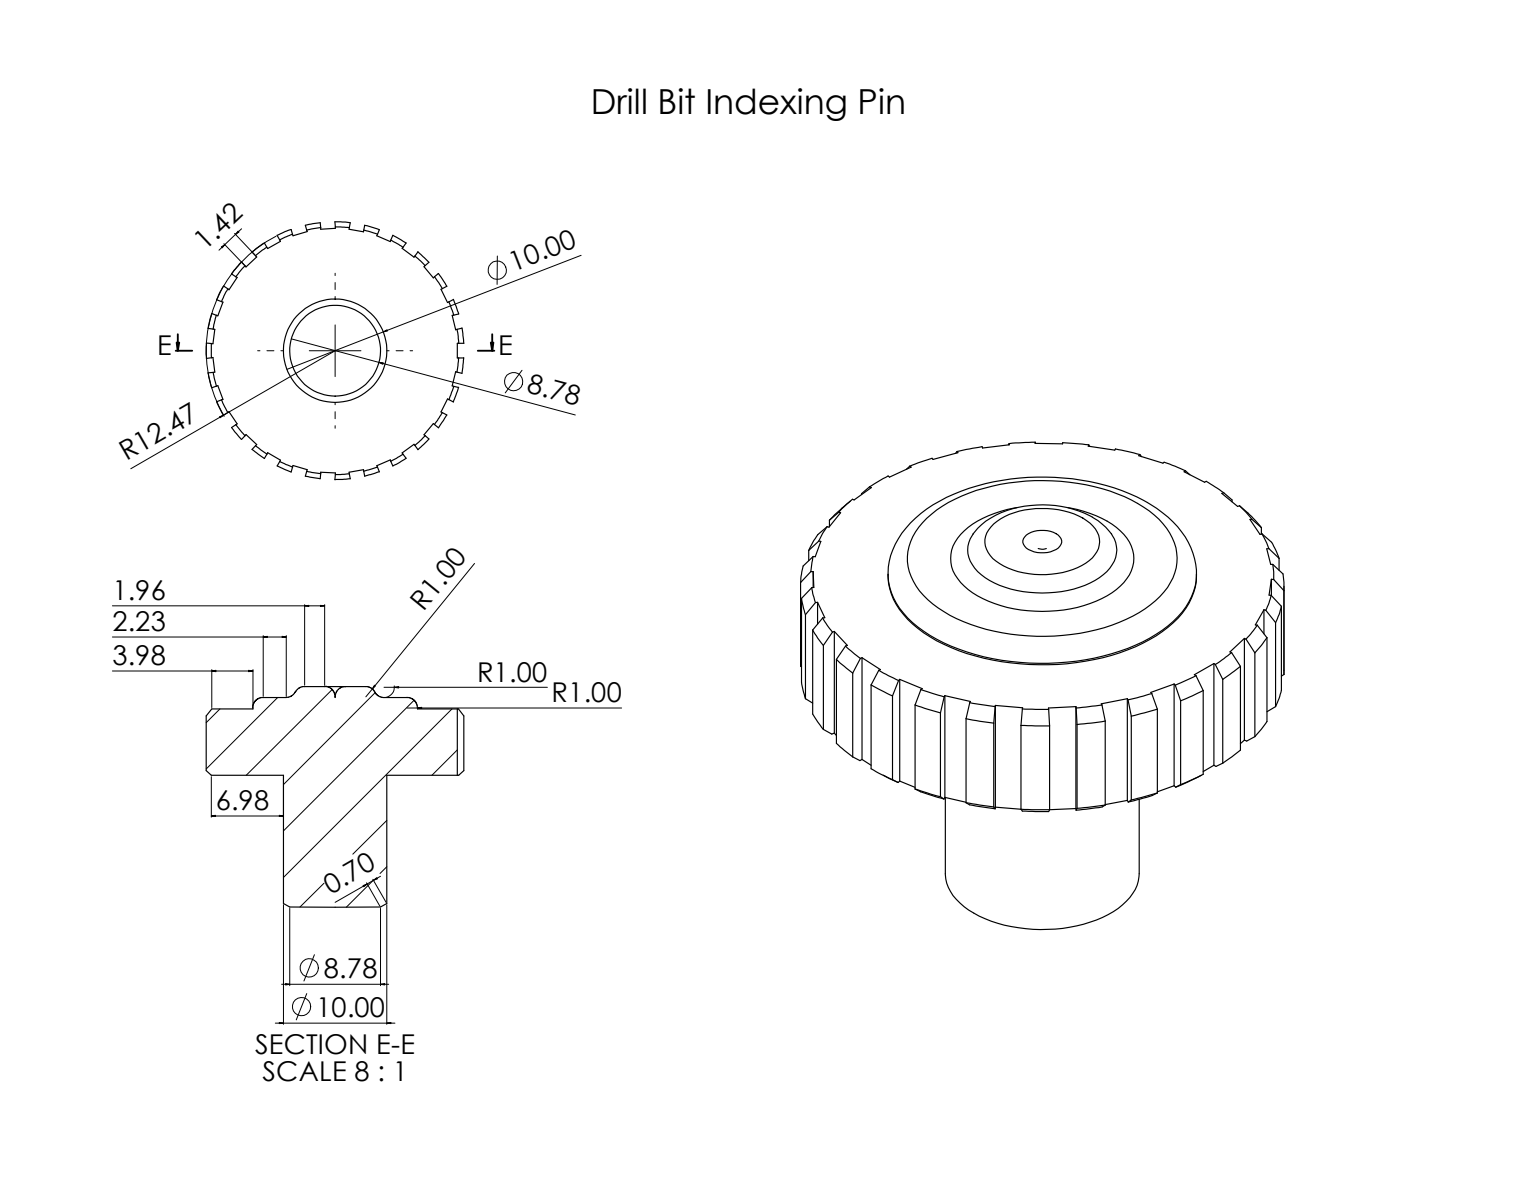
ISO-10303-21;
HEADER;
FILE_DESCRIPTION (('STEP AP214'),
    '1' );
FILE_NAME ('Drill Bit Indexing Pin.step',
    '2026-10-26T22:46:44',
    ( '' ),
    ( '' ),
    'SwSTEP 2.0',
    'SolidWorks 2025',
    '' );
FILE_SCHEMA (( 'AUTOMOTIVE_DESIGN' ));
ENDSEC;

DATA;
#1=PLANE ( 'NONE',  #9182 ) ;
#14=ORIENTED_EDGE ( 'NONE', *, *, #6610, .T. ) ;
#16=DIRECTION ( 'NONE',  ( -0.8660254037844355990, -0.5000000000000055511, 0.000000000000000000 ) ) ;
#17=ORIENTED_EDGE ( 'NONE', *, *, #2123, .F. ) ;
#21=LINE ( 'NONE', #16230, #18993 ) ;
#23=FACE_OUTER_BOUND ( 'NONE', #2829, .T. ) ;
#24=CARTESIAN_POINT ( 'NONE',  ( 211.0853526979653907, 12.80985690719961312, -24.65893733905802776 ) ) ;
#25=AXIS2_PLACEMENT_3D ( 'NONE', #18547, #841, #7289 ) ;
#31=DIRECTION ( 'NONE',  ( -0.2483788854153071712, -0.1434016163555487389, -0.9579895123154875680 ) ) ;
#32=VECTOR ( 'NONE', #7463, 1000.000000000000114 ) ;
#34=LINE ( 'NONE', #11272, #10471 ) ;
#35=CARTESIAN_POINT ( 'NONE',  ( 214.5488276859554162, 7.740514238813806180, -25.36561010639692881 ) ) ;
#39=EDGE_CURVE ( 'NONE', #7899, #11760, #18628, .T. ) ;
#43=B_SPLINE_CURVE_WITH_KNOTS ( 'NONE', 3,
 ( #9463, #2715, #6285, #20719 ),
 .UNSPECIFIED., .F., .F.,
 ( 4, 4 ),
 ( 9.419794497943025677E-05, 0.0009481836829574997018 ),
 .UNSPECIFIED. ) ;
#46=VECTOR ( 'NONE', #10219, 1000.000000000000227 ) ;
#52=LINE ( 'NONE', #20812, #10386 ) ;
#60=ORIENTED_EDGE ( 'NONE', *, *, #4152, .T. ) ;
#63=CARTESIAN_POINT ( 'NONE',  ( 213.9541640218532166, 4.979392293579961937, -14.00000000000005507 ) ) ;
#68=CARTESIAN_POINT ( 'NONE',  ( 204.1847125716027733, 2.529609678273321727, -2.551678190571418092 ) ) ;
#70=CARTESIAN_POINT ( 'NONE',  ( 192.7136026671465174, 6.680946580180795458, -11.01983352639493141 ) ) ;
#77=CARTESIAN_POINT ( 'NONE',  ( 199.2231352798573027, 21.03391272677540513, -14.00000000000005507 ) ) ;
#83=CARTESIAN_POINT ( 'NONE',  ( 215.3534639294407782, 15.62807865697965504, -9.913166705713923221 ) ) ;
#86=ORIENTED_EDGE ( 'NONE', *, *, #18700, .F. ) ;
#89=CARTESIAN_POINT ( 'NONE',  ( 204.5373383384513772, 2.217977392850209561, -25.12838443884007944 ) ) ;
#96=DIRECTION ( 'NONE',  ( 0.7500000000000014433, 0.4330127018922259596, 0.4999999999999919509 ) ) ;
#103=CIRCLE ( 'NONE', #7142, 11.94520687646042667 ) ;
#106=CARTESIAN_POINT ( 'NONE',  ( 199.3420759002524960, 10.50789738563077513, -26.10173121575770239 ) ) ;
#108=CARTESIAN_POINT ( 'NONE',  ( 209.9458835816058411, 16.63000860489531263, -23.47937149798938350 ) ) ;
#109=ADVANCED_FACE ( 'NONE', ( #2310 ), #10446, .F. ) ;
#110=FACE_OUTER_BOUND ( 'NONE', #8894, .T. ) ;
#112=VERTEX_POINT ( 'NONE', #8556 ) ;
#118=EDGE_CURVE ( 'NONE', #7633, #8779, #11849, .T. ) ;
#119=ORIENTED_EDGE ( 'NONE', *, *, #8707, .T. ) ;
#128=DIRECTION ( 'NONE',  ( 0.5000000000000054401, -0.8660254037844354880, 0.000000000000000000 ) ) ;
#131=ORIENTED_EDGE ( 'NONE', *, *, #17184, .F. ) ;
#145=CYLINDRICAL_SURFACE ( 'NONE', #15851, 12.47473710546057646 ) ;
#148=AXIS2_PLACEMENT_3D ( 'NONE', #15807, #6608, #5027 ) ;
#155=ORIENTED_EDGE ( 'NONE', *, *, #17412, .T. ) ;
#157=EDGE_LOOP ( 'NONE', ( #6682, #1571, #19730, #8704 ) ) ;
#159=DIRECTION ( 'NONE',  ( 0.5000000000000054401, -0.8660254037844353769, 3.330669073875469128E-16 ) ) ;
#160=LINE ( 'NONE', #8201, #12763 ) ;
#161=AXIS2_PLACEMENT_3D ( 'NONE', #9354, #1324, #10848 ) ;
#163=CARTESIAN_POINT ( 'NONE',  ( 204.3649803021097568, 2.376073449241438595, -2.709673684914560621 ) ) ;
#171=EDGE_CURVE ( 'NONE', #6173, #11821, #2564, .T. ) ;
#177=VECTOR ( 'NONE', #19876, 1000.000000000000114 ) ;
#178=ORIENTED_EDGE ( 'NONE', *, *, #4682, .F. ) ;
#184=VERTEX_POINT ( 'NONE', #12380 ) ;
#185=ORIENTED_EDGE ( 'NONE', *, *, #2629, .T. ) ;
#186=EDGE_CURVE ( 'NONE', #5696, #10545, #15103, .T. ) ;
#192=ORIENTED_EDGE ( 'NONE', *, *, #8358, .F. ) ;
#194=VECTOR ( 'NONE', #13444, 1000.000000000000000 ) ;
#202=CARTESIAN_POINT ( 'NONE',  ( 206.2111997916997552, 10.34978999605213978, -2.036337243043280676 ) ) ;
#210=EDGE_CURVE ( 'NONE', #4589, #15417, #7306, .T. ) ;
#211=VECTOR ( 'NONE', #12529, 1000.000000000000114 ) ;
#212=CARTESIAN_POINT ( 'NONE',  ( 206.9147384664715048, 10.75597823931694563, -16.91825718831810477 ) ) ;
#224=CIRCLE ( 'NONE', #4614, 1.000000000000000888 ) ;
#230=DIRECTION ( 'NONE',  ( -0.5000000000000049960, 0.8660254037844358210, -0.000000000000000000 ) ) ;
#233=DIRECTION ( 'NONE',  ( -0.8660254037844354880, -0.5000000000000055511, 0.000000000000000000 ) ) ;
#234=ADVANCED_FACE ( 'NONE', ( #2627 ), #13079, .T. ) ;
#242=ORIENTED_EDGE ( 'NONE', *, *, #18363, .T. ) ;
#244=DIRECTION ( 'NONE',  ( -0.5000000000000049960, 0.8660254037844357100, -0.000000000000000000 ) ) ;
#248=CARTESIAN_POINT ( 'NONE',  ( 215.3457899893760725, 15.62364810561754958, -18.11117897393244647 ) ) ;
#251=LINE ( 'NONE', #16684, #18558 ) ;
#255=VERTEX_POINT ( 'NONE', #1143 ) ;
#257=ORIENTED_EDGE ( 'NONE', *, *, #4813, .T. ) ;
#258=CARTESIAN_POINT ( 'NONE',  ( 204.4631859798315361, 9.340573751222835952, -1.438440158918556255 ) ) ;
#260=CARTESIAN_POINT ( 'NONE',  ( 216.5552780741873278, 15.79089711517258188, -12.53629070788368338 ) ) ;
#266=ORIENTED_EDGE ( 'NONE', *, *, #16288, .F. ) ;
#267=VECTOR ( 'NONE', #19215, 1000.000000000000227 ) ;
#271=B_SPLINE_CURVE_WITH_KNOTS ( 'NONE', 3,
 ( #15574, #20319, #4421, #12593 ),
 .UNSPECIFIED., .F., .F.,
 ( 4, 4 ),
 ( 3.854193985297353114E-07, 0.0008543711573825201388 ),
 .UNSPECIFIED. ) ;
#275=LINE ( 'NONE', #15144, #3748 ) ;
#277=EDGE_CURVE ( 'NONE', #4589, #9756, #12406, .T. ) ;
#284=B_SPLINE_CURVE_WITH_KNOTS ( 'NONE', 3,
 ( #15872, #6200, #7896, #7588 ),
 .UNSPECIFIED., .F., .F.,
 ( 4, 4 ),
 ( 5.392423665328082974E-07, 0.0008545249803445767369 ),
 .UNSPECIFIED. ) ;
#286=ORIENTED_EDGE ( 'NONE', *, *, #8772, .T. ) ;
#291=CARTESIAN_POINT ( 'NONE',  ( 213.7304257015346423, 14.51400719500950132, -6.188753603160008332 ) ) ;
#295=EDGE_CURVE ( 'NONE', #10545, #10364, #20522, .T. ) ;
#296=DIRECTION ( 'NONE',  ( 0.5943026915289653100, 0.3431208189343725179, 0.7273736415730454041 ) ) ;
#303=CARTESIAN_POINT ( 'NONE',  ( 205.0644204223817439, 9.510686714291797017, -26.12768996730766347 ) ) ;
#306=ORIENTED_EDGE ( 'NONE', *, *, #3575, .F. ) ;
#307=EDGE_CURVE ( 'NONE', #6314, #7288, #8664, .T. ) ;
#310=VERTEX_POINT ( 'NONE', #12278 ) ;
#315=EDGE_CURVE ( 'NONE', #14969, #8807, #10929, .T. ) ;
#317=CARTESIAN_POINT ( 'NONE',  ( 207.3576251285122112, 11.01167897286662800, -2.341985411377013548 ) ) ;
#320=DIRECTION ( 'NONE',  ( -0.8660254037844355990, -0.5000000000000055511, 0.000000000000000000 ) ) ;
#321=ORIENTED_EDGE ( 'NONE', *, *, #9028, .T. ) ;
#323=CARTESIAN_POINT ( 'NONE',  ( 209.1177676012032407, 5.377710327540435209, -26.45271578590685380 ) ) ;
#325=AXIS2_PLACEMENT_3D ( 'NONE', #1147, #20520, #11965 ) ;
#328=DIRECTION ( 'NONE',  ( 0.9537419254229496657, 0.000000000000000000, 0.3006265784832155008 ) ) ;
#330=VERTEX_POINT ( 'NONE', #3444 ) ;
#335=ORIENTED_EDGE ( 'NONE', *, *, #7992, .F. ) ;
#340=VERTEX_POINT ( 'NONE', #1652 ) ;
#341=LINE ( 'NONE', #19828, #4394 ) ;
#343=EDGE_CURVE ( 'NONE', #18516, #1461, #6859, .T. ) ;
#344=ORIENTED_EDGE ( 'NONE', *, *, #7860, .F. ) ;
#346=VECTOR ( 'NONE', #15320, 1000.000000000000114 ) ;
#356=CARTESIAN_POINT ( 'NONE',  ( 205.5965122587965084, 9.994899983462953941, -14.00000000000005507 ) ) ;
#357=CARTESIAN_POINT ( 'NONE',  ( 218.1364845712607803, 10.58466899794828642, -8.415281845792092597 ) ) ;
#360=ADVANCED_FACE ( 'NONE', ( #16385 ), #15798, .T. ) ;
#367=AXIS2_PLACEMENT_3D ( 'NONE', #16920, #11953, #10334 ) ;
#370=LINE ( 'NONE', #11808, #12203 ) ;
#375=LINE ( 'NONE', #8408, #1415 ) ;
#377=AXIS2_PLACEMENT_3D ( 'NONE', #5841, #2472, #8925 ) ;
#380=DIRECTION ( 'NONE',  ( 0.3430151393149036276, 0.1980398830195791438, -0.9182161068802751069 ) ) ;
#384=FACE_OUTER_BOUND ( 'NONE', #1878, .T. ) ;
#389=DIRECTION ( 'NONE',  ( 0.8660254037844355990, 0.5000000000000054401, 0.000000000000000000 ) ) ;
#392=CARTESIAN_POINT ( 'NONE',  ( 205.8264633344831225, 9.596613037118636669, -14.00000000000005507 ) ) ;
#405=DIRECTION ( 'NONE',  ( 1.000000000000000000, 0.000000000000000000, 0.000000000000000000 ) ) ;
#413=CIRCLE ( 'NONE', #5471, 12.47473710546057823 ) ;
#415=VECTOR ( 'NONE', #6964, 1000.000000000000114 ) ;
#418=DIRECTION ( 'NONE',  ( 0.1005394128318083530, 0.05804645706261224447, -0.9932383577419438003 ) ) ;
#420=CARTESIAN_POINT ( 'NONE',  ( 199.2144802262915846, 21.04890371929339921, -14.00000000000005507 ) ) ;
#421=DIRECTION ( 'NONE',  ( -0.8660254037844355990, -0.5000000000000054401, 9.734124438199387596E-15 ) ) ;
#425=VERTEX_POINT ( 'NONE', #12897 ) ;
#430=VECTOR ( 'NONE', #14086, 1000.000000000000114 ) ;
#437=VERTEX_POINT ( 'NONE', #8202 ) ;
#438=CARTESIAN_POINT ( 'NONE',  ( 212.7108869958215109, 14.10238615300026410, -22.72623880687309139 ) ) ;
#440=DIRECTION ( 'NONE',  ( 0.9679941405060923376, 0.000000000000000000, 0.2509727952306220478 ) ) ;
#441=CARTESIAN_POINT ( 'NONE',  ( 200.5889925535338989, 11.22780505105986748, -1.381056684022586634 ) ) ;
#446=DIRECTION ( 'NONE',  ( 0.8426815769442687065, 0.4865224352899183979, 0.2306158707424263710 ) ) ;
#451=CARTESIAN_POINT ( 'NONE',  ( 218.7787453705537928, 10.18265835266665675, -11.24974199967301836 ) ) ;
#453=EDGE_LOOP ( 'NONE', ( #8064, #10260, #20838, #5288 ) ) ;
#455=EDGE_CURVE ( 'NONE', #2505, #184, #11818, .T. ) ;
#457=AXIS2_PLACEMENT_3D ( 'NONE', #2689, #2291, #9232 ) ;
#467=EDGE_CURVE ( 'NONE', #12472, #14490, #11407, .T. ) ;
#472=AXIS2_PLACEMENT_3D ( 'NONE', #20887, #6361, #6670 ) ;
#473=CARTESIAN_POINT ( 'NONE',  ( 203.1005406747554218, 12.67784803492986434, -27.13030671846408737 ) ) ;
#478=EDGE_CURVE ( 'NONE', #11306, #15921, #11716, .T. ) ;
#479=ORIENTED_EDGE ( 'NONE', *, *, #14298, .T. ) ;
#489=DIRECTION ( 'NONE',  ( 0.8660254037844352659, 0.5000000000000056621, 0.000000000000000000 ) ) ;
#508=ORIENTED_EDGE ( 'NONE', *, *, #8439, .F. ) ;
#514=DIRECTION ( 'NONE',  ( 0.5171545105027486322, 0.2985792958513951434, -0.8021231927550452889 ) ) ;
#515=CARTESIAN_POINT ( 'NONE',  ( 203.4466382902124622, 1.588261426394339981, -3.504773242918958420 ) ) ;
#518=CIRCLE ( 'NONE', #2552, 11.94520687646042667 ) ;
#531=ORIENTED_EDGE ( 'NONE', *, *, #18795, .T. ) ;
#534=DIRECTION ( 'NONE',  ( -0.5000000000000051070, 0.8660254037844359321, -0.000000000000000000 ) ) ;
#536=EDGE_CURVE ( 'NONE', #19458, #4355, #2580, .T. ) ;
#539=CARTESIAN_POINT ( 'NONE',  ( 212.9607779367323417, 18.37065867240589156, -8.669480444820855780 ) ) ;
#543=DIRECTION ( 'NONE',  ( -0.8404609622711977091, 0.000000000000000000, 0.5418720982835085742 ) ) ;
#550=CARTESIAN_POINT ( 'NONE',  ( 207.0013954503587286, 3.383002205901548098, -25.76107385416581508 ) ) ;
#552=B_SPLINE_CURVE_WITH_KNOTS ( 'NONE', 3,
 ( #19683, #19790, #16415, #17907 ),
 .UNSPECIFIED., .F., .F.,
 ( 4, 4 ),
 ( 5.256891072071942815E-05, 0.0007252197027765627845 ),
 .UNSPECIFIED. ) ;
#556=ORIENTED_EDGE ( 'NONE', *, *, #2526, .F. ) ;
#561=EDGE_CURVE ( 'NONE', #18877, #3166, #9046, .T. ) ;
#562=VECTOR ( 'NONE', #12012, 1000.000000000000000 ) ;
#567=DIRECTION ( 'NONE',  ( -0.8660254037844355990, -0.5000000000000054401, 9.734124438199387596E-15 ) ) ;
#568=FACE_OUTER_BOUND ( 'NONE', #8960, .T. ) ;
#574=CARTESIAN_POINT ( 'NONE',  ( 205.7612434495831621, 0.2492073957305620258, -14.00000000000005507 ) ) ;
#579=ORIENTED_EDGE ( 'NONE', *, *, #17154, .T. ) ;
#581=DIRECTION ( 'NONE',  ( -0.5000000000000051070, 0.8660254037844359321, -0.000000000000000000 ) ) ;
#582=CARTESIAN_POINT ( 'NONE',  ( 199.2144802262915846, 21.04890371929339921, -14.00000000000005507 ) ) ;
#589=EDGE_CURVE ( 'NONE', #17484, #14639, #4503, .T. ) ;
#590=FACE_OUTER_BOUND ( 'NONE', #6120, .T. ) ;
#593=ADVANCED_FACE ( 'NONE', ( #20489 ), #18839, .T. ) ;
#599=CARTESIAN_POINT ( 'NONE',  ( 209.9028093415542457, 12.48114176340366122, -13.84394651341481008 ) ) ;
#600=VERTEX_POINT ( 'NONE', #20184 ) ;
#605=ADVANCED_FACE ( 'NONE', ( #2494 ), #17328, .F. ) ;
#606=ORIENTED_EDGE ( 'NONE', *, *, #5768, .T. ) ;
#610=DIRECTION ( 'NONE',  ( 0.5000000000000049960, -0.8660254037844358210, 0.000000000000000000 ) ) ;
#613=VECTOR ( 'NONE', #5948, 1000.000000000000114 ) ;
#620=CARTESIAN_POINT ( 'NONE',  ( 200.2585560139914378, -0.5099779577875940273, -20.52105855319921801 ) ) ;
#622=CARTESIAN_POINT ( 'NONE',  ( 199.5722073119862046, -0.9062415656482646353, -8.625373497621064089 ) ) ;
#629=EDGE_CURVE ( 'NONE', #9080, #19592, #13093, .T. ) ;
#630=EDGE_LOOP ( 'NONE', ( #1633, #10180, #13625, #15445 ) ) ;
#633=DIRECTION ( 'NONE',  ( 0.8645602258681710506, 0.4991540791356393614, -0.05814482891047953461 ) ) ;
#635=ORIENTED_EDGE ( 'NONE', *, *, #10307, .F. ) ;
#637=ORIENTED_EDGE ( 'NONE', *, *, #186, .T. ) ;
#642=DIRECTION ( 'NONE',  ( -0.7951984747223626027, -0.4591080534401425495, -0.3960797660391542907 ) ) ;
#644=LINE ( 'NONE', #6991, #11943 ) ;
#648=DIRECTION ( 'NONE',  ( -0.8660254037844354880, -0.5000000000000055511, 0.000000000000000000 ) ) ;
#649=VECTOR ( 'NONE', #3501, 1000.000000000000227 ) ;
#650=ORIENTED_EDGE ( 'NONE', *, *, #14383, .T. ) ;
#652=EDGE_CURVE ( 'NONE', #15437, #9266, #15812, .T. ) ;
#654=CARTESIAN_POINT ( 'NONE',  ( 198.4658173668363190, 5.877991368080599521, -5.291540431471293715 ) ) ;
#667=FACE_OUTER_BOUND ( 'NONE', #13989, .T. ) ;
#668=AXIS2_PLACEMENT_3D ( 'NONE', #6471, #18619, #19618 ) ;
#671=EDGE_LOOP ( 'NONE', ( #12795, #14132, #9579, #15722 ) ) ;
#683=DIRECTION ( 'NONE',  ( -0.8660254037844360431, -0.5000000000000046629, 0.000000000000000000 ) ) ;
#684=DIRECTION ( 'NONE',  ( -0.5000000000000049960, 0.8660254037844357100, -0.000000000000000000 ) ) ;
#688=VERTEX_POINT ( 'NONE', #7875 ) ;
#689=AXIS2_PLACEMENT_3D ( 'NONE', #12223, #19001, #18689 ) ;
#691=VECTOR ( 'NONE', #8828, 1000.000000000000114 ) ;
#694=VERTEX_POINT ( 'NONE', #14476 ) ;
#695=LINE ( 'NONE', #805, #4095 ) ;
#696=CARTESIAN_POINT ( 'NONE',  ( 197.9607918626003311, -1.063772618484184918, -11.13829696442576811 ) ) ;
#697=AXIS2_PLACEMENT_3D ( 'NONE', #2673, #767, #5401 ) ;
#698=CARTESIAN_POINT ( 'NONE',  ( 202.6752174627569332, 8.308289646587223132, -25.34310559273323449 ) ) ;
#700=DIRECTION ( 'NONE',  ( -0.8660254037844355990, -0.5000000000000055511, 0.000000000000000000 ) ) ;
#703=ORIENTED_EDGE ( 'NONE', *, *, #15898, .T. ) ;
#704=ORIENTED_EDGE ( 'NONE', *, *, #7277, .F. ) ;
#706=ORIENTED_EDGE ( 'NONE', *, *, #17795, .T. ) ;
#707=LINE ( 'NONE', #18409, #13248 ) ;
#708=DIRECTION ( 'NONE',  ( 0.9367698044638429478, 0.000000000000000000, 0.3499461864984006465 ) ) ;
#712=ORIENTED_EDGE ( 'NONE', *, *, #4751, .F. ) ;
#717=ORIENTED_EDGE ( 'NONE', *, *, #18489, .F. ) ;
#727=CARTESIAN_POINT ( 'NONE',  ( 209.3139125749813445, 4.975733814115070430, -1.899081834577973860 ) ) ;
#728=AXIS2_PLACEMENT_3D ( 'NONE', #13100, #4823, #8301 ) ;
#736=ORIENTED_EDGE ( 'NONE', *, *, #2296, .F. ) ;
#743=VECTOR ( 'NONE', #7557, 1000.000000000000227 ) ;
#744=EDGE_CURVE ( 'NONE', #6868, #9199, #6180, .T. ) ;
#746=ORIENTED_EDGE ( 'NONE', *, *, #6799, .T. ) ;
#751=VECTOR ( 'NONE', #3852, 1000.000000000000227 ) ;
#754=ADVANCED_FACE ( 'NONE', ( #1529, #19230 ), #4696, .F. ) ;
#756=CARTESIAN_POINT ( 'NONE',  ( 208.8107687779841228, 4.427644383670616079, -14.00000000000005507 ) ) ;
#759=CARTESIAN_POINT ( 'NONE',  ( 215.9194406937061217, 8.531838027793467560, -5.321846656828220112 ) ) ;
#764=VECTOR ( 'NONE', #5969, 1000.000000000000114 ) ;
#767=DIRECTION ( 'NONE',  ( 0.5000000000000054401, -0.8660254037844354880, 0.000000000000000000 ) ) ;
#768=CARTESIAN_POINT ( 'NONE',  ( 203.1960812450809897, 12.73300840892584063, -0.8632678296711639998 ) ) ;
#772=VERTEX_POINT ( 'NONE', #13385 ) ;
#777=CARTESIAN_POINT ( 'NONE',  ( 199.3993387870319509, 20.72871929987707063, -14.00000000000005507 ) ) ;
#781=CARTESIAN_POINT ( 'NONE',  ( 199.2144802262915846, 21.04890371929339921, -14.00000000000005507 ) ) ;
#782=CARTESIAN_POINT ( 'NONE',  ( 205.8264633344831225, 9.596613037118636669, -14.00000000000005507 ) ) ;
#786=DIRECTION ( 'NONE',  ( 0.5000000000000051070, -0.8660254037844359321, 0.000000000000000000 ) ) ;
#791=VERTEX_POINT ( 'NONE', #15207 ) ;
#792=ORIENTED_EDGE ( 'NONE', *, *, #10046, .T. ) ;
#797=FACE_OUTER_BOUND ( 'NONE', #8862, .T. ) ;
#798=ORIENTED_EDGE ( 'NONE', *, *, #10136, .F. ) ;
#799=EDGE_CURVE ( 'NONE', #310, #13335, #18256, .T. ) ;
#802=LINE ( 'NONE', #2502, #12393 ) ;
#803=VECTOR ( 'NONE', #16193, 1000.000000000000227 ) ;
#805=CARTESIAN_POINT ( 'NONE',  ( 189.5541235174889607, 15.47149417299831420, -8.415281845791808379 ) ) ;
#806=CARTESIAN_POINT ( 'NONE',  ( 198.4854721009812124, -1.276069208452816683, -11.19970074074890398 ) ) ;
#809=CARTESIAN_POINT ( 'NONE',  ( 200.9478142713745967, -0.1120345173462600208, -21.59012016402711609 ) ) ;
#811=EDGE_LOOP ( 'NONE', ( #7188, #13971, #15070, #13697 ) ) ;
#812=CARTESIAN_POINT ( 'NONE',  ( 201.7213150758130382, 0.3345463803147161741, -22.69908973750332848 ) ) ;
#821=DIRECTION ( 'NONE',  ( -0.8660254037844355990, -0.5000000000000054401, 1.154189040529355901E-14 ) ) ;
#834=ORIENTED_EDGE ( 'NONE', *, *, #12337, .F. ) ;
#835=VERTEX_POINT ( 'NONE', #6798 ) ;
#836=ORIENTED_EDGE ( 'NONE', *, *, #13762, .F. ) ;
#841=DIRECTION ( 'NONE',  ( -0.5000000000000049960, 0.8660254037844357100, -0.000000000000000000 ) ) ;
#844=VERTEX_POINT ( 'NONE', #8603 ) ;
#846=LINE ( 'NONE', #13785, #16170 ) ;
#852=ORIENTED_EDGE ( 'NONE', *, *, #12815, .T. ) ;
#855=CARTESIAN_POINT ( 'NONE',  ( 213.9946316566572193, 7.420549012114688203, -3.662783021451589960 ) ) ;
#858=DIRECTION ( 'NONE',  ( 0.1997192025788214198, 0.1153079353712215815, 0.9730448705798235842 ) ) ;
#859=CARTESIAN_POINT ( 'NONE',  ( 206.8262688097345574, 1.942051447093357419, -14.00000000000005507 ) ) ;
#860=CARTESIAN_POINT ( 'NONE',  ( 207.0179943350029248, 10.81559304280895262, -12.31324071153516364 ) ) ;
#864=VECTOR ( 'NONE', #2674, 1000.000000000000114 ) ;
#866=DIRECTION ( 'NONE',  ( 0.5000000000000052180, -0.8660254037844355990, 8.326672684688672821E-17 ) ) ;
#870=LINE ( 'NONE', #1189, #10969 ) ;
#872=DIRECTION ( 'NONE',  ( -0.8660254037844355990, -0.5000000000000055511, 0.000000000000000000 ) ) ;
#878=CARTESIAN_POINT ( 'NONE',  ( 202.7409362990318584, 7.815183172608958451, -2.044871543906938705 ) ) ;
#879=AXIS2_PLACEMENT_3D ( 'NONE', #8903, #12316, #5705 ) ;
#880=ADVANCED_FACE ( 'NONE', ( #19627 ), #12422, .T. ) ;
#882=ADVANCED_FACE ( 'NONE', ( #16671 ), #18054, .F. ) ;
#887=ADVANCED_FACE ( 'NONE', ( #5202 ), #10073, .F. ) ;
#893=EDGE_LOOP ( 'NONE', ( #12615, #1786 ) ) ;
#896=CIRCLE ( 'NONE', #4616, 12.47473710546057823 ) ;
#901=ORIENTED_EDGE ( 'NONE', *, *, #17043, .F. ) ;
#902=LINE ( 'NONE', #18920, #12017 ) ;
#904=DIRECTION ( 'NONE',  ( -0.5000000000000054401, 0.8660254037844354880, -0.000000000000000000 ) ) ;
#905=CARTESIAN_POINT ( 'NONE',  ( 205.0662616026534693, 10.91332106064940888, -14.00000000000005507 ) ) ;
#908=CARTESIAN_POINT ( 'NONE',  ( 209.6893306017077805, 12.35788975548704016, -15.55404723004300926 ) ) ;
#910=CARTESIAN_POINT ( 'NONE',  ( 199.2144802262915846, 21.04890371929339921, -14.00000000000005507 ) ) ;
#915=CARTESIAN_POINT ( 'NONE',  ( 211.7316270624183403, 13.53701016684330405, -23.47937149798937995 ) ) ;
#920=CARTESIAN_POINT ( 'NONE',  ( 205.8264633344831225, 9.596613037118636669, -14.00000000000005507 ) ) ;
#925=DIRECTION ( 'NONE',  ( -0.5000000000000054401, 0.8660254037844354880, -0.000000000000000000 ) ) ;
#928=EDGE_LOOP ( 'NONE', ( #19595, #19195, #3468, #19468 ) ) ;
#934=DIRECTION ( 'NONE',  ( -0.8660254037844354880, -0.5000000000000055511, 0.000000000000000000 ) ) ;
#937=ORIENTED_EDGE ( 'NONE', *, *, #14366, .F. ) ;
#940=DIRECTION ( 'NONE',  ( -0.8660254037844355990, -0.5000000000000054401, 1.237624392856779246E-14 ) ) ;
#945=EDGE_CURVE ( 'NONE', #3585, #11939, #6044, .T. ) ;
#958=VECTOR ( 'NONE', #7619, 999.9999999999998863 ) ;
#963=DIRECTION ( 'NONE',  ( 0.3430151393149145633, 0.1980398830195858606, 0.9182161068802694448 ) ) ;
#971=ORIENTED_EDGE ( 'NONE', *, *, #18549, .T. ) ;
#972=DIRECTION ( 'NONE',  ( 0.8296432542242784258, 0.4789947561577511115, 0.2868032327110801583 ) ) ;
#976=CARTESIAN_POINT ( 'NONE',  ( 213.4594667654058924, 14.53457888447970170, -21.59012016402729728 ) ) ;
#977=EDGE_CURVE ( 'NONE', #9718, #6001, #15416, .T. ) ;
#982=CYLINDRICAL_SURFACE ( 'NONE', #9493, 12.47473710546057646 ) ;
#984=CARTESIAN_POINT ( 'NONE',  ( 202.6090205221545943, 8.270070825110927615, -2.522505859538386908 ) ) ;
#985=ADVANCED_FACE ( 'NONE', ( #17194 ), #18683, .F. ) ;
#987=CARTESIAN_POINT ( 'NONE',  ( 219.2382532868116982, 10.96316161069002426, -14.00530714776927255 ) ) ;
#995=CARTESIAN_POINT ( 'NONE',  ( 202.7409362990318584, 7.815183172608958451, -2.044871543906938705 ) ) ;
#998=ORIENTED_EDGE ( 'NONE', *, *, #19233, .T. ) ;
#1000=VERTEX_POINT ( 'NONE', #976 ) ;
#1004=ORIENTED_EDGE ( 'NONE', *, *, #4187, .F. ) ;
#1006=EDGE_CURVE ( 'NONE', #18042, #12264, #12108, .T. ) ;
#1008=EDGE_CURVE ( 'NONE', #18502, #19425, #870, .T. ) ;
#1010=DIRECTION ( 'NONE',  ( 0.8660254037844355990, 0.5000000000000054401, 0.000000000000000000 ) ) ;
#1015=DIRECTION ( 'NONE',  ( -0.5000000000000049960, 0.8660254037844357100, -0.000000000000000000 ) ) ;
#1016=AXIS2_PLACEMENT_3D ( 'NONE', #910, #16815, #20500 ) ;
#1021=ORIENTED_EDGE ( 'NONE', *, *, #945, .F. ) ;
#1023=CARTESIAN_POINT ( 'NONE',  ( 198.8427921854145666, -1.327369585325435697, -11.24974199967268618 ) ) ;
#1025=ORIENTED_EDGE ( 'NONE', *, *, #12215, .T. ) ;
#1028=CARTESIAN_POINT ( 'NONE',  ( 197.6529114527598381, 5.408659919762685675, -6.286464976498783663 ) ) ;
#1029=CARTESIAN_POINT ( 'NONE',  ( 205.0662616026534693, 10.91332106064940888, -14.00000000000005507 ) ) ;
#1030=DIRECTION ( 'NONE',  ( -0.5000000000000053291, 0.8660254037844354880, 0.000000000000000000 ) ) ;
#1033=ORIENTED_EDGE ( 'NONE', *, *, #8767, .F. ) ;
#1036=AXIS2_PLACEMENT_3D ( 'NONE', #3801, #18758, #2222 ) ;
#1045=ORIENTED_EDGE ( 'NONE', *, *, #1095, .T. ) ;
#1046=AXIS2_PLACEMENT_3D ( 'NONE', #11317, #4843, #17688 ) ;
#1047=LINE ( 'NONE', #7499, #3075 ) ;
#1048=CARTESIAN_POINT ( 'NONE',  ( 213.0626749079333422, 13.95146441739924725, -5.040853264743544671 ) ) ;
#1049=CARTESIAN_POINT ( 'NONE',  ( 212.7675431533135679, 7.484909225033065994, -2.551678190571531335 ) ) ;
#1051=VERTEX_POINT ( 'NONE', #1087 ) ;
#1053=VERTEX_POINT ( 'NONE', #2782 ) ;
#1055=DIRECTION ( 'NONE',  ( 0.8660254037844355990, 0.5000000000000054401, 4.449885457462577074E-15 ) ) ;
#1059=ORIENTED_EDGE ( 'NONE', *, *, #1720, .F. ) ;
#1060=EDGE_CURVE ( 'NONE', #14979, #11827, #7535, .T. ) ;
#1061=DIRECTION ( 'NONE',  ( 0.5000000000000055511, -0.8660254037844353769, 2.220446049250313574E-16 ) ) ;
#1063=CARTESIAN_POINT ( 'NONE',  ( 209.7467543128910563, 12.39104335059656670, -14.69381062500531954 ) ) ;
#1068=EDGE_CURVE ( 'NONE', #5521, #2903, #5936, .T. ) ;
#1073=CARTESIAN_POINT ( 'NONE',  ( 215.9063259570648654, 8.781865454870326104, -5.186396688528637000 ) ) ;
#1082=CARTESIAN_POINT ( 'NONE',  ( 210.7420593526228458, 5.542675516821637949, -26.96550585544247269 ) ) ;
#1085=VECTOR ( 'NONE', #6641, 1000.000000000000000 ) ;
#1087=CARTESIAN_POINT ( 'NONE',  ( 202.7150726112346319, 7.800250765496993033, -25.94618751764486575 ) ) ;
#1092=CARTESIAN_POINT ( 'NONE',  ( 202.0355941508142337, 1.288815579510670828, -24.01557619556968248 ) ) ;
#1095=EDGE_CURVE ( 'NONE', #9963, #11917, #13002, .T. ) ;
#1096=DIRECTION ( 'NONE',  ( 0.8660254037844358210, 0.5000000000000049960, 0.000000000000000000 ) ) ;
#1099=VECTOR ( 'NONE', #8346, 1000.000000000000114 ) ;
#1100=CARTESIAN_POINT ( 'NONE',  ( 203.0861028855985069, 1.895327080324426428, -3.188775577416750995 ) ) ;
#1101=CARTESIAN_POINT ( 'NONE',  ( 210.8574505745143028, 17.15630205363537186, -5.407152407594056243 ) ) ;
#1103=ORIENTED_EDGE ( 'NONE', *, *, #15143, .T. ) ;
#1104=DIRECTION ( 'NONE',  ( 0.8660254037844352659, 0.5000000000000056621, 0.000000000000000000 ) ) ;
#1110=ORIENTED_EDGE ( 'NONE', *, *, #3916, .F. ) ;
#1112=ORIENTED_EDGE ( 'NONE', *, *, #18437, .T. ) ;
#1122=CARTESIAN_POINT ( 'NONE',  ( 198.4659246047362444, -1.544954184478863901, -13.98474561060102772 ) ) ;
#1125=CARTESIAN_POINT ( 'NONE',  ( 214.8665333410018263, 15.34694915066777909, -8.609703802792745719 ) ) ;
#1133=ORIENTED_EDGE ( 'NONE', *, *, #18363, .F. ) ;
#1136=CARTESIAN_POINT ( 'NONE',  ( 218.3033847652179702, 9.908208779213840245, -6.724618537539639007 ) ) ;
#1143=CARTESIAN_POINT ( 'NONE',  ( 198.3196067457501783, -0.8566107491083605474, -18.25196083293855409 ) ) ;
#1144=PLANE ( 'NONE',  #16507 ) ;
#1145=TOROIDAL_SURFACE ( 'NONE', #16388, 2.961423854602172501, 1.000000000000000000 ) ;
#1147=CARTESIAN_POINT ( 'NONE',  ( 213.7787453705537075, 18.84291239051101741, -11.24974199967302013 ) ) ;
#1149=LINE ( 'NONE', #9488, #430 ) ;
#1151=LINE ( 'NONE', #3896, #18721 ) ;
#1152=CARTESIAN_POINT ( 'NONE',  ( 199.9308801844630636, -0.4415624623656884684, -20.66514661561410549 ) ) ;
#1158=AXIS2_PLACEMENT_3D ( 'NONE', #16759, #2241, #2346 ) ;
#1162=ORIENTED_EDGE ( 'NONE', *, *, #18700, .T. ) ;
#1163=CARTESIAN_POINT ( 'NONE',  ( 205.3647371392095806, 3.210897180031505371, -25.94618751764486575 ) ) ;
#1164=LINE ( 'NONE', #1470, #8820 ) ;
#1167=ORIENTED_EDGE ( 'NONE', *, *, #13583, .F. ) ;
#1168=ORIENTED_EDGE ( 'NONE', *, *, #10911, .T. ) ;
#1171=CARTESIAN_POINT ( 'NONE',  ( 204.2095024616932051, 2.543922127990230209, -25.46066938576250038 ) ) ;
#1174=CARTESIAN_POINT ( 'NONE',  ( 212.1209189702634035, 13.40774137327457360, -4.128377653168339378 ) ) ;
#1176=CARTESIAN_POINT ( 'NONE',  ( 199.1867014016590076, -1.128813506749884343, -18.06789442459577799 ) ) ;
#1177=CARTESIAN_POINT ( 'NONE',  ( 213.9518117939439890, 7.653426176657557534, -3.504773242919091647 ) ) ;
#1181=ORIENTED_EDGE ( 'NONE', *, *, #20493, .T. ) ;
#1184=EDGE_LOOP ( 'NONE', ( #11879, #20337, #17758, #4615, #18514, #9160 ) ) ;
#1186=CARTESIAN_POINT ( 'NONE',  ( 214.4659469037960662, 7.692662996923436580, -2.579136038830254218 ) ) ;
#1187=EDGE_CURVE ( 'NONE', #10193, #12707, #6084, .T. ) ;
#1189=CARTESIAN_POINT ( 'NONE',  ( 210.8363079006330452, 5.597089941386081513, -1.053683606938506045 ) ) ;
#1190=VERTEX_POINT ( 'NONE', #6246 ) ;
#1194=DIRECTION ( 'NONE',  ( 0.5000000000000057732, -0.8660254037844352659, 4.857225732735059864E-17 ) ) ;
#1197=CARTESIAN_POINT ( 'NONE',  ( 206.2111997916997552, 10.34978999605213978, -2.036337243043280676 ) ) ;
#1204=FACE_OUTER_BOUND ( 'NONE', #16741, .T. ) ;
#1206=APPLICATION_CONTEXT ( 'automotive_design' ) ;
#1209=ORIENTED_EDGE ( 'NONE', *, *, #20082, .F. ) ;
#1223=CARTESIAN_POINT ( 'NONE',  ( 205.5965122587965084, 9.994899983462953941, -14.00000000000005507 ) ) ;
#1226=LINE ( 'NONE', #7675, #19537 ) ;
#1228=CARTESIAN_POINT ( 'NONE',  ( 203.7831613941889088, 8.947961373646505123, -25.80036831778739881 ) ) ;
#1235=ORIENTED_EDGE ( 'NONE', *, *, #18795, .F. ) ;
#1238=DIRECTION ( 'NONE',  ( 0.5000000000000051070, -0.8660254037844359321, 0.000000000000000000 ) ) ;
#1241=CARTESIAN_POINT ( 'NONE',  ( 209.9776323673034426, 12.17031427610509908, -2.697891510991576869 ) ) ;
#1244=AXIS2_PLACEMENT_3D ( 'NONE', #5646, #18600, #13730 ) ;
#1246=EDGE_CURVE ( 'NONE', #6296, #7157, #7592, .T. ) ;
#1248=CARTESIAN_POINT ( 'NONE',  ( 196.9311089575304266, 4.991927054840251010, -20.59651891138145174 ) ) ;
#1249=CARTESIAN_POINT ( 'NONE',  ( 210.7957517463719057, 12.99668230119596934, -3.627429155984617459 ) ) ;
#1252=EDGE_CURVE ( 'NONE', #8980, #17374, #4189, .T. ) ;
#1256=ORIENTED_EDGE ( 'NONE', *, *, #17820, .F. ) ;
#1261=ORIENTED_EDGE ( 'NONE', *, *, #6861, .T. ) ;
#1262=AXIS2_PLACEMENT_3D ( 'NONE', #9740, #1916, #8362 ) ;
#1264=AXIS2_PLACEMENT_3D ( 'NONE', #6030, #17709, #18980 ) ;
#1274=DIRECTION ( 'NONE',  ( 0.000000000000000000, 0.000000000000000000, 1.000000000000000000 ) ) ;
#1275=DIRECTION ( 'NONE',  ( 0.8660254037844369313, 0.5000000000000027756, 0.000000000000000000 ) ) ;
#1276=EDGE_CURVE ( 'NONE', #12454, #9370, #18344, .T. ) ;
#1279=CIRCLE ( 'NONE', #13122, 12.47473710546057823 ) ;
#1284=AXIS2_PLACEMENT_3D ( 'NONE', #20720, #9259, #6188 ) ;
#1298=ORIENTED_EDGE ( 'NONE', *, *, #15859, .T. ) ;
#1302=FACE_OUTER_BOUND ( 'NONE', #1876, .T. ) ;
#1304=DIRECTION ( 'NONE',  ( 0.8660254037844352659, 0.5000000000000056621, 0.000000000000000000 ) ) ;
#1306=EDGE_CURVE ( 'NONE', #694, #5859, #19492, .T. ) ;
#1308=ORIENTED_EDGE ( 'NONE', *, *, #2161, .F. ) ;
#1312=LINE ( 'NONE', #10835, #6469 ) ;
#1313=DIRECTION ( 'NONE',  ( 0.5000000000000055511, -0.8660254037844353769, -3.885780586188047891E-16 ) ) ;
#1314=ORIENTED_EDGE ( 'NONE', *, *, #8642, .T. ) ;
#1315=ORIENTED_EDGE ( 'NONE', *, *, #3282, .F. ) ;
#1316=ORIENTED_EDGE ( 'NONE', *, *, #3981, .F. ) ;
#1317=LINE ( 'NONE', #10841, #8842 ) ;
#1324=DIRECTION ( 'NONE',  ( 0.1997192025788090408, 0.1153079353712143929, -0.9730448705798271369 ) ) ;
#1329=DIRECTION ( 'NONE',  ( -0.8137976813493730255, -0.4698463103929600426, -0.3420201433256623291 ) ) ;
#1330=EDGE_CURVE ( 'NONE', #7157, #3143, #8364, .T. ) ;
#1337=VERTEX_POINT ( 'NONE', #16647 ) ;
#1338=ORIENTED_EDGE ( 'NONE', *, *, #16161, .T. ) ;
#1340=LINE ( 'NONE', #16082, #15648 ) ;
#1342=B_SPLINE_CURVE_WITH_KNOTS ( 'NONE', 3,
 ( #15658, #12259, #12363, #1125 ),
 .UNSPECIFIED., .F., .F.,
 ( 4, 4 ),
 ( 6.919709117056541925E-07, 0.0006733427629548835750 ),
 .UNSPECIFIED. ) ;
#1347=CARTESIAN_POINT ( 'NONE',  ( 215.7735982840993927, 15.87064333973761343, -15.39542905462748656 ) ) ;
#1348=ADVANCED_FACE ( 'NONE', ( #8581 ), #10797, .F. ) ;
#1349=CONICAL_SURFACE ( 'NONE', #17952, 38.65920715899539317, 0.03863996524032856789 ) ;
#1350=EDGE_CURVE ( 'NONE', #14490, #14969, #12086, .T. ) ;
#1355=FACE_OUTER_BOUND ( 'NONE', #13439, .T. ) ;
#1359=CARTESIAN_POINT ( 'NONE',  ( 212.7272071507568967, 14.11180859884542649, -5.291540431471497996 ) ) ;
#1360=( NAMED_UNIT ( * ) SI_UNIT ( $, .STERADIAN. ) SOLID_ANGLE_UNIT ( ) );
#1361=ORIENTED_EDGE ( 'NONE', *, *, #4420, .F. ) ;
#1371=ORIENTED_EDGE ( 'NONE', *, *, #1850, .F. ) ;
#1377=DIRECTION ( 'NONE',  ( -0.5000000000000049960, 0.8660254037844358210, -0.000000000000000000 ) ) ;
#1378=CARTESIAN_POINT ( 'NONE',  ( 207.8614403295549380, 4.652369439064019119, -1.545471579934808215 ) ) ;
#1384=CARTESIAN_POINT ( 'NONE',  ( 208.4761278624580711, 5.007259451653140125, -14.00000000000005507 ) ) ;
#1386=EDGE_LOOP ( 'NONE', ( #16247, #3887, #7387, #1033, #8752, #6624 ) ) ;
#1390=ORIENTED_EDGE ( 'NONE', *, *, #8484, .T. ) ;
#1399=AXIS2_PLACEMENT_3D ( 'NONE', #17157, #2641, #9082 ) ;
#1405=DIRECTION ( 'NONE',  ( -0.8660254037844357100, -0.5000000000000051070, 0.000000000000000000 ) ) ;
#1406=AXIS2_PLACEMENT_3D ( 'NONE', #3019, #7571, #20811 ) ;
#1408=CARTESIAN_POINT ( 'NONE',  ( 210.9308365141136790, 12.89766362403163491, -24.52223341984404570 ) ) ;
#1410=VECTOR ( 'NONE', #159, 1000.000000000000114 ) ;
#1411=LINE ( 'NONE', #20788, #14012 ) ;
#1414=ORIENTED_EDGE ( 'NONE', *, *, #5727, .F. ) ;
#1415=VECTOR ( 'NONE', #11712, 1000.000000000000227 ) ;
#1423=EDGE_LOOP ( 'NONE', ( #15729, #19961, #20861, #4129, #20202, #13171, #20531 ) ) ;
#1433=VERTEX_POINT ( 'NONE', #20449 ) ;
#1439=LINE ( 'NONE', #15662, #5742 ) ;
#1447=DIRECTION ( 'NONE',  ( 1.000000000000000000, 0.000000000000000000, 0.000000000000000000 ) ) ;
#1452=ORIENTED_EDGE ( 'NONE', *, *, #6302, .F. ) ;
#1453=CARTESIAN_POINT ( 'NONE',  ( 212.2669970461267042, 13.31505690926096364, -24.01557619556987788 ) ) ;
#1461=VERTEX_POINT ( 'NONE', #18446 ) ;
#1468=ORIENTED_EDGE ( 'NONE', *, *, #11042, .F. ) ;
#1470=CARTESIAN_POINT ( 'NONE',  ( 214.4667135392577961, 16.34067451675213434, -14.00000000000005507 ) ) ;
#1471=CARTESIAN_POINT ( 'NONE',  ( 216.2725394319739110, 15.91768827161142674, -14.00000000000005507 ) ) ;
#1475=VERTEX_POINT ( 'NONE', #8898 ) ;
#1480=B_SPLINE_CURVE_WITH_KNOTS ( 'NONE', 3,
 ( #878, #2892, #18792, #984 ),
 .UNSPECIFIED., .F., .F.,
 ( 4, 4 ),
 ( 2.816680711908978775E-07, 0.0006729324601288649149 ),
 .UNSPECIFIED. ) ;
#1489=ORIENTED_EDGE ( 'NONE', *, *, #12667, .F. ) ;
#1491=ADVANCED_FACE ( 'NONE', ( #7399 ), #9603, .T. ) ;
#1493=ORIENTED_EDGE ( 'NONE', *, *, #2131, .F. ) ;
#1495=CARTESIAN_POINT ( 'NONE',  ( 209.3577481411912231, 3.480248335904264856, -14.00000000000005507 ) ) ;
#1498=ORIENTED_EDGE ( 'NONE', *, *, #7269, .T. ) ;
#1502=CARTESIAN_POINT ( 'NONE',  ( 194.1867014016589508, 7.531440531094472313, -18.06789442459577444 ) ) ;
#1506=ADVANCED_FACE ( 'NONE', ( #17384 ), #8308, .F. ) ;
#1508=DIRECTION ( 'NONE',  ( -0.5000000000000049960, 0.8660254037844357100, -0.000000000000000000 ) ) ;
#1511=LINE ( 'NONE', #3303, #4175 ) ;
#1513=CARTESIAN_POINT ( 'NONE',  ( 202.6305150283801026, 8.282480684066333865, -25.48492467622465441 ) ) ;
#1517=EDGE_CURVE ( 'NONE', #1689, #7288, #16483, .T. ) ;
#1522=VERTEX_POINT ( 'NONE', #20650 ) ;
#1524=ORIENTED_EDGE ( 'NONE', *, *, #171, .T. ) ;
#1529=FACE_BOUND ( 'NONE', #1543, .T. ) ;
#1532=CARTESIAN_POINT ( 'NONE',  ( 215.7705878007389515, 15.51487865500265073, -18.20503500338685399 ) ) ;
#1534=EDGE_LOOP ( 'NONE', ( #11958, #14108, #9602, #5050 ) ) ;
#1536=PLANE ( 'NONE',  #8185 ) ;
#1537=EDGE_CURVE ( 'NONE', #9185, #5663, #6711, .T. ) ;
#1541=DIRECTION ( 'NONE',  ( -0.8660254037844358210, -0.5000000000000049960, 0.000000000000000000 ) ) ;
#1543=EDGE_LOOP ( 'NONE', ( #7691, #17063 ) ) ;
#1545=LINE ( 'NONE', #8086, #1740 ) ;
#1546=ORIENTED_EDGE ( 'NONE', *, *, #18168, .T. ) ;
#1548=FACE_OUTER_BOUND ( 'NONE', #20054, .T. ) ;
#1550=AXIS2_PLACEMENT_3D ( 'NONE', #3099, #1508, #11566 ) ;
#1555=CARTESIAN_POINT ( 'NONE',  ( 209.0038672028605617, 11.96213727764295598, -11.52983444460693008 ) ) ;
#1560=VECTOR ( 'NONE', #12071, 1000.000000000000114 ) ;
#1565=ORIENTED_EDGE ( 'NONE', *, *, #4070, .T. ) ;
#1567=CARTESIAN_POINT ( 'NONE',  ( 194.1738290307969805, 7.524008664312185957, -9.972943347741734854 ) ) ;
#1570=ORIENTED_EDGE ( 'NONE', *, *, #10314, .T. ) ;
#1571=ORIENTED_EDGE ( 'NONE', *, *, #12337, .T. ) ;
#1581=VECTOR ( 'NONE', #10544, 1000.000000000000000 ) ;
#1583=DIRECTION ( 'NONE',  ( -0.5943026915289566503, -0.3431208189343668002, 0.7273736415730551741 ) ) ;
#1584=DIRECTION ( 'NONE',  ( -0.8137976813493681405, -0.4698463103929584328, 0.3420201433256762624 ) ) ;
#1587=EDGE_CURVE ( 'NONE', #11760, #1337, #2864, .T. ) ;
#1589=CARTESIAN_POINT ( 'NONE',  ( 208.4761278624580711, 5.007259451653140125, -14.00000000000005507 ) ) ;
#1592=AXIS2_PLACEMENT_3D ( 'NONE', #582, #684, #8524 ) ;
#1593=EDGE_CURVE ( 'NONE', #255, #1746, #12510, .T. ) ;
#1599=CARTESIAN_POINT ( 'NONE',  ( 208.4761278624580711, 5.007259451653140125, -14.00000000000005507 ) ) ;
#1606=DIRECTION ( 'NONE',  ( -0.8089634933040120712, 0.000000000000000000, 0.5878588831525550784 ) ) ;
#1608=FACE_OUTER_BOUND ( 'NONE', #671, .T. ) ;
#1619=CARTESIAN_POINT ( 'NONE',  ( 202.7058429191241089, 0.9029637956749735350, -4.494676796018656439 ) ) ;
#1624=ORIENTED_EDGE ( 'NONE', *, *, #6295, .F. ) ;
#1628=ORIENTED_EDGE ( 'NONE', *, *, #10951, .T. ) ;
#1632=EDGE_CURVE ( 'NONE', #3202, #8339, #7249, .T. ) ;
#1633=ORIENTED_EDGE ( 'NONE', *, *, #16546, .T. ) ;
#1634=CIRCLE ( 'NONE', #17557, 12.47473710546057823 ) ;
#1635=FACE_OUTER_BOUND ( 'NONE', #16500, .T. ) ;
#1636=ADVANCED_FACE ( 'NONE', ( #797 ), #11820, .F. ) ;
#1644=CARTESIAN_POINT ( 'NONE',  ( 207.8564944041415004, 11.29970128344163882, -16.00578157674290125 ) ) ;
#1647=EDGE_CURVE ( 'NONE', #12707, #2199, #5884, .T. ) ;
#1652=CARTESIAN_POINT ( 'NONE',  ( 209.6384834804775608, 12.32853315635724556, -3.125199447383530060 ) ) ;
#1658=CARTESIAN_POINT ( 'NONE',  ( 201.7852296553354563, 11.91845286379962943, -1.053683606938436323 ) ) ;
#1669=ORIENTED_EDGE ( 'NONE', *, *, #20521, .T. ) ;
#1670=ORIENTED_EDGE ( 'NONE', *, *, #2537, .T. ) ;
#1671=CARTESIAN_POINT ( 'NONE',  ( 204.3734207737316808, 2.380946557804465957, -25.29453042277885544 ) ) ;
#1672=DIRECTION ( 'NONE',  ( -0.1503837331804444566, -0.08682408883347132733, -0.9848077530122061329 ) ) ;
#1674=EDGE_LOOP ( 'NONE', ( #3864, #19996, #508, #20023 ) ) ;
#1680=AXIS2_PLACEMENT_3D ( 'NONE', #12486, #10879, #4627 ) ;
#1684=LINE ( 'NONE', #15905, #8770 ) ;
#1685=B_SPLINE_CURVE_WITH_KNOTS ( 'NONE', 3,
 ( #10004, #18194, #3658, #10111 ),
 .UNSPECIFIED., .F., .F.,
 ( 4, 4 ),
 ( 5.762863496319040269E-05, 0.0009116143729456499924 ),
 .UNSPECIFIED. ) ;
#1689=VERTEX_POINT ( 'NONE', #16588 ) ;
#1692=EDGE_LOOP ( 'NONE', ( #15892, #9863, #17810, #13286, #4435, #5929 ) ) ;
#1695=AXIS2_PLACEMENT_3D ( 'NONE', #4115, #2115, #20215 ) ;
#1696=ORIENTED_EDGE ( 'NONE', *, *, #17820, .T. ) ;
#1697=DIRECTION ( 'NONE',  ( -1.000000000000000000, 0.000000000000000000, 2.645739781067712995E-16 ) ) ;
#1701=CARTESIAN_POINT ( 'NONE',  ( 208.8107687779841228, 4.427644383670616079, -14.00000000000005507 ) ) ;
#1707=DIRECTION ( 'NONE',  ( 0.5000000000000049960, -0.8660254037844358210, 0.000000000000000000 ) ) ;
#1709=LINE ( 'NONE', #12961, #11365 ) ;
#1710=CARTESIAN_POINT ( 'NONE',  ( 214.1110484215691656, 14.37972046727219144, -5.993340328401894013 ) ) ;
#1714=CARTESIAN_POINT ( 'NONE',  ( 207.0274154277438754, 3.398024846849156511, -2.233628351993186101 ) ) ;
#1717=LINE ( 'NONE', #16241, #12214 ) ;
#1720=EDGE_CURVE ( 'NONE', #15392, #20411, #15740, .T. ) ;
#1722=ORIENTED_EDGE ( 'NONE', *, *, #9784, .F. ) ;
#1727=ORIENTED_EDGE ( 'NONE', *, *, #6581, .T. ) ;
#1728=VECTOR ( 'NONE', #1778, 1000.000000000000227 ) ;
#1733=DIRECTION ( 'NONE',  ( 0.1503837331804316890, 0.08682408883346424966, -0.9848077530122086864 ) ) ;
#1736=ORIENTED_EDGE ( 'NONE', *, *, #7040, .F. ) ;
#1740=VECTOR ( 'NONE', #11292, 1000.000000000000227 ) ;
#1746=VERTEX_POINT ( 'NONE', #2182 ) ;
#1751=ORIENTED_EDGE ( 'NONE', *, *, #4381, .F. ) ;
#1756=AXIS2_PLACEMENT_3D ( 'NONE', #539, #642, #6989 ) ;
#1759=DIRECTION ( 'NONE',  ( 0.6946590618905487124, 0.4010615963775265858, 0.5971585917027844026 ) ) ;
#1760=VERTEX_POINT ( 'NONE', #14914 ) ;
#1765=EDGE_CURVE ( 'NONE', #17716, #11581, #11935, .T. ) ;
#1766=EDGE_LOOP ( 'NONE', ( #16172, #13234, #3164, #836 ) ) ;
#1767=FACE_OUTER_BOUND ( 'NONE', #11658, .T. ) ;
#1773=LINE ( 'NONE', #13115, #20854 ) ;
#1774=EDGE_LOOP ( 'NONE', ( #1414, #5592, #7610, #17747, #12350, #20491 ) ) ;
#1775=ORIENTED_EDGE ( 'NONE', *, *, #10252, .F. ) ;
#1777=ORIENTED_EDGE ( 'NONE', *, *, #10252, .T. ) ;
#1778=DIRECTION ( 'NONE',  ( -0.5000000000000049960, 0.8660254037844358210, -0.000000000000000000 ) ) ;
#1780=EDGE_CURVE ( 'NONE', #8339, #20025, #11662, .T. ) ;
#1781=ORIENTED_EDGE ( 'NONE', *, *, #13560, .T. ) ;
#1782=EDGE_LOOP ( 'NONE', ( #10897, #13519, #16878, #2698, #556, #15768, #8331 ) ) ;
#1786=ORIENTED_EDGE ( 'NONE', *, *, #277, .T. ) ;
#1788=B_SPLINE_CURVE_WITH_KNOTS ( 'NONE', 3,
 ( #17763, #3231, #11396, #7892 ),
 .UNSPECIFIED., .F., .F.,
 ( 4, 4 ),
 ( 4.692417266429781039E-07, 0.0008544549797053814250 ),
 .UNSPECIFIED. ) ;
#1790=ADVANCED_FACE ( 'NONE', ( #18601 ), #17016, .F. ) ;
#1797=DIRECTION ( 'NONE',  ( -0.5000000000000054401, 0.8660254037844354880, -0.000000000000000000 ) ) ;
#1801=DIRECTION ( 'NONE',  ( -0.8660254037844355990, -0.5000000000000054401, 2.642119490368404866E-15 ) ) ;
#1802=ORIENTED_EDGE ( 'NONE', *, *, #8441, .F. ) ;
#1805=ORIENTED_EDGE ( 'NONE', *, *, #20779, .T. ) ;
#1812=CARTESIAN_POINT ( 'NONE',  ( 215.3534639294407782, 15.62807865697965504, -9.913166705713923221 ) ) ;
#1816=CARTESIAN_POINT ( 'NONE',  ( 205.0662616026534693, 10.91332106064940888, -14.00000000000005507 ) ) ;
#1817=LINE ( 'NONE', #20687, #12630 ) ;
#1818=VERTEX_POINT ( 'NONE', #7669 ) ;
#1822=ORIENTED_EDGE ( 'NONE', *, *, #1008, .F. ) ;
#1825=ADVANCED_FACE ( 'NONE', ( #12567 ), #9281, .T. ) ;
#1830=CIRCLE ( 'NONE', #8241, 1.000000000000000888 ) ;
#1831=B_SPLINE_CURVE_WITH_KNOTS ( 'NONE', 3,
 ( #3340, #1858, #9789, #13205 ),
 .UNSPECIFIED., .F., .F.,
 ( 4, 4 ),
 ( 4.499189576780315060E-05, 0.0008989776337512245903 ),
 .UNSPECIFIED. ) ;
#1832=EDGE_LOOP ( 'NONE', ( #8388, #6845, #1751, #131, #19942, #18550 ) ) ;
#1836=ORIENTED_EDGE ( 'NONE', *, *, #8767, .T. ) ;
#1838=ORIENTED_EDGE ( 'NONE', *, *, #1765, .F. ) ;
#1844=EDGE_CURVE ( 'NONE', #20139, #4463, #10999, .T. ) ;
#1846=AXIS2_PLACEMENT_3D ( 'NONE', #15131, #19763, #13521 ) ;
#1849=ORIENTED_EDGE ( 'NONE', *, *, #13049, .F. ) ;
#1850=EDGE_CURVE ( 'NONE', #20019, #13147, #15755, .T. ) ;
#1853=VERTEX_POINT ( 'NONE', #5967 ) ;
#1858=CARTESIAN_POINT ( 'NONE',  ( 216.7437086208277321, 9.265328561208580282, -21.78787861992518415 ) ) ;
#1863=ORIENTED_EDGE ( 'NONE', *, *, #11828, .F. ) ;
#1867=ADVANCED_FACE ( 'NONE', ( #2609 ), #2815, .F. ) ;
#1872=EDGE_CURVE ( 'NONE', #12920, #3711, #10863, .T. ) ;
#1873=DIRECTION ( 'NONE',  ( 0.5000000000000055511, -0.8660254037844353769, 2.775557561562890735E-17 ) ) ;
#1876=EDGE_LOOP ( 'NONE', ( #7394, #14928, #19480, #9817 ) ) ;
#1877=EDGE_LOOP ( 'NONE', ( #5949, #5091, #15998, #9190 ) ) ;
#1878=EDGE_LOOP ( 'NONE', ( #3906, #8354, #1025, #3153 ) ) ;
#1879=DIRECTION ( 'NONE',  ( -0.8089634933040207310, 0.000000000000000000, -0.5878588831525431990 ) ) ;
#1888=ORIENTED_EDGE ( 'NONE', *, *, #15850, .F. ) ;
#1889=EDGE_CURVE ( 'NONE', #10818, #1853, #14056, .T. ) ;
#1899=FACE_OUTER_BOUND ( 'NONE', #4390, .T. ) ;
#1901=EDGE_CURVE ( 'NONE', #2978, #13943, #902, .T. ) ;
#1906=EDGE_CURVE ( 'NONE', #13379, #18096, #15079, .T. ) ;
#1911=CARTESIAN_POINT ( 'NONE',  ( 210.5178922176470451, 5.670851784906956183, -2.061577111287821840 ) ) ;
#1916=DIRECTION ( 'NONE',  ( 0.5000000000000054401, -0.8660254037844354880, 0.000000000000000000 ) ) ;
#1917=EDGE_CURVE ( 'NONE', #14639, #2132, #3024, .T. ) ;
#1920=VECTOR ( 'NONE', #16064, 999.9999999999998863 ) ;
#1926=CARTESIAN_POINT ( 'NONE',  ( 207.8872982515397609, 15.44148381043179263, -24.85758746085098991 ) ) ;
#1927=VERTEX_POINT ( 'NONE', #14480 ) ;
#1930=CARTESIAN_POINT ( 'NONE',  ( 215.9000602621138114, 8.778247954203701298, -22.82042918318467173 ) ) ;
#1931=ORIENTED_EDGE ( 'NONE', *, *, #1780, .F. ) ;
#1933=CARTESIAN_POINT ( 'NONE',  ( 200.4233784773551861, 6.654163220837372883, -3.334988897836806299 ) ) ;
#1942=ORIENTED_EDGE ( 'NONE', *, *, #6092, .T. ) ;
#1946=LINE ( 'NONE', #16883, #6090 ) ;
#1956=CARTESIAN_POINT ( 'NONE',  ( 205.8264633344831225, 9.596613037118636669, -14.00000000000005507 ) ) ;
#1959=ADVANCED_FACE ( 'NONE', ( #9873 ), #3543, .T. ) ;
#1967=VECTOR ( 'NONE', #3429, 1000.000000000000227 ) ;
#1968=EDGE_CURVE ( 'NONE', #15950, #18037, #16419, .T. ) ;
#1976=FACE_OUTER_BOUND ( 'NONE', #20668, .T. ) ;
#1977=DIRECTION ( 'NONE',  ( 0.5000000000000049960, -0.8660254037844358210, 0.000000000000000000 ) ) ;
#1978=( GEOMETRIC_REPRESENTATION_CONTEXT ( 3 ) GLOBAL_UNCERTAINTY_ASSIGNED_CONTEXT ( ( #8067 ) ) GLOBAL_UNIT_ASSIGNED_CONTEXT ( ( #11108, #10782, #1360 ) ) REPRESENTATION_CONTEXT ( 'NONE', 'WORKASPACE' ) );
#1982=ORIENTED_EDGE ( 'NONE', *, *, #19125, .T. ) ;
#1984=CARTESIAN_POINT ( 'NONE',  ( 215.8997106868019387, 9.293266993639628382, -23.06309126349817618 ) ) ;
#1987=ORIENTED_EDGE ( 'NONE', *, *, #4381, .T. ) ;
#1990=LINE ( 'NONE', #16611, #4096 ) ;
#1991=CARTESIAN_POINT ( 'NONE',  ( 213.9207374538404736, 14.44686705926026882, -6.091045511237016541 ) ) ;
#1994=FACE_OUTER_BOUND ( 'NONE', #18121, .T. ) ;
#1995=EDGE_CURVE ( 'NONE', #15941, #18395, #13922, .T. ) ;
#1997=EDGE_CURVE ( 'NONE', #16845, #4228, #19716, .T. ) ;
#1998=CARTESIAN_POINT ( 'NONE',  ( 216.3390813779211612, 15.84309857482137396, -12.56470246848408223 ) ) ;
#1999=CONICAL_SURFACE ( 'NONE', #16232, 13.07248899748297433, 0.6693469023067423196 ) ;
#2000=DIRECTION ( 'NONE',  ( -0.8660254037844354880, -0.5000000000000055511, 0.000000000000000000 ) ) ;
#2003=PLANE ( 'NONE',  #11847 ) ;
#2011=VERTEX_POINT ( 'NONE', #11382 ) ;
#2014=DIRECTION ( 'NONE',  ( -0.8660254037844358210, -0.5000000000000049960, 0.000000000000000000 ) ) ;
#2020=CARTESIAN_POINT ( 'NONE',  ( 208.8627203077920171, 26.61931772755388081, -19.61257667712965258 ) ) ;
#2025=CARTESIAN_POINT ( 'NONE',  ( 207.4098631234038521, 11.04183859327925354, -25.80036831778744144 ) ) ;
#2027=EDGE_CURVE ( 'NONE', #8176, #2805, #11482, .T. ) ;
#2029=CARTESIAN_POINT ( 'NONE',  ( 205.5965122587965084, 9.994899983462953941, -14.00000000000005507 ) ) ;
#2030=CIRCLE ( 'NONE', #11853, 12.47473710546057823 ) ;
#2031=CARTESIAN_POINT ( 'NONE',  ( 215.7517163971578782, 8.326610718103061970, -14.00000000000005329 ) ) ;
#2032=CARTESIAN_POINT ( 'NONE',  ( 215.8998893078988033, 9.035756268811685032, -22.94176278698385119 ) ) ;
#2041=VERTEX_POINT ( 'NONE', #7879 ) ;
#2044=VECTOR ( 'NONE', #16175, 1000.000000000000227 ) ;
#2054=VECTOR ( 'NONE', #4786, 1000.000000000000114 ) ;
#2057=ORIENTED_EDGE ( 'NONE', *, *, #7860, .T. ) ;
#2058=CIRCLE ( 'NONE', #1046, 12.47473710546057823 ) ;
#2059=CARTESIAN_POINT ( 'NONE',  ( 218.1364845712607803, 10.58466899794828642, -8.415281845792092597 ) ) ;
#2066=ORIENTED_EDGE ( 'NONE', *, *, #1593, .T. ) ;
#2068=CARTESIAN_POINT ( 'NONE',  ( 208.4761278624580711, 5.007259451653140125, -14.00000000000005507 ) ) ;
#2070=CARTESIAN_POINT ( 'NONE',  ( 195.9595725116093945, 4.431010226260183593, -9.972943347741736630 ) ) ;
#2080=CARTESIAN_POINT ( 'NONE',  ( 205.0662616026534693, 10.91332106064940888, -14.00000000000005507 ) ) ;
#2084=CARTESIAN_POINT ( 'NONE',  ( 212.8019350911804963, 7.247151567852217369, -25.29453042277899755 ) ) ;
#2085=CARTESIAN_POINT ( 'NONE',  ( 207.4176018615383441, 11.04630655582438337, -15.90550977090996909 ) ) ;
#2087=CIRCLE ( 'NONE', #20689, 4.730184897849355252 ) ;
#2103=CARTESIAN_POINT ( 'NONE',  ( 208.8107687779841228, 4.427644383670616079, -14.00000000000005507 ) ) ;
#2109=AXIS2_PLACEMENT_3D ( 'NONE', #7229, #13712, #20164 ) ;
#2112=DIRECTION ( 'NONE',  ( -0.8645602258681719388, -0.4991540791356394169, -0.05814482891046558050 ) ) ;
#2114=CARTESIAN_POINT ( 'NONE',  ( 206.2878473285719281, 10.21703256791452041, -1.872710068124176841 ) ) ;
#2115=DIRECTION ( 'NONE',  ( -0.5000000000000054401, 0.8660254037844354880, -0.000000000000000000 ) ) ;
#2116=DIRECTION ( 'NONE',  ( 0.5000000000000054401, -0.8660254037844354880, 0.000000000000000000 ) ) ;
#2121=EDGE_CURVE ( 'NONE', #18641, #13417, #8613, .T. ) ;
#2123=EDGE_CURVE ( 'NONE', #7107, #10758, #6797, .T. ) ;
#2125=CARTESIAN_POINT ( 'NONE',  ( 218.6326489791658503, 10.87112965241456841, -18.25196083293883120 ) ) ;
#2126=AXIS2_PLACEMENT_3D ( 'NONE', #5501, #18134, #3606 ) ;
#2127=VECTOR ( 'NONE', #20616, 1000.000000000000114 ) ;
#2128=ORIENTED_EDGE ( 'NONE', *, *, #4038, .F. ) ;
#2129=LINE ( 'NONE', #14865, #7674 ) ;
#2131=EDGE_CURVE ( 'NONE', #4355, #3665, #15432, .T. ) ;
#2132=VERTEX_POINT ( 'NONE', #11909 ) ;
#2134=DIRECTION ( 'NONE',  ( 0.000000000000000000, 0.000000000000000000, -1.000000000000000000 ) ) ;
#2137=CARTESIAN_POINT ( 'NONE',  ( 195.6285356662269237, 4.239886014466930142, -11.24974199967268618 ) ) ;
#2138=VECTOR ( 'NONE', #10774, 1000.000000000000227 ) ;
#2143=VERTEX_POINT ( 'NONE', #16569 ) ;
#2145=EDGE_CURVE ( 'NONE', #4987, #1053, #18374, .T. ) ;
#2148=EDGE_LOOP ( 'NONE', ( #6519, #11364, #16039, #18985 ) ) ;
#2154=EDGE_LOOP ( 'NONE', ( #10992, #18674, #1110, #16450 ) ) ;
#2157=CARTESIAN_POINT ( 'NONE',  ( 211.5875185857062206, 6.803621723274593691, -25.94618751764496878 ) ) ;
#2160=CARTESIAN_POINT ( 'NONE',  ( 219.2049426021622764, 11.20154352970703471, -12.53629070788368338 ) ) ;
#2161=EDGE_CURVE ( 'NONE', #16889, #14507, #3838, .T. ) ;
#2168=LINE ( 'NONE', #8619, #17284 ) ;
#2171=EDGE_CURVE ( 'NONE', #3291, #4535, #15006, .T. ) ;
#2172=ORIENTED_EDGE ( 'NONE', *, *, #17565, .F. ) ;
#2174=VERTEX_POINT ( 'NONE', #20064 ) ;
#2177=CARTESIAN_POINT ( 'NONE',  ( 208.4761278624580711, 5.007259451653140125, -14.00000000000005507 ) ) ;
#2182=CARTESIAN_POINT ( 'NONE',  ( 195.6699422177752581, 3.732742836357164862, -18.25196083293855054 ) ) ;
#2187=LINE ( 'NONE', #20401, #9823 ) ;
#2190=DIRECTION ( 'NONE',  ( -0.8660254037844358210, -0.5000000000000049960, 0.000000000000000000 ) ) ;
#2192=DIRECTION ( 'NONE',  ( -0.5000000000000051070, 0.8660254037844359321, -0.000000000000000000 ) ) ;
#2194=ORIENTED_EDGE ( 'NONE', *, *, #8580, .F. ) ;
#2195=ORIENTED_EDGE ( 'NONE', *, *, #1632, .T. ) ;
#2198=PLANE ( 'NONE',  #15254 ) ;
#2199=VERTEX_POINT ( 'NONE', #11799 ) ;
#2200=VERTEX_POINT ( 'NONE', #5526 ) ;
#2209=EDGE_CURVE ( 'NONE', #5382, #13116, #19946, .T. ) ;
#2213=DIRECTION ( 'NONE',  ( 0.5000000000000054401, -0.8660254037844354880, 0.000000000000000000 ) ) ;
#2216=CARTESIAN_POINT ( 'NONE',  ( 213.3559741392790556, 18.59882530632892994, -21.18305361806777398 ) ) ;
#2218=ORIENTED_EDGE ( 'NONE', *, *, #19902, .F. ) ;
#2222=DIRECTION ( 'NONE',  ( -0.9987303135603804449, 0.000000000000000000, 0.05037619254751497799 ) ) ;
#2223=CARTESIAN_POINT ( 'NONE',  ( 220.1325240088992814, 10.96426281393859981, -15.47241223420017775 ) ) ;
#2225=AXIS2_PLACEMENT_3D ( 'NONE', #768, #10278, #10383 ) ;
#2226=ORIENTED_EDGE ( 'NONE', *, *, #11032, .F. ) ;
#2231=ORIENTED_EDGE ( 'NONE', *, *, #8439, .T. ) ;
#2234=EDGE_CURVE ( 'NONE', #5663, #14662, #1946, .T. ) ;
#2237=CARTESIAN_POINT ( 'NONE',  ( 214.9988779556950078, 8.000350883196837515, -23.57241037536588735 ) ) ;
#2238=DIRECTION ( 'NONE',  ( -0.8426815769442687065, -0.4865224352899185645, -0.2306158707424266763 ) ) ;
#2241=DIRECTION ( 'NONE',  ( 0.5000000000000054401, -0.8660254037844354880, 0.000000000000000000 ) ) ;
#2244=VERTEX_POINT ( 'NONE', #9327 ) ;
#2247=VERTEX_POINT ( 'NONE', #2683 ) ;
#2248=DIRECTION ( 'NONE',  ( -0.5000000000000051070, 0.8660254037844359321, -0.000000000000000000 ) ) ;
#2255=DIRECTION ( 'NONE',  ( 0.5000000000000051070, -0.8660254037844359321, 0.000000000000000000 ) ) ;
#2257=CARTESIAN_POINT ( 'NONE',  ( 198.4369456227295245, 5.507295677492109576, -5.040853264743329731 ) ) ;
#2261=EDGE_CURVE ( 'NONE', #20843, #16845, #18974, .T. ) ;
#2262=CARTESIAN_POINT ( 'NONE',  ( 208.0931370707057226, 4.270918748101473206, -26.10149651730435494 ) ) ;
#2263=CARTESIAN_POINT ( 'NONE',  ( 209.9432949659958183, 27.24318779734733553, -12.53629070788368338 ) ) ;
#2265=ORIENTED_EDGE ( 'NONE', *, *, #15773, .F. ) ;
#2267=DIRECTION ( 'NONE',  ( -0.8660254037844354880, -0.5000000000000055511, 0.000000000000000000 ) ) ;
#2274=CARTESIAN_POINT ( 'NONE',  ( 192.3204675648519242, 17.06864365341445477, -14.00000000000005507 ) ) ;
#2277=ORIENTED_EDGE ( 'NONE', *, *, #1587, .T. ) ;
#2278=EDGE_CURVE ( 'NONE', #1760, #20025, #15627, .T. ) ;
#2286=CARTESIAN_POINT ( 'NONE',  ( 210.5718816476998256, 5.444423373074280370, -2.341985411377013548 ) ) ;
#2290=DIRECTION ( 'NONE',  ( 0.3886714912512189701, 0.2243995901002275584, -0.8936326403234180482 ) ) ;
#2291=DIRECTION ( 'NONE',  ( 0.5000000000000051070, -0.8660254037844359321, 0.000000000000000000 ) ) ;
#2293=FACE_OUTER_BOUND ( 'NONE', #20113, .T. ) ;
#2295=CARTESIAN_POINT ( 'NONE',  ( 206.4681030732283205, 9.967063913005945963, -26.45271578590685380 ) ) ;
#2296=EDGE_CURVE ( 'NONE', #3214, #5044, #12539, .T. ) ;
#2297=VERTEX_POINT ( 'NONE', #1092 ) ;
#2299=EDGE_LOOP ( 'NONE', ( #5299, #19836, #10972, #16721 ) ) ;
#2304=TOROIDAL_SURFACE ( 'NONE', #5312, 2.961423854602172501, 1.000000000000000000 ) ;
#2306=DIRECTION ( 'NONE',  ( -0.5000000000000051070, 0.8660254037844359321, -0.000000000000000000 ) ) ;
#2308=ADVANCED_FACE ( 'NONE', ( #12113 ), #18657, .T. ) ;
#2309=AXIS2_PLACEMENT_3D ( 'NONE', #5495, #8995, #15497 ) ;
#2310=FACE_OUTER_BOUND ( 'NONE', #12343, .T. ) ;
#2311=CARTESIAN_POINT ( 'NONE',  ( 203.0861028855985069, 1.895327080324426428, -3.188775577416750995 ) ) ;
#2314=ADVANCED_FACE ( 'NONE', ( #20372 ), #982, .T. ) ;
#2315=B_SPLINE_CURVE_WITH_KNOTS ( 'NONE', 3,
 ( #3925, #15506, #1073, #759 ),
 .UNSPECIFIED., .F., .F.,
 ( 4, 4 ),
 ( 4.203583920150003484E-07, 0.0008544060963757356712 ),
 .UNSPECIFIED. ) ;
#2320=DIRECTION ( 'NONE',  ( -0.8528685319524387243, -0.4924038765061080070, 0.1736481776669413502 ) ) ;
#2327=ORIENTED_EDGE ( 'NONE', *, *, #16127, .F. ) ;
#2329=ORIENTED_EDGE ( 'NONE', *, *, #20256, .T. ) ;
#2339=CARTESIAN_POINT ( 'NONE',  ( 214.9458835816058979, 7.969754567050957306, -23.47937149798938350 ) ) ;
#2342=LINE ( 'NONE', #20452, #4135 ) ;
#2344=DIRECTION ( 'NONE',  ( 0.5000000000000051070, -0.8660254037844355990, 0.000000000000000000 ) ) ;
#2346=DIRECTION ( 'NONE',  ( -0.8660254037844355990, -0.5000000000000054401, 2.044166132021871316E-14 ) ) ;
#2348=VECTOR ( 'NONE', #15597, 999.9999999999998863 ) ;
#2354=ADVANCED_FACE ( 'NONE', ( #13919 ), #9824, .T. ) ;
#2361=DIRECTION ( 'NONE',  ( 0.8660254037844355990, 0.5000000000000054401, 0.000000000000000000 ) ) ;
#2362=CARTESIAN_POINT ( 'NONE',  ( 196.2195613929434899, 4.227088295528298900, -8.480087152951162111 ) ) ;
#2365=ADVANCED_FACE ( 'NONE', ( #18899 ), #14950, .T. ) ;
#2366=CARTESIAN_POINT ( 'NONE',  ( 217.5077365114557608, 9.448841045723993304, -22.49869731917979010 ) ) ;
#2368=VERTEX_POINT ( 'NONE', #15734 ) ;
#2369=CARTESIAN_POINT ( 'NONE',  ( 213.7874248973967610, 18.84792351767029572, -16.70797078425240656 ) ) ;
#2371=DIRECTION ( 'NONE',  ( 0.5000000000000052180, -0.8660254037844355990, -0.000000000000000000 ) ) ;
#2373=EDGE_CURVE ( 'NONE', #13537, #7703, #14250, .T. ) ;
#2381=CARTESIAN_POINT ( 'NONE',  ( 219.0841311483638947, 10.35897291369198747, -15.40190399002830723 ) ) ;
#2391=ORIENTED_EDGE ( 'NONE', *, *, #14474, .F. ) ;
#2392=DIRECTION ( 'NONE',  ( 0.8660254037844355990, 0.5000000000000054401, 0.000000000000000000 ) ) ;
#2394=EDGE_CURVE ( 'NONE', #4803, #4463, #14455, .T. ) ;
#2399=ORIENTED_EDGE ( 'NONE', *, *, #5489, .T. ) ;
#2401=CARTESIAN_POINT ( 'NONE',  ( 209.4254563108873413, 4.782534396259798370, -2.075899210536075401 ) ) ;
#2402=CARTESIAN_POINT ( 'NONE',  ( 203.0627220339503936, 1.881828139331499727, -24.79563718815128226 ) ) ;
#2404=VECTOR ( 'NONE', #96, 1000.000000000000227 ) ;
#2411=DIRECTION ( 'NONE',  ( -0.8601696498176563122, -0.4966191788709776733, -0.1160929141252233648 ) ) ;
#2412=FACE_OUTER_BOUND ( 'NONE', #9581, .T. ) ;
#2424=ORIENTED_EDGE ( 'NONE', *, *, #16699, .T. ) ;
#2426=CIRCLE ( 'NONE', #14296, 12.47473710546057823 ) ;
#2428=ORIENTED_EDGE ( 'NONE', *, *, #17412, .F. ) ;
#2429=EDGE_LOOP ( 'NONE', ( #1493, #12041, #20542, #18730, #10468, #7009 ) ) ;
#2435=DIRECTION ( 'NONE',  ( 0.5000000000000054401, -0.8660254037844354880, 0.000000000000000000 ) ) ;
#2436=ADVANCED_FACE ( 'NONE', ( #1608 ), #9435, .T. ) ;
#2439=CARTESIAN_POINT ( 'NONE',  ( 207.6891655446386551, 10.67204465957205350, -26.28791492288521781 ) ) ;
#2445=VECTOR ( 'NONE', #15907, 1000.000000000000114 ) ;
#2448=AXIS2_PLACEMENT_3D ( 'NONE', #781, #7331, #15112 ) ;
#2452=VERTEX_POINT ( 'NONE', #16044 ) ;
#2454=LINE ( 'NONE', #14230, #14712 ) ;
#2460=AXIS2_PLACEMENT_3D ( 'NONE', #6433, #16521, #11434 ) ;
#2467=ORIENTED_EDGE ( 'NONE', *, *, #3686, .F. ) ;
#2468=CARTESIAN_POINT ( 'NONE',  ( 211.7141293194486025, 6.361499597646727011, -2.388950188371981032 ) ) ;
#2470=AXIS2_PLACEMENT_3D ( 'NONE', #14671, #128, #16344 ) ;
#2472=DIRECTION ( 'NONE',  ( -0.5000000000000054401, 0.8660254037844354880, -0.000000000000000000 ) ) ;
#2473=ORIENTED_EDGE ( 'NONE', *, *, #20493, .F. ) ;
#2474=VECTOR ( 'NONE', #19048, 1000.000000000000114 ) ;
#2477=DIRECTION ( 'NONE',  ( 0.1005394128318209540, 0.05804645706261960664, 0.9932383577419421350 ) ) ;
#2486=CARTESIAN_POINT ( 'NONE',  ( 212.6158184066919716, 14.04749827747483693, -22.62267072728679906 ) ) ;
#2487=AXIS2_PLACEMENT_3D ( 'NONE', #18427, #15476, #12068 ) ;
#2488=ORIENTED_EDGE ( 'NONE', *, *, #3032, .F. ) ;
#2490=CARTESIAN_POINT ( 'NONE',  ( 205.6550139379351663, 24.76734759143572262, -24.01557619556987788 ) ) ;
#2491=CARTESIAN_POINT ( 'NONE',  ( 211.7681187495013830, 6.135071185814040540, -2.669358488461178069 ) ) ;
#2493=EDGE_CURVE ( 'NONE', #6314, #20898, #21, .T. ) ;
#2494=FACE_OUTER_BOUND ( 'NONE', #20816, .T. ) ;
#2500=CARTESIAN_POINT ( 'NONE',  ( 219.0136128684463870, 10.31825916579886382, -8.145074743996644884 ) ) ;
#2502=CARTESIAN_POINT ( 'NONE',  ( 205.6089461623839441, 14.12607661844890039, -25.65046807331635748 ) ) ;
#2505=VERTEX_POINT ( 'NONE', #11260 ) ;
#2509=CARTESIAN_POINT ( 'NONE',  ( 217.9776690748798558, 9.720156737717866591, -19.29168348739315775 ) ) ;
#2510=CARTESIAN_POINT ( 'NONE',  ( 199.4574108924007305, -0.1996992187545574282, -7.132002368301175288 ) ) ;
#2515=DIRECTION ( 'NONE',  ( 0.1997192025788092351, 0.1153079353712145594, -0.9730448705798270259 ) ) ;
#2517=EDGE_LOOP ( 'NONE', ( #13399, #4945, #9576, #14159 ) ) ;
#2521=CARTESIAN_POINT ( 'NONE',  ( 205.8264633344831225, 9.596613037118636669, -14.00000000000005507 ) ) ;
#2523=CARTESIAN_POINT ( 'NONE',  ( 199.3931344365919927, 6.236368223744671369, -4.253719131806056986 ) ) ;
#2525=CARTESIAN_POINT ( 'NONE',  ( 205.2117758015800462, 9.241723024529527208, -1.545471579934808215 ) ) ;
#2526=EDGE_CURVE ( 'NONE', #772, #9185, #16908, .T. ) ;
#2532=DIRECTION ( 'NONE',  ( 0.5000000000000049960, -0.8660254037844358210, 0.000000000000000000 ) ) ;
#2535=ORIENTED_EDGE ( 'NONE', *, *, #19238, .F. ) ;
#2537=EDGE_CURVE ( 'NONE', #20176, #19523, #12107, .T. ) ;
#2544=DIRECTION ( 'NONE',  ( -0.8660254037844355990, -0.5000000000000054401, -3.615531934188343626E-15 ) ) ;
#2548=CARTESIAN_POINT ( 'NONE',  ( 212.7272071507568967, 14.11180859884542649, -5.291540431471497996 ) ) ;
#2549=ADVANCED_FACE ( 'NONE', ( #8121 ), #20341, .F. ) ;
#2550=CARTESIAN_POINT ( 'NONE',  ( 211.6495311407713018, 17.61360998178372483, -6.376588578941996488 ) ) ;
#2552=AXIS2_PLACEMENT_3D ( 'NONE', #15146, #2192, #11834 ) ;
#2553=LINE ( 'NONE', #7400, #4712 ) ;
#2554=EDGE_CURVE ( 'NONE', #19224, #15951, #3261, .T. ) ;
#2561=CARTESIAN_POINT ( 'NONE',  ( 205.8264633344831225, 9.596613037118636669, -14.00000000000005507 ) ) ;
#2564=CIRCLE ( 'NONE', #5238, 12.47473710546057823 ) ;
#2567=ORIENTED_EDGE ( 'NONE', *, *, #8251, .F. ) ;
#2575=EDGE_CURVE ( 'NONE', #3665, #9396, #10168, .T. ) ;
#2579=ORIENTED_EDGE ( 'NONE', *, *, #4235, .F. ) ;
#2580=CIRCLE ( 'NONE', #14438, 11.94520687646042667 ) ;
#2590=CARTESIAN_POINT ( 'NONE',  ( 205.8311783259423464, 2.707377034109388347, -2.561001429077326197 ) ) ;
#2591=ORIENTED_EDGE ( 'NONE', *, *, #10824, .T. ) ;
#2593=DIRECTION ( 'NONE',  ( 0.5000000000000027756, -0.8660254037844372643, 0.000000000000000000 ) ) ;
#2594=CARTESIAN_POINT ( 'NONE',  ( 211.2164883113428857, 12.70854540844746872, -3.188775577416895324 ) ) ;
#2595=DIRECTION ( 'NONE',  ( -0.8660254037844355990, -0.5000000000000054401, 2.044166132021871316E-14 ) ) ;
#2597=ORIENTED_EDGE ( 'NONE', *, *, #12642, .F. ) ;
#2599=ORIENTED_EDGE ( 'NONE', *, *, #6392, .F. ) ;
#2609=FACE_OUTER_BOUND ( 'NONE', #13876, .T. ) ;
#2615=CARTESIAN_POINT ( 'NONE',  ( 208.0983737146324870, 5.661548828456886895, -14.00000000000005507 ) ) ;
#2617=DIRECTION ( 'NONE',  ( 0.7951984747223628247, 0.4591080534401421609, 0.3960797660391544572 ) ) ;
#2619=ORIENTED_EDGE ( 'NONE', *, *, #15165, .F. ) ;
#2621=DIRECTION ( 'NONE',  ( -0.8660254037844357100, -0.5000000000000051070, 0.000000000000000000 ) ) ;
#2626=CARTESIAN_POINT ( 'NONE',  ( 200.4142678326970213, 6.648903187691491468, -24.65893733905786078 ) ) ;
#2627=FACE_OUTER_BOUND ( 'NONE', #9159, .T. ) ;
#2629=EDGE_CURVE ( 'NONE', #10364, #340, #12712, .T. ) ;
#2636=DIRECTION ( 'NONE',  ( -0.4330127018922106941, -0.2499999999999983347, 0.8660254037844433705 ) ) ;
#2639=ORIENTED_EDGE ( 'NONE', *, *, #12097, .T. ) ;
#2641=DIRECTION ( 'NONE',  ( -0.5000000000000049960, 0.8660254037844357100, -0.000000000000000000 ) ) ;
#2644=VERTEX_POINT ( 'NONE', #8553 ) ;
#2646=CARTESIAN_POINT ( 'NONE',  ( 206.4249228987308413, 10.47318308942859133, -13.04168858804099784 ) ) ;
#2655=CARTESIAN_POINT ( 'NONE',  ( 199.2231352798573027, 21.03391272677540513, -14.00000000000005507 ) ) ;
#2658=DIRECTION ( 'NONE',  ( -0.8660254037844357100, -0.5000000000000049960, 0.000000000000000000 ) ) ;
#2661=CARTESIAN_POINT ( 'NONE',  ( 193.8341126585712857, 7.327873325359597345, -16.70797078425209392 ) ) ;
#2662=CARTESIAN_POINT ( 'NONE',  ( 208.6806335619233153, 11.77551824803669689, -26.30940818168328477 ) ) ;
#2664=LINE ( 'NONE', #12320, #14185 ) ;
#2666=CARTESIAN_POINT ( 'NONE',  ( 208.4761278624580711, 5.007259451653140125, -14.00000000000005507 ) ) ;
#2673=CARTESIAN_POINT ( 'NONE',  ( 205.0662616026534693, 10.91332106064940888, -14.00000000000005507 ) ) ;
#2674=DIRECTION ( 'NONE',  ( 0.8528685319524407227, 0.4924038765061096168, 0.1736481776669271115 ) ) ;
#2680=CARTESIAN_POINT ( 'NONE',  ( 211.7903592300262119, 6.147911733231966380, -2.561001429077395475 ) ) ;
#2681=CARTESIAN_POINT ( 'NONE',  ( 201.4921241270915857, 0.4598221481815398803, -5.186396688528427390 ) ) ;
#2683=CARTESIAN_POINT ( 'NONE',  ( 212.2669970461267042, 13.31505690926096364, -24.01557619556987788 ) ) ;
#2689=CARTESIAN_POINT ( 'NONE',  ( 205.5965122587965084, 9.994899983462953941, -14.00000000000005507 ) ) ;
#2690=CARTESIAN_POINT ( 'NONE',  ( 205.5965122587965084, 9.994899983462953941, -14.00000000000005507 ) ) ;
#2698=ORIENTED_EDGE ( 'NONE', *, *, #1537, .F. ) ;
#2700=VECTOR ( 'NONE', #20829, 1000.000000000000227 ) ;
#2703=ORIENTED_EDGE ( 'NONE', *, *, #12792, .F. ) ;
#2704=EDGE_CURVE ( 'NONE', #17213, #11315, #15258, .T. ) ;
#2707=B_SPLINE_CURVE_WITH_KNOTS ( 'NONE', 3,
 ( #18022, #4875, #9737, #3493 ),
 .UNSPECIFIED., .F., .F.,
 ( 4, 4 ),
 ( 2.946819598302503673E-07, 0.0008542804199448367306 ),
 .UNSPECIFIED. ) ;
#2710=VERTEX_POINT ( 'NONE', #7167 ) ;
#2713=VECTOR ( 'NONE', #15106, 1000.000000000000114 ) ;
#2715=CARTESIAN_POINT ( 'NONE',  ( 199.9261466397861113, -0.4442953756591617176, -7.343163769975552313 ) ) ;
#2719=CARTESIAN_POINT ( 'NONE',  ( 215.9094043865061110, 15.77204112533624958, -11.19512133156266032 ) ) ;
#2723=EDGE_LOOP ( 'NONE', ( #19092, #6082, #335, #2194, #8230, #7344 ) ) ;
#2725=VERTEX_POINT ( 'NONE', #13546 ) ;
#2731=AXIS2_PLACEMENT_3D ( 'NONE', #11154, #7964, #1104 ) ;
#2732=ORIENTED_EDGE ( 'NONE', *, *, #16416, .F. ) ;
#2737=CARTESIAN_POINT ( 'NONE',  ( 209.0908153953612612, 5.362149464242316199, -1.545471579934816875 ) ) ;
#2738=LINE ( 'NONE', #5895, #8445 ) ;
#2742=ORIENTED_EDGE ( 'NONE', *, *, #20819, .F. ) ;
#2743=VECTOR ( 'NONE', #14626, 1000.000000000000227 ) ;
#2745=CARTESIAN_POINT ( 'NONE',  ( 208.8026598822967514, 11.49194359559607115, -2.204078039983189630 ) ) ;
#2760=AXIS2_PLACEMENT_3D ( 'NONE', #8227, #19377, #17790 ) ;
#2762=CARTESIAN_POINT ( 'NONE',  ( 216.6299025733443102, 15.83398158984899240, -14.00000000000005507 ) ) ;
#2770=CARTESIAN_POINT ( 'NONE',  ( 208.5625094892126583, 11.70731928285941770, -25.48492467622476099 ) ) ;
#2779=VECTOR ( 'NONE', #3257, 1000.000000000000227 ) ;
#2782=CARTESIAN_POINT ( 'NONE',  ( 199.4915863999364660, 6.470219395467344370, -4.494676796018650222 ) ) ;
#2787=DIRECTION ( 'NONE',  ( -0.5000000000000049960, 0.8660254037844357100, -0.000000000000000000 ) ) ;
#2788=EDGE_CURVE ( 'NONE', #3973, #3166, #1990, .T. ) ;
#2798=DIRECTION ( 'NONE',  ( 0.5000000000000055511, -0.8660254037844353769, -3.885780586188047891E-16 ) ) ;
#2805=VERTEX_POINT ( 'NONE', #15568 ) ;
#2806=EDGE_LOOP ( 'NONE', ( #11116, #1546, #14669, #20944 ) ) ;
#2815=PLANE ( 'NONE',  #161 ) ;
#2821=EDGE_CURVE ( 'NONE', #10684, #11395, #8310, .T. ) ;
#2827=CARTESIAN_POINT ( 'NONE',  ( 199.2144802262915846, 21.04890371929339921, -14.00000000000005507 ) ) ;
#2828=EDGE_CURVE ( 'NONE', #11210, #9561, #10761, .T. ) ;
#2829=EDGE_LOOP ( 'NONE', ( #17064, #1727, #12572, #7279, #20224, #20917 ) ) ;
#2833=PLANE ( 'NONE',  #2938 ) ;
#2839=DIRECTION ( 'NONE',  ( 0.8660254037844352659, 0.5000000000000056621, 0.000000000000000000 ) ) ;
#2840=CARTESIAN_POINT ( 'NONE',  ( 211.7903592300262119, 6.147911733231966380, -2.561001429077395475 ) ) ;
#2849=VECTOR ( 'NONE', #20466, 1000.000000000000114 ) ;
#2852=CIRCLE ( 'NONE', #9254, 12.47473710546057823 ) ;
#2853=DIRECTION ( 'NONE',  ( -0.5000000000000054401, 0.8660254037844354880, -0.000000000000000000 ) ) ;
#2855=ORIENTED_EDGE ( 'NONE', *, *, #15536, .T. ) ;
#2861=VERTEX_POINT ( 'NONE', #15771 ) ;
#2863=CARTESIAN_POINT ( 'NONE',  ( 207.3946896431964149, 11.03307818039693267, -25.65046807331635392 ) ) ;
#2864=LINE ( 'NONE', #9299, #16071 ) ;
#2865=EDGE_CURVE ( 'NONE', #9778, #3962, #3769, .T. ) ;
#2868=DIRECTION ( 'NONE',  ( 0.6299240516454520655, 0.3636868207865263658, -0.6862416378687372642 ) ) ;
#2872=FACE_OUTER_BOUND ( 'NONE', #8945, .T. ) ;
#2885=CARTESIAN_POINT ( 'NONE',  ( 202.4269704670640238, 0.9995559342156025151, -23.72013913782470595 ) ) ;
#2886=ADVANCED_FACE ( 'NONE', ( #20823 ), #7893, .F. ) ;
#2892=CARTESIAN_POINT ( 'NONE',  ( 202.6969606483661721, 7.966816499295318543, -2.204078039983093706 ) ) ;
#2898=CARTESIAN_POINT ( 'NONE',  ( 194.6438684810882194, 7.795386067467640068, -19.29168348739290550 ) ) ;
#2901=DIRECTION ( 'NONE',  ( -0.8660254037844357100, -0.5000000000000051070, 0.000000000000000000 ) ) ;
#2903=VERTEX_POINT ( 'NONE', #12893 ) ;
#2904=EDGE_LOOP ( 'NONE', ( #10747, #1361, #2579, #19863, #12319, #1498 ) ) ;
#2907=ORIENTED_EDGE ( 'NONE', *, *, #8738, .T. ) ;
#2910=EDGE_LOOP ( 'NONE', ( #13458, #9217, #12056, #15316 ) ) ;
#2911=CONICAL_SURFACE ( 'NONE', #7961, 10.85470691220533190, 0.8171114040043576665 ) ;
#2913=CIRCLE ( 'NONE', #8303, 12.47473710546057823 ) ;
#2914=DIRECTION ( 'NONE',  ( 0.5000000000000051070, -0.8660254037844359321, 0.000000000000000000 ) ) ;
#2917=EDGE_CURVE ( 'NONE', #9370, #2041, #1340, .T. ) ;
#2922=CARTESIAN_POINT ( 'NONE',  ( 209.8577037357181894, 2.614299844655262106, -14.00000000000005507 ) ) ;
#2927=CARTESIAN_POINT ( 'NONE',  ( 217.4948448325154970, 10.21421812206089541, -7.132002368301439077 ) ) ;
#2930=DIRECTION ( 'NONE',  ( -0.8660254037844355990, -0.5000000000000055511, 0.000000000000000000 ) ) ;
#2931=CARTESIAN_POINT ( 'NONE',  ( 207.6064227804952225, 10.80129578285631453, -1.876704962899016893 ) ) ;
#2932=CARTESIAN_POINT ( 'NONE',  ( 209.5209968812125112, 4.837694770255529519, -27.13030671846411579 ) ) ;
#2933=EDGE_CURVE ( 'NONE', #12370, #15417, #20357, .T. ) ;
#2938=AXIS2_PLACEMENT_3D ( 'NONE', #14077, #5985, #20825 ) ;
#2939=CARTESIAN_POINT ( 'NONE',  ( 215.8574505745143597, 8.496048015791016539, -5.407152407594054466 ) ) ;
#2941=EDGE_CURVE ( 'NONE', #9185, #6444, #10528, .T. ) ;
#2944=CARTESIAN_POINT ( 'NONE',  ( 210.2598317367304332, 3.924419927273977482, -14.00000000000005507 ) ) ;
#2947=ORIENTED_EDGE ( 'NONE', *, *, #9251, .F. ) ;
#2952=EDGE_CURVE ( 'NONE', #17941, #6800, #12690, .T. ) ;
#2960=VERTEX_POINT ( 'NONE', #19250 ) ;
#2966=DIRECTION ( 'NONE',  ( -0.5000000000000058842, 0.8660254037844351549, 0.000000000000000000 ) ) ;
#2969=CARTESIAN_POINT ( 'NONE',  ( 205.0443405901917231, 9.676103521955074172, -13.34105989163307981 ) ) ;
#2971=DIRECTION ( 'NONE',  ( -0.4758887346169484722, -0.2747544890354094993, -0.8354878114129318245 ) ) ;
#2974=AXIS2_PLACEMENT_3D ( 'NONE', #4193, #1015, #15557 ) ;
#2975=DIRECTION ( 'NONE',  ( 0.8660254037844352659, 0.5000000000000056621, 0.000000000000000000 ) ) ;
#2978=VERTEX_POINT ( 'NONE', #17559 ) ;
#2981=ORIENTED_EDGE ( 'NONE', *, *, #19238, .T. ) ;
#2983=CARTESIAN_POINT ( 'NONE',  ( 200.9720064151970575, -0.09806717659808367182, -6.376588578941771779 ) ) ;
#2987=DIRECTION ( 'NONE',  ( -0.8426815769442658199, -0.4865224352899169546, 0.2306158707424407761 ) ) ;
#2996=DIRECTION ( 'NONE',  ( -0.8660254037844354880, -0.5000000000000055511, 0.000000000000000000 ) ) ;
#2999=LINE ( 'NONE', #9440, #4450 ) ;
#3000=LINE ( 'NONE', #20583, #267 ) ;
#3001=ORIENTED_EDGE ( 'NONE', *, *, #17168, .T. ) ;
#3011=ORIENTED_EDGE ( 'NONE', *, *, #18559, .T. ) ;
#3013=DIRECTION ( 'NONE',  ( -0.5000000000000054401, 0.8660254037844354880, -0.000000000000000000 ) ) ;
#3018=ORIENTED_EDGE ( 'NONE', *, *, #14425, .F. ) ;
#3019=CARTESIAN_POINT ( 'NONE',  ( 209.4102522745655506, 3.389308509292514149, -14.00000000000005507 ) ) ;
#3021=DIRECTION ( 'NONE',  ( -0.4330127018922105830, -0.2499999999999990563, 0.8660254037844432595 ) ) ;
#3024=B_SPLINE_CURVE_WITH_KNOTS ( 'NONE', 3,
 ( #17955, #6586, #12876, #19331 ),
 .UNSPECIFIED., .F., .F.,
 ( 4, 4 ),
 ( 3.993865398866640540E-07, 0.0006730501785945447674 ),
 .UNSPECIFIED. ) ;
#3026=EDGE_LOOP ( 'NONE', ( #16299, #19995, #7059, #14450, #19047, #8478 ) ) ;
#3028=ORIENTED_EDGE ( 'NONE', *, *, #9163, .F. ) ;
#3031=DIRECTION ( 'NONE',  ( -0.5000000000000054401, 0.8660254037844354880, -0.000000000000000000 ) ) ;
#3032=EDGE_CURVE ( 'NONE', #18332, #12370, #2087, .T. ) ;
#3041=CARTESIAN_POINT ( 'NONE',  ( 209.9458835816058411, 16.63000860489531263, -23.47937149798938350 ) ) ;
#3042=AXIS2_PLACEMENT_3D ( 'NONE', #14262, #19018, #14469 ) ;
#3043=EDGE_CURVE ( 'NONE', #8683, #15788, #18074, .T. ) ;
#3044=DIRECTION ( 'NONE',  ( 0.3430151393149146744, 0.1980398830195856108, 0.9182161068802695558 ) ) ;
#3054=CARTESIAN_POINT ( 'NONE',  ( 219.2795586678252562, 11.24462313530347757, -14.01558723443205068 ) ) ;
#3056=VECTOR ( 'NONE', #2798, 1000.000000000000114 ) ;
#3065=LINE ( 'NONE', #14424, #12813 ) ;
#3074=DIRECTION ( 'NONE',  ( -0.6946590618905486014, -0.4010615963775267523, -0.5971585917027842916 ) ) ;
#3075=VECTOR ( 'NONE', #13990, 1000.000000000000000 ) ;
#3076=DIRECTION ( 'NONE',  ( 0.5000000000000054401, -0.8660254037844354880, 0.000000000000000000 ) ) ;
#3081=VECTOR ( 'NONE', #4970, 999.9999999999998863 ) ;
#3085=CARTESIAN_POINT ( 'NONE',  ( 208.0983737146324870, 5.661548828456886895, -14.00000000000005507 ) ) ;
#3086=CONICAL_SURFACE ( 'NONE', #13240, 10.85470691220533190, 0.8171114040043576665 ) ;
#3088=VECTOR ( 'NONE', #4887, 1000.000000000000227 ) ;
#3090=DIRECTION ( 'NONE',  ( 0.5000000000000052180, -0.8660254037844355990, 0.000000000000000000 ) ) ;
#3096=DIRECTION ( 'NONE',  ( -0.5566703992264186995, -0.3213938048432738448, -0.7660444431189767922 ) ) ;
#3099=CARTESIAN_POINT ( 'NONE',  ( 199.2144802262915846, 21.04890371929339921, -14.00000000000005507 ) ) ;
#3100=FACE_OUTER_BOUND ( 'NONE', #18819, .T. ) ;
#3106=ORIENTED_EDGE ( 'NONE', *, *, #19854, .T. ) ;
#3107=AXIS2_PLACEMENT_3D ( 'NONE', #10271, #16760, #11998 ) ;
#3108=AXIS2_PLACEMENT_3D ( 'NONE', #5903, #6113, #18861 ) ;
#3109=LINE ( 'NONE', #20479, #8122 ) ;
#3134=EDGE_CURVE ( 'NONE', #9243, #18502, #19007, .T. ) ;
#3135=CIRCLE ( 'NONE', #15008, 6.960520131757800932 ) ;
#3136=ORIENTED_EDGE ( 'NONE', *, *, #7836, .F. ) ;
#3138=DIRECTION ( 'NONE',  ( -0.5000000000000051070, 0.8660254037844359321, -0.000000000000000000 ) ) ;
#3139=DIRECTION ( 'NONE',  ( -0.5000000000000051070, 0.8660254037844359321, -0.000000000000000000 ) ) ;
#3143=VERTEX_POINT ( 'NONE', #8302 ) ;
#3145=CARTESIAN_POINT ( 'NONE',  ( 197.6384891630574430, 5.400333206920676865, -21.69368824361338355 ) ) ;
#3146=VECTOR ( 'NONE', #10242, 1000.000000000000000 ) ;
#3147=ORIENTED_EDGE ( 'NONE', *, *, #16761, .T. ) ;
#3150=DIRECTION ( 'NONE',  ( -0.6946590618905487124, -0.4010615963775269188, -0.5971585917027841806 ) ) ;
#3153=ORIENTED_EDGE ( 'NONE', *, *, #14366, .T. ) ;
#3154=CARTESIAN_POINT ( 'NONE',  ( 195.4355411401220124, 3.951450668684652445, -16.79818413631467067 ) ) ;
#3163=CONICAL_SURFACE ( 'NONE', #9918, 10.85470691220533190, 0.8171114040043576665 ) ;
#3164=ORIENTED_EDGE ( 'NONE', *, *, #16286, .T. ) ;
#3165=EDGE_CURVE ( 'NONE', #16570, #5150, #15023, .T. ) ;
#3166=VERTEX_POINT ( 'NONE', #11610 ) ;
#3175=AXIS2_PLACEMENT_3D ( 'NONE', #5396, #19718, #10162 ) ;
#3178=DIRECTION ( 'NONE',  ( -0.4758887346169385357, -0.2747544890354034486, 0.8354878114129393740 ) ) ;
#3179=EDGE_CURVE ( 'NONE', #14733, #18877, #17665, .T. ) ;
#3180=ORIENTED_EDGE ( 'NONE', *, *, #9539, .T. ) ;
#3182=ORIENTED_EDGE ( 'NONE', *, *, #19141, .F. ) ;
#3185=CARTESIAN_POINT ( 'NONE',  ( 217.5096804110553137, 10.22278344732445809, -20.84195174293596153 ) ) ;
#3192=CARTESIAN_POINT ( 'NONE',  ( 212.6431940553267452, 14.06330361558336861, -5.407152407594061572 ) ) ;
#3195=VERTEX_POINT ( 'NONE', #20593 ) ;
#3197=DIRECTION ( 'NONE',  ( 0.5000000000000054401, -0.8660254037844354880, 0.000000000000000000 ) ) ;
#3199=LINE ( 'NONE', #17023, #2054 ) ;
#3202=VERTEX_POINT ( 'NONE', #14050 ) ;
#3204=DIRECTION ( 'NONE',  ( 0.8660254037844352659, 0.5000000000000056621, 0.000000000000000000 ) ) ;
#3207=LINE ( 'NONE', #9343, #20597 ) ;
#3212=ORIENTED_EDGE ( 'NONE', *, *, #3394, .T. ) ;
#3214=VERTEX_POINT ( 'NONE', #4066 ) ;
#3217=CARTESIAN_POINT ( 'NONE',  ( 195.3111273346253824, 3.525580966981323616, -11.13829696442576811 ) ) ;
#3220=CARTESIAN_POINT ( 'NONE',  ( 206.6380630506355089, 25.33491126127989546, -23.06309126349817618 ) ) ;
#3222=CARTESIAN_POINT ( 'NONE',  ( 214.2406644785986600, 14.98560359448187818, -21.57386172707946059 ) ) ;
#3223=VERTEX_POINT ( 'NONE', #2491 ) ;
#3224=CARTESIAN_POINT ( 'NONE',  ( 199.3859296228393134, 5.878169164976177363, -24.01557619556968248 ) ) ;
#3225=CARTESIAN_POINT ( 'NONE',  ( 198.7027818574981666, 10.13880079795527323, -24.25943249057081630 ) ) ;
#3231=CARTESIAN_POINT ( 'NONE',  ( 200.4318181982995952, 0.1052612498401872959, -21.90921222372413979 ) ) ;
#3233=VECTOR ( 'NONE', #7042, 999.9999999999998863 ) ;
#3235=CARTESIAN_POINT ( 'NONE',  ( 209.3053130134501885, 4.970768854950152971, -26.10149651730436915 ) ) ;
#3238=EDGE_LOOP ( 'NONE', ( #6683, #6477, #9346, #19511, #15256 ) ) ;
#3241=DIRECTION ( 'NONE',  ( -0.5000000000000049960, 0.8660254037844358210, -0.000000000000000000 ) ) ;
#3243=CARTESIAN_POINT ( 'NONE',  ( 211.5616548979095626, 6.788689316162965781, -2.044871543907030631 ) ) ;
#3244=VECTOR ( 'NONE', #10888, 1000.000000000000227 ) ;
#3247=ORIENTED_EDGE ( 'NONE', *, *, #9674, .T. ) ;
#3249=EDGE_LOOP ( 'NONE', ( #11950, #1982 ) ) ;
#3250=CARTESIAN_POINT ( 'NONE',  ( 201.7213150758130382, 0.3345463803147161741, -22.69908973750332848 ) ) ;
#3257=DIRECTION ( 'NONE',  ( -0.5000000000000049960, 0.8660254037844358210, -0.000000000000000000 ) ) ;
#3259=B_SPLINE_CURVE_WITH_KNOTS ( 'NONE', 3,
 ( #5092, #1933, #11574, #13069 ),
 .UNSPECIFIED., .F., .F.,
 ( 4, 4 ),
 ( 3.066983677782642140E-07, 0.0006729574904242660452 ),
 .UNSPECIFIED. ) ;
#3261=LINE ( 'NONE', #14635, #2404 ) ;
#3266=AXIS2_PLACEMENT_3D ( 'NONE', #18734, #3031, #9270 ) ;
#3267=DIRECTION ( 'NONE',  ( 0.7743856023693681534, 0.000000000000000000, 0.6327139470906508745 ) ) ;
#3278=ORIENTED_EDGE ( 'NONE', *, *, #9674, .F. ) ;
#3282=EDGE_CURVE ( 'NONE', #3474, #20283, #4285, .T. ) ;
#3291=VERTEX_POINT ( 'NONE', #16899 ) ;
#3299=CARTESIAN_POINT ( 'NONE',  ( 203.6269058993112253, 1.434739755226664970, -3.662783021451444299 ) ) ;
#3302=PLANE ( 'NONE',  #7457 ) ;
#3303=CARTESIAN_POINT ( 'NONE',  ( 213.4348361543090959, 18.64435631193540388, -18.06789442459603023 ) ) ;
#3304=CARTESIAN_POINT ( 'NONE',  ( 206.5868379288083645, 3.916477399883220745, -1.717498466822807490 ) ) ;
#3307=DIRECTION ( 'NONE',  ( 0.6634139481689348417, 0.3830222215594926705, -0.6427876096865408062 ) ) ;
#3314=ORIENTED_EDGE ( 'NONE', *, *, #11329, .T. ) ;
#3317=EDGE_CURVE ( 'NONE', #9778, #10058, #11277, .T. ) ;
#3320=ORIENTED_EDGE ( 'NONE', *, *, #10046, .F. ) ;
#3323=VERTEX_POINT ( 'NONE', #6476 ) ;
#3325=DIRECTION ( 'NONE',  ( -0.5000000000000054401, 0.8660254037844354880, -0.000000000000000000 ) ) ;
#3326=B_SPLINE_CURVE_WITH_KNOTS ( 'NONE', 3,
 ( #13757, #2523, #5359, #15469 ),
 .UNSPECIFIED., .F., .F.,
 ( 4, 4 ),
 ( 5.891946918164437828E-05, 0.0007315702612368541607 ),
 .UNSPECIFIED. ) ;
#3327=EDGE_CURVE ( 'NONE', #11827, #9243, #16062, .T. ) ;
#3328=( GEOMETRIC_REPRESENTATION_CONTEXT ( 3 ) GLOBAL_UNCERTAINTY_ASSIGNED_CONTEXT ( ( #18710 ) ) GLOBAL_UNIT_ASSIGNED_CONTEXT ( ( #20717, #12570, #12678 ) ) REPRESENTATION_CONTEXT ( 'NONE', 'WORKASPACE' ) );
#3335=DIRECTION ( 'NONE',  ( 0.5566703992264184775, 0.3213938048432735117, 0.7660444431189770143 ) ) ;
#3340=CARTESIAN_POINT ( 'NONE',  ( 216.7438708388689292, 9.007822994031293717, -21.66653917424403986 ) ) ;
#3342=DIRECTION ( 'NONE',  ( -0.4758887346169383692, -0.2747544890354036706, 0.8354878114129394850 ) ) ;
#3351=DIRECTION ( 'NONE',  ( 0.5000000000000049960, -0.8660254037844358210, 0.000000000000000000 ) ) ;
#3353=VERTEX_POINT ( 'NONE', #17428 ) ;
#3355=ORIENTED_EDGE ( 'NONE', *, *, #18858, .F. ) ;
#3356=CARTESIAN_POINT ( 'NONE',  ( 218.6234151596997322, 10.86579850426016769, -9.718744748713266546 ) ) ;
#3357=DIRECTION ( 'NONE',  ( -0.8660254037844355990, -0.5000000000000055511, 0.000000000000000000 ) ) ;
#3360=CARTESIAN_POINT ( 'NONE',  ( 205.5965122587965084, 9.994899983462953941, -14.00000000000005507 ) ) ;
#3361=CARTESIAN_POINT ( 'NONE',  ( 214.8451803045405484, 14.80357170752643370, -7.132002368301448847 ) ) ;
#3371=CARTESIAN_POINT ( 'NONE',  ( 209.6730417323522033, 12.34848537237979649, -24.85758746085098991 ) ) ;
#3372=FACE_OUTER_BOUND ( 'NONE', #9626, .T. ) ;
#3391=ADVANCED_FACE ( 'NONE', ( #10431 ), #13611, .T. ) ;
#3394=EDGE_CURVE ( 'NONE', #17439, #15921, #14064, .T. ) ;
#3397=B_SPLINE_CURVE_WITH_KNOTS ( 'NONE', 3,
 ( #2157, #10391, #19945, #5525 ),
 .UNSPECIFIED., .F., .F.,
 ( 4, 4 ),
 ( 3.426792995371261377E-07, 0.0008543284172840702635 ),
 .UNSPECIFIED. ) ;
#3400=CARTESIAN_POINT ( 'NONE',  ( 206.1084928877312734, 25.02916378517234364, -14.00000000000005329 ) ) ;
#3401=PLANE ( 'NONE',  #8166 ) ;
#3403=CARTESIAN_POINT ( 'NONE',  ( 208.0983737146324870, 5.661548828456886895, -14.00000000000005507 ) ) ;
#3408=CIRCLE ( 'NONE', #4757, 11.98469917212512215 ) ;
#3419=ORIENTED_EDGE ( 'NONE', *, *, #7177, .F. ) ;
#3420=DIRECTION ( 'NONE',  ( -0.2961981327260175267, -0.1710100716628331352, 0.9396926207859105373 ) ) ;
#3423=VECTOR ( 'NONE', #17452, 1000.000000000000114 ) ;
#3429=DIRECTION ( 'NONE',  ( 0.5000000000000049960, -0.8660254037844358210, 0.000000000000000000 ) ) ;
#3434=VERTEX_POINT ( 'NONE', #12044 ) ;
#3444=CARTESIAN_POINT ( 'NONE',  ( 202.6090205221545943, 8.270070825110927615, -2.522505859538386908 ) ) ;
#3447=ORIENTED_EDGE ( 'NONE', *, *, #799, .T. ) ;
#3449=ADVANCED_FACE ( 'NONE', ( #2293 ), #10541, .T. ) ;
#3453=FACE_OUTER_BOUND ( 'NONE', #1782, .T. ) ;
#3455=DIRECTION ( 'NONE',  ( -0.7500000000000013323, -0.4330127018922261817, -0.4999999999999918954 ) ) ;
#3462=ORIENTED_EDGE ( 'NONE', *, *, #19445, .T. ) ;
#3466=CARTESIAN_POINT ( 'NONE',  ( 192.5001239273000806, 6.557694572264193944, -12.41782726985248964 ) ) ;
#3468=ORIENTED_EDGE ( 'NONE', *, *, #11961, .T. ) ;
#3469=ORIENTED_EDGE ( 'NONE', *, *, #8484, .F. ) ;
#3474=VERTEX_POINT ( 'NONE', #698 ) ;
#3477=FACE_OUTER_BOUND ( 'NONE', #8979, .T. ) ;
#3478=AXIS2_PLACEMENT_3D ( 'NONE', #441, #2238, #2344 ) ;
#3482=LINE ( 'NONE', #14850, #4150 ) ;
#3484=CARTESIAN_POINT ( 'NONE',  ( 198.8157711536554189, -0.5701500946419610916, -8.415281845791808379 ) ) ;
#3485=B_SPLINE_CURVE_WITH_KNOTS ( 'NONE', 3,
 ( #11469, #15095, #9860, #550 ),
 .UNSPECIFIED., .F., .F.,
 ( 4, 4 ),
 ( 3.242053695260285290E-07, 0.0008543099433540281762 ),
 .UNSPECIFIED. ) ;
#3487=CARTESIAN_POINT ( 'NONE',  ( 204.7687975563032978, 2.094011210776437704, -3.125199447383417262 ) ) ;
#3489=ORIENTED_EDGE ( 'NONE', *, *, #14474, .T. ) ;
#3490=AXIS2_PLACEMENT_3D ( 'NONE', #19583, #2213, #7075 ) ;
#3492=ORIENTED_EDGE ( 'NONE', *, *, #14716, .T. ) ;
#3493=CARTESIAN_POINT ( 'NONE',  ( 207.8614403295549380, 4.652369439064019119, -1.545471579934808215 ) ) ;
#3501=DIRECTION ( 'NONE',  ( -0.5000000000000049960, 0.8660254037844358210, -0.000000000000000000 ) ) ;
#3502=AXIS2_PLACEMENT_3D ( 'NONE', #2944, #9383, #11309 ) ;
#3503=CARTESIAN_POINT ( 'NONE',  ( 205.8264633344831225, 9.596613037118636669, -14.00000000000005507 ) ) ;
#3506=B_SPLINE_CURVE_WITH_KNOTS ( 'NONE', 3,
 ( #1812, #4578, #12958, #20681 ),
 .UNSPECIFIED., .F., .F.,
 ( 4, 4 ),
 ( 0.0001303590654009653270, 0.0008030098574441160708 ),
 .UNSPECIFIED. ) ;
#3509=CARTESIAN_POINT ( 'NONE',  ( 193.1209940990829637, 6.916154133074862820, -9.448537646917497312 ) ) ;
#3512=LINE ( 'NONE', #14566, #10836 ) ;
#3514=CARTESIAN_POINT ( 'NONE',  ( 205.5965122587965084, 9.994899983462953941, -14.00000000000005507 ) ) ;
#3518=VERTEX_POINT ( 'NONE', #20914 ) ;
#3522=VERTEX_POINT ( 'NONE', #3224 ) ;
#3524=FACE_OUTER_BOUND ( 'NONE', #18859, .T. ) ;
#3536=ADVANCED_FACE ( 'NONE', ( #14175 ), #6190, .F. ) ;
#3538=ORIENTED_EDGE ( 'NONE', *, *, #17867, .T. ) ;
#3540=LINE ( 'NONE', #10093, #15312 ) ;
#3543=CONICAL_SURFACE ( 'NONE', #4569, 13.07248899748297433, 0.6693469023067423196 ) ;
#3545=LINE ( 'NONE', #13208, #5999 ) ;
#3556=DIRECTION ( 'NONE',  ( 0.5000000000000051070, -0.8660254037844359321, 0.000000000000000000 ) ) ;
#3561=EDGE_LOOP ( 'NONE', ( #6545, #20756, #9762, #7156 ) ) ;
#3562=ORIENTED_EDGE ( 'NONE', *, *, #1060, .F. ) ;
#3575=EDGE_CURVE ( 'NONE', #11395, #13335, #8443, .T. ) ;
#3581=LINE ( 'NONE', #17911, #12950 ) ;
#3584=EDGE_CURVE ( 'NONE', #20836, #17213, #4277, .T. ) ;
#3585=VERTEX_POINT ( 'NONE', #12884 ) ;
#3592=CARTESIAN_POINT ( 'NONE',  ( 198.5778388975847690, -0.9651341984995248646, -18.20125362229437016 ) ) ;
#3602=CARTESIAN_POINT ( 'NONE',  ( 197.7577498960094431, 5.469188423194260906, -6.376588578941773555 ) ) ;
#3603=CIRCLE ( 'NONE', #14475, 11.94520687646042667 ) ;
#3604=ORIENTED_EDGE ( 'NONE', *, *, #7207, .F. ) ;
#3606=DIRECTION ( 'NONE',  ( 0.8660254037844355990, 0.5000000000000054401, 0.000000000000000000 ) ) ;
#3608=LINE ( 'NONE', #19819, #6432 ) ;
#3610=CARTESIAN_POINT ( 'NONE',  ( 206.7336986317416176, 3.743653614488819503, -1.889534153981315523 ) ) ;
#3611=ORIENTED_EDGE ( 'NONE', *, *, #7381, .T. ) ;
#3612=DIRECTION ( 'NONE',  ( 0.5000000000000051070, -0.8660254037844359321, 0.000000000000000000 ) ) ;
#3620=ORIENTED_EDGE ( 'NONE', *, *, #15618, .F. ) ;
#3621=CARTESIAN_POINT ( 'NONE',  ( 212.9776690748797989, 18.38041077556222191, -19.29168348739316130 ) ) ;
#3622=ORIENTED_EDGE ( 'NONE', *, *, #14406, .T. ) ;
#3623=CARTESIAN_POINT ( 'NONE',  ( 204.7012550509497260, 2.055015527128745578, -24.96223045542551233 ) ) ;
#3628=CARTESIAN_POINT ( 'NONE',  ( 219.0871984830704662, 10.36074384021052985, -12.62839849932177394 ) ) ;
#3629=CARTESIAN_POINT ( 'NONE',  ( 208.0983737146324870, 5.661548828456886895, -14.00000000000005507 ) ) ;
#3631=ADVANCED_FACE ( 'NONE', ( #17341 ), #20642, .F. ) ;
#3633=ORIENTED_EDGE ( 'NONE', *, *, #10450, .F. ) ;
#3636=PLANE ( 'NONE',  #6095 ) ;
#3647=ORIENTED_EDGE ( 'NONE', *, *, #3923, .F. ) ;
#3656=CARTESIAN_POINT ( 'NONE',  ( 195.7290327299236594, 3.943881439888561324, -18.20503500338657688 ) ) ;
#3658=CARTESIAN_POINT ( 'NONE',  ( 205.5286554512480848, 3.047921609845726465, -25.78004855466121370 ) ) ;
#3659=AXIS2_PLACEMENT_3D ( 'NONE', #8047, #17727, #11456 ) ;
#3661=ORIENTED_EDGE ( 'NONE', *, *, #5748, .F. ) ;
#3665=VERTEX_POINT ( 'NONE', #2059 ) ;
#3666=ADVANCED_FACE ( 'NONE', ( #19638 ), #16471, .F. ) ;
#3675=CARTESIAN_POINT ( 'NONE',  ( 213.2304086110926278, 13.87128283563446018, -4.915515517929359035 ) ) ;
#3679=CARTESIAN_POINT ( 'NONE',  ( 207.0179943350028395, 10.81559304280891531, -15.68675928846492695 ) ) ;
#3683=ORIENTED_EDGE ( 'NONE', *, *, #6658, .T. ) ;
#3684=ORIENTED_EDGE ( 'NONE', *, *, #1917, .F. ) ;
#3686=EDGE_CURVE ( 'NONE', #10275, #15281, #5117, .T. ) ;
#3690=EDGE_LOOP ( 'NONE', ( #12816, #10856, #15069, #3180 ) ) ;
#3691=CARTESIAN_POINT ( 'NONE',  ( 203.1960812450809897, 12.73300840892584063, -2.187257959407754804 ) ) ;
#3692=DIRECTION ( 'NONE',  ( -0.5000000000000051070, 0.8660254037844359321, -0.000000000000000000 ) ) ;
#3693=ORIENTED_EDGE ( 'NONE', *, *, #5697, .T. ) ;
#3708=VECTOR ( 'NONE', #7049, 1000.000000000000114 ) ;
#3711=VERTEX_POINT ( 'NONE', #11704 ) ;
#3714=B_SPLINE_CURVE_WITH_KNOTS ( 'NONE', 3,
 ( #2737, #13871, #727, #5578 ),
 .UNSPECIFIED., .F., .F.,
 ( 4, 4 ),
 ( 3.220132087640094245E-07, 0.0008543077511937698446 ),
 .UNSPECIFIED. ) ;
#3718=ORIENTED_EDGE ( 'NONE', *, *, #3584, .F. ) ;
#3724=ORIENTED_EDGE ( 'NONE', *, *, #18207, .F. ) ;
#3727=DIRECTION ( 'NONE',  ( 0.8660254037844352659, 0.5000000000000056621, 0.000000000000000000 ) ) ;
#3733=FACE_OUTER_BOUND ( 'NONE', #5121, .T. ) ;
#3736=AXIS2_PLACEMENT_3D ( 'NONE', #17475, #4431, #12705 ) ;
#3748=VECTOR ( 'NONE', #14434, 1000.000000000000000 ) ;
#3766=DIRECTION ( 'NONE',  ( 0.5566703992264087075, 0.3213938048432681271, -0.7660444431189863401 ) ) ;
#3769=CIRCLE ( 'NONE', #16641, 11.98469917212512215 ) ;
#3775=AXIS2_PLACEMENT_3D ( 'NONE', #19400, #17816, #11345 ) ;
#3777=CIRCLE ( 'NONE', #8511, 12.47473710546057823 ) ;
#3786=CARTESIAN_POINT ( 'NONE',  ( 208.6876230897591142, 11.60254374963070667, -25.63868392505628435 ) ) ;
#3794=CARTESIAN_POINT ( 'NONE',  ( 215.2205796351215668, 15.55135787388338464, -18.06789442459603023 ) ) ;
#3797=ORIENTED_EDGE ( 'NONE', *, *, #6157, .F. ) ;
#3799=ORIENTED_EDGE ( 'NONE', *, *, #10826, .F. ) ;
#3801=CARTESIAN_POINT ( 'NONE',  ( 215.1325240088992246, 19.62451685178295691, -15.47241223420017953 ) ) ;
#3802=CARTESIAN_POINT ( 'NONE',  ( 217.4675698996929896, 9.683250065417357888, -20.66514661561436483 ) ) ;
#3813=ADVANCED_FACE ( 'NONE', ( #15116 ), #12021, .T. ) ;
#3817=FACE_OUTER_BOUND ( 'NONE', #15287, .T. ) ;
#3826=ADVANCED_FACE ( 'NONE', ( #10296 ), #16787, .T. ) ;
#3827=ORIENTED_EDGE ( 'NONE', *, *, #16546, .F. ) ;
#3829=FACE_OUTER_BOUND ( 'NONE', #1692, .T. ) ;
#3830=EDGE_CURVE ( 'NONE', #688, #1818, #13718, .T. ) ;
#3832=CIRCLE ( 'NONE', #4525, 12.47473710546057823 ) ;
#3833=DIRECTION ( 'NONE',  ( -0.000000000000000000, 0.000000000000000000, 1.000000000000000000 ) ) ;
#3838=LINE ( 'NONE', #10078, #5063 ) ;
#3842=DIRECTION ( 'NONE',  ( 0.8296432542242749841, 0.4789947561577487245, -0.2868032327110942581 ) ) ;
#3844=DIRECTION ( 'NONE',  ( 0.5000000000000049960, -0.8660254037844358210, 0.000000000000000000 ) ) ;
#3845=CARTESIAN_POINT ( 'NONE',  ( 208.2224579217690632, 4.087982952467670295, -25.92587471718749725 ) ) ;
#3848=AXIS2_PLACEMENT_3D ( 'NONE', #4030, #12321, #9309 ) ;
#3852=DIRECTION ( 'NONE',  ( 0.5000000000000054401, -0.8660254037844354880, -1.665334536937734318E-16 ) ) ;
#3854=ORIENTED_EDGE ( 'NONE', *, *, #5139, .T. ) ;
#3859=CARTESIAN_POINT ( 'NONE',  ( 205.7420593526227890, 14.20292955466599238, -26.96550585544247269 ) ) ;
#3863=CARTESIAN_POINT ( 'NONE',  ( 198.4834855446717938, -1.277216147272815849, -16.79062062844341696 ) ) ;
#3864=ORIENTED_EDGE ( 'NONE', *, *, #1632, .F. ) ;
#3866=DIRECTION ( 'NONE',  ( 0.5000000000000054401, -0.8660254037844354880, 0.000000000000000000 ) ) ;
#3867=ORIENTED_EDGE ( 'NONE', *, *, #12518, .F. ) ;
#3874=ORIENTED_EDGE ( 'NONE', *, *, #10282, .F. ) ;
#3878=VECTOR ( 'NONE', #12139, 1000.000000000000114 ) ;
#3882=VERTEX_POINT ( 'NONE', #4688 ) ;
#3883=ORIENTED_EDGE ( 'NONE', *, *, #17795, .F. ) ;
#3887=ORIENTED_EDGE ( 'NONE', *, *, #4751, .T. ) ;
#3888=CARTESIAN_POINT ( 'NONE',  ( 204.5209968812124544, 13.49794880809988484, -27.13030671846411579 ) ) ;
#3892=CARTESIAN_POINT ( 'NONE',  ( 197.4890135470689643, -2.108974046597433816, -15.47241223419981715 ) ) ;
#3896=CARTESIAN_POINT ( 'NONE',  ( 209.9028093415542173, 12.48114176340364700, -14.15605348658545282 ) ) ;
#3900=VERTEX_POINT ( 'NONE', #9444 ) ;
#3904=ORIENTED_EDGE ( 'NONE', *, *, #18283, .T. ) ;
#3906=ORIENTED_EDGE ( 'NONE', *, *, #1187, .T. ) ;
#3907=CARTESIAN_POINT ( 'NONE',  ( 199.2144802262915846, 21.04890371929339921, -14.00000000000005507 ) ) ;
#3909=CARTESIAN_POINT ( 'NONE',  ( 200.1138010445123143, -0.5935522783828972582, -22.49869731917958404 ) ) ;
#3912=CARTESIAN_POINT ( 'NONE',  ( 216.1231765438266166, 15.71844586073754790, -16.84511136304323387 ) ) ;
#3913=ORIENTED_EDGE ( 'NONE', *, *, #5748, .T. ) ;
#3916=EDGE_CURVE ( 'NONE', #4803, #10151, #12448, .T. ) ;
#3922=AXIS2_PLACEMENT_3D ( 'NONE', #2521, #4523, #14297 ) ;
#3923=EDGE_CURVE ( 'NONE', #19176, #9963, #4379, .T. ) ;
#3924=ORIENTED_EDGE ( 'NONE', *, *, #2788, .F. ) ;
#3925=CARTESIAN_POINT ( 'NONE',  ( 215.8800731390675764, 9.281929250168950318, -4.915515517929356371 ) ) ;
#3926=FACE_OUTER_BOUND ( 'NONE', #15077, .T. ) ;
#3928=AXIS2_PLACEMENT_3D ( 'NONE', #9114, #12328, #18784 ) ;
#3935=DIRECTION ( 'NONE',  ( 0.8660254037844355990, 0.5000000000000054401, -3.198355172551227375E-14 ) ) ;
#3936=CARTESIAN_POINT ( 'NONE',  ( 213.7787453705537075, 18.84291239051101741, -11.24974199967302013 ) ) ;
#3942=CONICAL_SURFACE ( 'NONE', #9682, 10.85470691220533190, 0.8171114040043576665 ) ;
#3945=CARTESIAN_POINT ( 'NONE',  ( 200.4559313511114453, 7.026984212619883152, -3.762296834228767928 ) ) ;
#3948=EDGE_LOOP ( 'NONE', ( #1103, #12176, #13988, #2172 ) ) ;
#3952=CARTESIAN_POINT ( 'NONE',  ( 210.5718816476998256, 5.444423373074280370, -2.341985411377013548 ) ) ;
#3955=DIRECTION ( 'NONE',  ( -0.5000000000000049960, 0.8660254037844357100, -0.000000000000000000 ) ) ;
#3961=ORIENTED_EDGE ( 'NONE', *, *, #8809, .F. ) ;
#3962=VERTEX_POINT ( 'NONE', #6057 ) ;
#3965=DIRECTION ( 'NONE',  ( 0.5000000000000054401, -0.8660254037844354880, 0.000000000000000000 ) ) ;
#3968=CARTESIAN_POINT ( 'NONE',  ( 206.2818991689553627, 10.21359839635873357, -26.12768996730768478 ) ) ;
#3972=EDGE_CURVE ( 'NONE', #17245, #11939, #11865, .T. ) ;
#3973=VERTEX_POINT ( 'NONE', #17630 ) ;
#3976=CARTESIAN_POINT ( 'NONE',  ( 207.8527399996651184, 15.42153159440924881, -3.125199447383529172 ) ) ;
#3979=CARTESIAN_POINT ( 'NONE',  ( 205.0662616026534693, 10.91332106064940888, -14.00000000000005507 ) ) ;
#3981=EDGE_CURVE ( 'NONE', #6334, #17905, #20928, .T. ) ;
#3986=EDGE_LOOP ( 'NONE', ( #1468, #20086, #13542, #19228 ) ) ;
#3989=PLANE ( 'NONE',  #367 ) ;
#3990=EDGE_CURVE ( 'NONE', #600, #7107, #3109, .T. ) ;
#3992=B_SPLINE_CURVE_WITH_KNOTS ( 'NONE', 3,
 ( #3145, #4725, #7900, #20625 ),
 .UNSPECIFIED., .F., .F.,
 ( 4, 4 ),
 ( 6.424236652724635136E-05, 0.0007368931585819213240 ),
 .UNSPECIFIED. ) ;
#3996=CARTESIAN_POINT ( 'NONE',  ( 195.4998201364199417, 4.165572068683992768, -11.22353489230383339 ) ) ;
#4001=CIRCLE ( 'NONE', #17892, 11.94520687646042667 ) ;
#4004=LINE ( 'NONE', #5792, #2138 ) ;
#4013=ORIENTED_EDGE ( 'NONE', *, *, #19159, .F. ) ;
#4016=EDGE_LOOP ( 'NONE', ( #13423, #14880 ) ) ;
#4020=LINE ( 'NONE', #1063, #958 ) ;
#4022=EDGE_CURVE ( 'NONE', #17056, #4395, #3259, .T. ) ;
#4029=DIRECTION ( 'NONE',  ( 0.8660254037844352659, 0.5000000000000056621, 0.000000000000000000 ) ) ;
#4030=CARTESIAN_POINT ( 'NONE',  ( 209.3577037357181894, 3.480325248439694263, -14.00000000000005507 ) ) ;
#4031=CARTESIAN_POINT ( 'NONE',  ( 201.5598379337182848, 7.133275713455735634, -25.46066938576250394 ) ) ;
#4034=EDGE_CURVE ( 'NONE', #10335, #19279, #17840, .T. ) ;
#4036=DIRECTION ( 'NONE',  ( -0.8660254037844355990, -0.5000000000000055511, 0.000000000000000000 ) ) ;
#4038=EDGE_CURVE ( 'NONE', #15921, #5032, #3512, .T. ) ;
#4039=DIRECTION ( 'NONE',  ( 0.9885408208161388099, 0.000000000000000000, 0.1509537862398780406 ) ) ;
#4040=VECTOR ( 'NONE', #19153, 1000.000000000000000 ) ;
#4041=ORIENTED_EDGE ( 'NONE', *, *, #945, .T. ) ;
#4045=CARTESIAN_POINT ( 'NONE',  ( 205.8264633344831225, 9.596613037118636669, -14.00000000000005507 ) ) ;
#4050=B_SPLINE_CURVE_WITH_KNOTS ( 'NONE', 3,
 ( #5422, #18383, #18588, #10514 ),
 .UNSPECIFIED., .F., .F.,
 ( 4, 4 ),
 ( 6.863716774068141194E-05, 0.0007412879597948096892 ),
 .UNSPECIFIED. ) ;
#4056=CARTESIAN_POINT ( 'NONE',  ( 208.0983737146324870, 5.661548828456886895, -14.00000000000005507 ) ) ;
#4064=VERTEX_POINT ( 'NONE', #5192 ) ;
#4066=CARTESIAN_POINT ( 'NONE',  ( 201.5199827852405861, 7.641314594545947969, -24.85758746085086557 ) ) ;
#4067=EDGE_LOOP ( 'NONE', ( #5245, #6014, #15021, #5942 ) ) ;
#4069=B_SPLINE_CURVE_WITH_KNOTS ( 'NONE', 3,
 ( #15194, #17181, #11996, #18454 ),
 .UNSPECIFIED., .F., .F.,
 ( 4, 4 ),
 ( 5.972954429729013304E-06, 0.0003733324143565315990 ),
 .UNSPECIFIED. ) ;
#4070=EDGE_CURVE ( 'NONE', #688, #14131, #1717, .T. ) ;
#4076=ORIENTED_EDGE ( 'NONE', *, *, #19588, .F. ) ;
#4077=VERTEX_POINT ( 'NONE', #16446 ) ;
#4080=LINE ( 'NONE', #8948, #3233 ) ;
#4081=AXIS2_PLACEMENT_3D ( 'NONE', #19989, #15461, #2621 ) ;
#4083=EDGE_LOOP ( 'NONE', ( #14996, #1298, #1256, #6821, #6211, #6184 ) ) ;
#4090=ORIENTED_EDGE ( 'NONE', *, *, #455, .T. ) ;
#4095=VECTOR ( 'NONE', #6838, 1000.000000000000227 ) ;
#4096=VECTOR ( 'NONE', #20511, 1000.000000000000227 ) ;
#4097=ORIENTED_EDGE ( 'NONE', *, *, #12346, .F. ) ;
#4105=CARTESIAN_POINT ( 'NONE',  ( 203.2663706161054620, 1.741790851292542408, -3.346771071759890859 ) ) ;
#4107=DIRECTION ( 'NONE',  ( -0.5000000000000051070, 0.8660254037844359321, -0.000000000000000000 ) ) ;
#4108=ADVANCED_FACE ( 'NONE', ( #11466 ), #9151, .T. ) ;
#4109=AXIS2_PLACEMENT_3D ( 'NONE', #14395, #6395, #6197 ) ;
#4115=CARTESIAN_POINT ( 'NONE',  ( 205.8264633344831225, 9.596613037118636669, -14.00000000000005507 ) ) ;
#4119=ORIENTED_EDGE ( 'NONE', *, *, #2027, .T. ) ;
#4120=FACE_OUTER_BOUND ( 'NONE', #7915, .T. ) ;
#4123=ADVANCED_FACE ( 'NONE', ( #6467 ), #18659, .T. ) ;
#4128=LINE ( 'NONE', #20027, #5591 ) ;
#4129=ORIENTED_EDGE ( 'NONE', *, *, #10460, .F. ) ;
#4131=LINE ( 'NONE', #15182, #12779 ) ;
#4133=AXIS2_PLACEMENT_3D ( 'NONE', #4396, #18716, #4295 ) ;
#4135=VECTOR ( 'NONE', #1377, 1000.000000000000227 ) ;
#4146=ORIENTED_EDGE ( 'NONE', *, *, #16467, .F. ) ;
#4147=CIRCLE ( 'NONE', #17315, 4.999999999999977796 ) ;
#4150=VECTOR ( 'NONE', #9927, 1000.000000000000000 ) ;
#4152=EDGE_CURVE ( 'NONE', #18151, #18856, #3408, .T. ) ;
#4161=AXIS2_PLACEMENT_3D ( 'NONE', #6643, #7491, #14088 ) ;
#4173=DIRECTION ( 'NONE',  ( -0.8660254037844354880, -0.5000000000000055511, 0.000000000000000000 ) ) ;
#4174=FACE_OUTER_BOUND ( 'NONE', #4016, .T. ) ;
#4175=VECTOR ( 'NONE', #6256, 1000.000000000000114 ) ;
#4179=ORIENTED_EDGE ( 'NONE', *, *, #16223, .T. ) ;
#4183=DIRECTION ( 'NONE',  ( 0.5000000000000049960, -0.8660254037844358210, 0.000000000000000000 ) ) ;
#4185=FACE_OUTER_BOUND ( 'NONE', #10949, .T. ) ;
#4187=EDGE_CURVE ( 'NONE', #15382, #11167, #15198, .T. ) ;
#4189=CIRCLE ( 'NONE', #17743, 11.94520687646042667 ) ;
#4193=CARTESIAN_POINT ( 'NONE',  ( 199.2144802262915846, 21.04890371929339921, -14.00000000000005507 ) ) ;
#4200=EDGE_LOOP ( 'NONE', ( #12514, #4332, #15081, #14287 ) ) ;
#4203=CARTESIAN_POINT ( 'NONE',  ( 210.3388300726135753, 6.082691074106562290, -26.28791492288521425 ) ) ;
#4206=AXIS2_PLACEMENT_3D ( 'NONE', #2655, #8795, #1275 ) ;
#4208=EDGE_CURVE ( 'NONE', #11395, #16570, #14097, .T. ) ;
#4214=ADVANCED_FACE ( 'NONE', ( #20635 ), #20435, .T. ) ;
#4219=EDGE_CURVE ( 'NONE', #5521, #7807, #15620, .T. ) ;
#4228=VERTEX_POINT ( 'NONE', #18854 ) ;
#4230=CARTESIAN_POINT ( 'NONE',  ( 214.1487250227890797, 14.93252232492107545, -20.52105855319947025 ) ) ;
#4234=ORIENTED_EDGE ( 'NONE', *, *, #744, .T. ) ;
#4235=EDGE_CURVE ( 'NONE', #835, #5696, #15155, .T. ) ;
#4237=ORIENTED_EDGE ( 'NONE', *, *, #3032, .T. ) ;
#4243=CARTESIAN_POINT ( 'NONE',  ( 214.7133389289038803, 15.25850231560466597, -7.412933984336929960 ) ) ;
#4244=EDGE_CURVE ( 'NONE', #16739, #18930, #6767, .T. ) ;
#4246=PLANE ( 'NONE',  #9657 ) ;
#4249=DIRECTION ( 'NONE',  ( -0.5000000000000049960, 0.8660254037844358210, -0.000000000000000000 ) ) ;
#4252=ADVANCED_FACE ( 'NONE', ( #10893 ), #7707, .F. ) ;
#4254=ORIENTED_EDGE ( 'NONE', *, *, #13413, .T. ) ;
#4255=VECTOR ( 'NONE', #20361, 1000.000000000000114 ) ;
#4262=EDGE_LOOP ( 'NONE', ( #5568, #15501, #6738, #5039, #7228, #16402 ) ) ;
#4265=CARTESIAN_POINT ( 'NONE',  ( 196.7914626300884322, 9.035300127502988943, -22.62267072728657169 ) ) ;
#4267=CARTESIAN_POINT ( 'NONE',  ( 199.2144802262915846, 21.04890371929339921, -14.00000000000005507 ) ) ;
#4268=AXIS2_PLACEMENT_3D ( 'NONE', #20053, #16981, #5513 ) ;
#4269=FACE_OUTER_BOUND ( 'NONE', #19539, .T. ) ;
#4275=DIRECTION ( 'NONE',  ( -0.8660254037844357100, -0.5000000000000051070, 0.000000000000000000 ) ) ;
#4276=LINE ( 'NONE', #7548, #15935 ) ;
#4277=B_SPLINE_CURVE_WITH_KNOTS ( 'NONE', 3,
 ( #1228, #15762, #15970, #9467 ),
 .UNSPECIFIED., .F., .F.,
 ( 4, 4 ),
 ( 1.412303226746373230E-05, 0.0006867738243255644111 ),
 .UNSPECIFIED. ) ;
#4283=AXIS2_PLACEMENT_3D ( 'NONE', #9401, #17586, #19073 ) ;
#4285=LINE ( 'NONE', #10736, #743 ) ;
#4295=DIRECTION ( 'NONE',  ( -0.8660254037844355990, -0.5000000000000054401, 1.237624392856779246E-14 ) ) ;
#4296=ORIENTED_EDGE ( 'NONE', *, *, #10953, .T. ) ;
#4302=LINE ( 'NONE', #10433, #1581 ) ;
#4306=ORIENTED_EDGE ( 'NONE', *, *, #8567, .F. ) ;
#4308=ORIENTED_EDGE ( 'NONE', *, *, #13828, .T. ) ;
#4309=DIRECTION ( 'NONE',  ( 0.5000000000000051070, -0.8660254037844359321, 0.000000000000000000 ) ) ;
#4310=CARTESIAN_POINT ( 'NONE',  ( 207.7157532681331134, 10.68739508888871548, -1.717498466822861225 ) ) ;
#4311=DIRECTION ( 'NONE',  ( -1.000000000000000000, 0.000000000000000000, 0.000000000000000000 ) ) ;
#4313=AXIS2_PLACEMENT_3D ( 'NONE', #12928, #14843, #3267 ) ;
#4318=B_SPLINE_CURVE_WITH_KNOTS ( 'NONE', 3,
 ( #20846, #12610, #9508, #6321 ),
 .UNSPECIFIED., .F., .F.,
 ( 4, 4 ),
 ( 4.713673267783319110E-06, 0.0006773644653211034414 ),
 .UNSPECIFIED. ) ;
#4319=FACE_OUTER_BOUND ( 'NONE', #3948, .T. ) ;
#4321=CARTESIAN_POINT ( 'NONE',  ( 195.6791760372415183, 3.738073984511642855, -9.718744748712971671 ) ) ;
#4324=EDGE_CURVE ( 'NONE', #18930, #5590, #10781, .T. ) ;
#4327=ORIENTED_EDGE ( 'NONE', *, *, #12667, .T. ) ;
#4330=CARTESIAN_POINT ( 'NONE',  ( 206.6184255029011183, 25.32357351780921917, -4.915515517929356371 ) ) ;
#4332=ORIENTED_EDGE ( 'NONE', *, *, #11381, .T. ) ;
#4335=DIRECTION ( 'NONE',  ( 0.1997192025788214753, 0.1153079353712215399, 0.9730448705798235842 ) ) ;
#4342=EDGE_CURVE ( 'NONE', #18395, #12920, #19319, .T. ) ;
#4343=DIRECTION ( 'NONE',  ( 0.5000000000000052180, -0.8660254037844355990, 2.220446049250312588E-16 ) ) ;
#4348=CARTESIAN_POINT ( 'NONE',  ( 199.2144802262915846, 21.04890371929339921, -14.00000000000005507 ) ) ;
#4353=CARTESIAN_POINT ( 'NONE',  ( 219.8858643771923198, 10.82185380917437278, -17.08769543353844256 ) ) ;
#4354=ADVANCED_FACE ( 'NONE', ( #15790 ), #14206, .F. ) ;
#4355=VERTEX_POINT ( 'NONE', #4738 ) ;
#4361=CARTESIAN_POINT ( 'NONE',  ( 197.6384891630574430, 5.400333206920676865, -21.69368824361338355 ) ) ;
#4362=EDGE_CURVE ( 'NONE', #1433, #18162, #14606, .T. ) ;
#4368=DIRECTION ( 'NONE',  ( -0.2961981327260292396, -0.1710100716628399076, -0.9396926207859056523 ) ) ;
#4371=VECTOR ( 'NONE', #13686, 1000.000000000000114 ) ;
#4372=DIRECTION ( 'NONE',  ( -0.5000000000000027756, 0.8660254037844372643, -0.000000000000000000 ) ) ;
#4374=CARTESIAN_POINT ( 'NONE',  ( 219.1556129512320013, 10.40024295182009517, -13.98474561060134747 ) ) ;
#4375=DIRECTION ( 'NONE',  ( 0.5000000000000052180, -0.8660254037844355990, 1.665334536937734564E-16 ) ) ;
#4377=LINE ( 'NONE', #4487, #613 ) ;
#4379=LINE ( 'NONE', #7757, #14917 ) ;
#4381=EDGE_CURVE ( 'NONE', #16338, #12547, #16101, .T. ) ;
#4382=ADVANCED_FACE ( 'NONE', ( #6416 ), #14411, .F. ) ;
#4386=ORIENTED_EDGE ( 'NONE', *, *, #8580, .T. ) ;
#4390=EDGE_LOOP ( 'NONE', ( #7986, #1781, #9138, #1628 ) ) ;
#4394=VECTOR ( 'NONE', #19723, 1000.000000000000000 ) ;
#4395=VERTEX_POINT ( 'NONE', #5149 ) ;
#4396=CARTESIAN_POINT ( 'NONE',  ( 208.4761278624580711, 5.007259451653140125, -14.00000000000005507 ) ) ;
#4397=EDGE_LOOP ( 'NONE', ( #12714, #15387, #15546, #15107, #13210, #19022 ) ) ;
#4398=CARTESIAN_POINT ( 'NONE',  ( 198.0735972701637024, -1.389238810292188875, -14.00000000000005507 ) ) ;
#4399=CARTESIAN_POINT ( 'NONE',  ( 195.2174643819972744, 4.002553897860817500, -13.98704593443225797 ) ) ;
#4407=ORIENTED_EDGE ( 'NONE', *, *, #8738, .F. ) ;
#4408=EDGE_LOOP ( 'NONE', ( #15426, #14543, #7872, #11973 ) ) ;
#4409=EDGE_CURVE ( 'NONE', #1689, #20898, #2058, .T. ) ;
#4410=DIRECTION ( 'NONE',  ( -0.5000000000000054401, 0.8660254037844354880, -0.000000000000000000 ) ) ;
#4412=CARTESIAN_POINT ( 'NONE',  ( 205.0662616026534693, 10.91332106064940888, -14.00000000000005507 ) ) ;
#4420=EDGE_CURVE ( 'NONE', #5696, #13143, #13225, .T. ) ;
#4421=CARTESIAN_POINT ( 'NONE',  ( 213.9443517339557843, 7.649119109015196649, -24.50020013040646560 ) ) ;
#4423=DIRECTION ( 'NONE',  ( -0.8660254037844369313, -0.5000000000000027756, 0.000000000000000000 ) ) ;
#4426=ORIENTED_EDGE ( 'NONE', *, *, #1906, .T. ) ;
#4427=ORIENTED_EDGE ( 'NONE', *, *, #2952, .F. ) ;
#4431=DIRECTION ( 'NONE',  ( -0.5000000000000049960, 0.8660254037844357100, -0.000000000000000000 ) ) ;
#4433=VECTOR ( 'NONE', #14568, 1000.000000000000114 ) ;
#4435=ORIENTED_EDGE ( 'NONE', *, *, #19079, .F. ) ;
#4438=CARTESIAN_POINT ( 'NONE',  ( 207.3877668936371492, 11.02908132907535332, -2.195132782454303655 ) ) ;
#4442=EDGE_LOOP ( 'NONE', ( #20192, #20407, #4526, #18482, #344, #15073 ) ) ;
#4450=VECTOR ( 'NONE', #12967, 1000.000000000000227 ) ;
#4456=CARTESIAN_POINT ( 'NONE',  ( 211.6640881527417832, 17.62201447656351405, -23.53124788243930965 ) ) ;
#4457=DIRECTION ( 'NONE',  ( 0.5000000000000051070, -0.8660254037844359321, 0.000000000000000000 ) ) ;
#4463=VERTEX_POINT ( 'NONE', #11416 ) ;
#4465=ADVANCED_FACE ( 'NONE', ( #19675 ), #13580, .T. ) ;
#4468=EDGE_CURVE ( 'NONE', #1190, #3202, #9031, .T. ) ;
#4471=VECTOR ( 'NONE', #14316, 1000.000000000000114 ) ;
#4472=VECTOR ( 'NONE', #17107, 1000.000000000000227 ) ;
#4480=VECTOR ( 'NONE', #13848, 1000.000000000000114 ) ;
#4482=CARTESIAN_POINT ( 'NONE',  ( 199.2231352798572743, 21.03391272677540513, -14.00000000000005507 ) ) ;
#4484=AXIS2_PLACEMENT_3D ( 'NONE', #17049, #13662, #18636 ) ;
#4487=CARTESIAN_POINT ( 'NONE',  ( 205.5254235590769838, 9.953856903543536916, -15.84972809015757278 ) ) ;
#4490=ADVANCED_FACE ( 'NONE', ( #16607 ), #3989, .F. ) ;
#4491=DIRECTION ( 'NONE',  ( 0.4661719196087402706, -0.8846941513134933821, 4.730853538934608585E-18 ) ) ;
#4493=CARTESIAN_POINT ( 'NONE',  ( 211.5944766886066191, 17.58182427900635503, -4.392917125964958203 ) ) ;
#4495=ORIENTED_EDGE ( 'NONE', *, *, #5131, .F. ) ;
#4503=LINE ( 'NONE', #15847, #20517 ) ;
#4504=EDGE_CURVE ( 'NONE', #9864, #1927, #14954, .T. ) ;
#4506=DIRECTION ( 'NONE',  ( 0.5000000000000054401, -0.8660254037844354880, 0.000000000000000000 ) ) ;
#4507=DIRECTION ( 'NONE',  ( -0.8660254037844354880, -0.5000000000000055511, 0.000000000000000000 ) ) ;
#4513=DIRECTION ( 'NONE',  ( 0.8660254037844352659, 0.5000000000000056621, 0.000000000000000000 ) ) ;
#4515=ORIENTED_EDGE ( 'NONE', *, *, #1997, .T. ) ;
#4516=DIRECTION ( 'NONE',  ( -0.8660254037844357100, -0.5000000000000051070, 0.000000000000000000 ) ) ;
#4520=DIRECTION ( 'NONE',  ( 0.8660254037844352659, 0.5000000000000056621, 0.000000000000000000 ) ) ;
#4522=CARTESIAN_POINT ( 'NONE',  ( 218.9852377222535154, 11.07469685814948157, -16.89203719259520753 ) ) ;
#4523=DIRECTION ( 'NONE',  ( -0.5000000000000054401, 0.8660254037844354880, -0.000000000000000000 ) ) ;
#4525=AXIS2_PLACEMENT_3D ( 'NONE', #14563, #14463, #7862 ) ;
#4526=ORIENTED_EDGE ( 'NONE', *, *, #16699, .F. ) ;
#4529=CARTESIAN_POINT ( 'NONE',  ( 211.2164883113428857, 12.70854540844746872, -3.188775577416895324 ) ) ;
#4532=CARTESIAN_POINT ( 'NONE',  ( 193.6336827526812101, 7.212155065240265728, -15.39542905462715083 ) ) ;
#4534=EDGE_LOOP ( 'NONE', ( #1316, #5052, #8100, #12206, #17872, #17188 ) ) ;
#4535=VERTEX_POINT ( 'NONE', #13333 ) ;
#4540=ORIENTED_EDGE ( 'NONE', *, *, #2575, .T. ) ;
#4541=ORIENTED_EDGE ( 'NONE', *, *, #5697, .F. ) ;
#4557=CARTESIAN_POINT ( 'NONE',  ( 195.4194262334934535, 4.119156627188157671, -15.39542905462715083 ) ) ;
#4562=LINE ( 'NONE', #7932, #20108 ) ;
#4567=VERTEX_POINT ( 'NONE', #1984 ) ;
#4569=AXIS2_PLACEMENT_3D ( 'NONE', #19235, #3013, #19428 ) ;
#4572=CARTESIAN_POINT ( 'NONE',  ( 201.0721825858487364, 0.7325896531374328502, -4.915515517929136990 ) ) ;
#4576=ORIENTED_EDGE ( 'NONE', *, *, #4034, .F. ) ;
#4577=DIRECTION ( 'NONE',  ( 0.4758887346169485832, 0.2747544890354092773, 0.8354878114129317135 ) ) ;
#4578=CARTESIAN_POINT ( 'NONE',  ( 215.5602275462317436, 15.57044378260907180, -9.848357292554322129 ) ) ;
#4581=EDGE_CURVE ( 'NONE', #18042, #1689, #6725, .T. ) ;
#4583=CARTESIAN_POINT ( 'NONE',  ( 208.0983737146324870, 5.661548828456886895, -14.00000000000005507 ) ) ;
#4586=CARTESIAN_POINT ( 'NONE',  ( 201.9688168050318211, 0.4774415703040005288, -3.480441514389559288 ) ) ;
#4587=CIRCLE ( 'NONE', #17116, 12.47473710546057823 ) ;
#4589=VERTEX_POINT ( 'NONE', #7056 ) ;
#4593=DIRECTION ( 'NONE',  ( -0.5000000000000051070, 0.8660254037844359321, -0.000000000000000000 ) ) ;
#4600=VECTOR ( 'NONE', #17720, 1000.000000000000227 ) ;
#4601=PLANE ( 'NONE',  #8718 ) ;
#4602=CARTESIAN_POINT ( 'NONE',  ( 205.0662616026534693, 10.91332106064940888, -14.00000000000005507 ) ) ;
#4607=FACE_OUTER_BOUND ( 'NONE', #4083, .T. ) ;
#4609=AXIS2_PLACEMENT_3D ( 'NONE', #15774, #14079, #20313 ) ;
#4610=ADVANCED_FACE ( 'NONE', ( #16719 ), #2198, .F. ) ;
#4614=AXIS2_PLACEMENT_3D ( 'NONE', #14941, #8018, #405 ) ;
#4615=ORIENTED_EDGE ( 'NONE', *, *, #20040, .F. ) ;
#4616=AXIS2_PLACEMENT_3D ( 'NONE', #1384, #3076, #1801 ) ;
#4619=DIRECTION ( 'NONE',  ( -0.5000000000000052180, 0.8660254037844355990, 0.000000000000000000 ) ) ;
#4620=CARTESIAN_POINT ( 'NONE',  ( 210.8300749258795577, 17.14049671552684728, -22.62267072728681683 ) ) ;
#4621=DIRECTION ( 'NONE',  ( 0.1005394128318083391, 0.05804645706261228610, -0.9932383577419438003 ) ) ;
#4624=FACE_OUTER_BOUND ( 'NONE', #6834, .T. ) ;
#4626=AXIS2_PLACEMENT_3D ( 'NONE', #17509, #2987, #3090 ) ;
#4627=DIRECTION ( 'NONE',  ( 0.8660254037844352659, 0.5000000000000056621, 0.000000000000000000 ) ) ;
#4631=FACE_OUTER_BOUND ( 'NONE', #15976, .T. ) ;
#4640=CARTESIAN_POINT ( 'NONE',  ( 192.4175317442008009, 6.510009953118869319, -14.05525385477287870 ) ) ;
#4643=EDGE_LOOP ( 'NONE', ( #16156, #155, #1489, #18989, #4013, #10388 ) ) ;
#4646=AXIS2_PLACEMENT_3D ( 'NONE', #19088, #17498, #2975 ) ;
#4654=VECTOR ( 'NONE', #11850, 999.9999999999998863 ) ;
#4657=LINE ( 'NONE', #15909, #14353 ) ;
#4659=LINE ( 'NONE', #17601, #10033 ) ;
#4667=CARTESIAN_POINT ( 'NONE',  ( 208.8577037357181894, 4.346350652224121092, -14.00000000000005507 ) ) ;
#4670=LINE ( 'NONE', #17614, #19520 ) ;
#4675=CARTESIAN_POINT ( 'NONE',  ( 195.3111273346253824, 3.525580966981323616, -11.13829696442576811 ) ) ;
#4678=EDGE_LOOP ( 'NONE', ( #3147, #20446, #18491, #5135 ) ) ;
#4682=EDGE_CURVE ( 'NONE', #4077, #16512, #18946, .T. ) ;
#4688=CARTESIAN_POINT ( 'NONE',  ( 195.3479444306255175, 4.077886589060220501, -13.97827067520021416 ) ) ;
#4696=PLANE ( 'NONE',  #16470 ) ;
#4704=DIRECTION ( 'NONE',  ( 0.5000000000000054401, -0.8660254037844354880, 0.000000000000000000 ) ) ;
#4709=ADVANCED_FACE ( 'NONE', ( #19120 ), #20699, .F. ) ;
#4712=VECTOR ( 'NONE', #8797, 1000.000000000000227 ) ;
#4716=ORIENTED_EDGE ( 'NONE', *, *, #2526, .T. ) ;
#4721=CARTESIAN_POINT ( 'NONE',  ( 209.2115421631071968, 5.174237244332543284, -26.27710986211784672 ) ) ;
#4725=CARTESIAN_POINT ( 'NONE',  ( 197.6120640069452463, 5.208066731742445832, -21.80597602412970559 ) ) ;
#4733=DIRECTION ( 'NONE',  ( -0.5000000000000053291, 0.8660254037844354880, 0.000000000000000000 ) ) ;
#4738=CARTESIAN_POINT ( 'NONE',  ( 218.0493302439821548, 9.761530332989567071, -8.625373497621339425 ) ) ;
#4744=CARTESIAN_POINT ( 'NONE',  ( 195.1526463715632076, 3.788121297904891271, -13.99656000852303173 ) ) ;
#4746=DIRECTION ( 'NONE',  ( 0.8660254037844355990, 0.5000000000000054401, 0.000000000000000000 ) ) ;
#4747=ORIENTED_EDGE ( 'NONE', *, *, #13413, .F. ) ;
#4748=AXIS2_PLACEMENT_3D ( 'NONE', #3225, #8517, #18270 ) ;
#4751=EDGE_CURVE ( 'NONE', #16239, #4535, #34, .T. ) ;
#4757=AXIS2_PLACEMENT_3D ( 'NONE', #18142, #3612, #3204 ) ;
#4767=EDGE_LOOP ( 'NONE', ( #13463, #4119, #8906, #5101 ) ) ;
#4772=FACE_OUTER_BOUND ( 'NONE', #6274, .T. ) ;
#4774=AXIS2_PLACEMENT_3D ( 'NONE', #16351, #18138, #14776 ) ;
#4775=AXIS2_PLACEMENT_3D ( 'NONE', #6849, #5349, #18199 ) ;
#4781=CARTESIAN_POINT ( 'NONE',  ( 208.8107687779841228, 4.427644383670616079, -14.00000000000005507 ) ) ;
#4785=B_SPLINE_CURVE_WITH_KNOTS ( 'NONE', 3,
 ( #15419, #2681, #9024, #10719 ),
 .UNSPECIFIED., .F., .F.,
 ( 4, 4 ),
 ( 8.431164558841520529E-05, 0.0009382973835678675096 ),
 .UNSPECIFIED. ) ;
#4786=DIRECTION ( 'NONE',  ( -0.7499999999999954481, -0.4330127018922224624, 0.5000000000000038858 ) ) ;
#4788=LINE ( 'NONE', #3400, #8571 ) ;
#4791=AXIS2_PLACEMENT_3D ( 'NONE', #3360, #8119, #17901 ) ;
#4799=ORIENTED_EDGE ( 'NONE', *, *, #9084, .T. ) ;
#4802=CARTESIAN_POINT ( 'NONE',  ( 219.6142080168453106, 10.66501293640096470, -14.00000000000005507 ) ) ;
#4803=VERTEX_POINT ( 'NONE', #6265 ) ;
#4805=ADVANCED_FACE ( 'NONE', ( #8062 ), #14570, .T. ) ;
#4807=AXIS2_PLACEMENT_3D ( 'NONE', #1223, #20397, #16070 ) ;
#4808=CARTESIAN_POINT ( 'NONE',  ( 215.5581897081276566, 15.56926723623108977, -18.15810777665862830 ) ) ;
#4809=ORIENTED_EDGE ( 'NONE', *, *, #19845, .F. ) ;
#4811=CARTESIAN_POINT ( 'NONE',  ( 214.1694065045551838, 14.94446278398596206, -7.515250618841530894 ) ) ;
#4813=EDGE_CURVE ( 'NONE', #3474, #3214, #341, .T. ) ;
#4815=ORIENTED_EDGE ( 'NONE', *, *, #4581, .T. ) ;
#4820=CIRCLE ( 'NONE', #2470, 12.47473710546057823 ) ;
#4822=ORIENTED_EDGE ( 'NONE', *, *, #12785, .T. ) ;
#4823=DIRECTION ( 'NONE',  ( 0.5000000000000054401, -0.8660254037844354880, 0.000000000000000000 ) ) ;
#4824=DIRECTION ( 'NONE',  ( -1.060575238724903217E-16, -6.123233995736827666E-17, 1.000000000000000000 ) ) ;
#4825=DIRECTION ( 'NONE',  ( 0.8660254037844355990, 0.5000000000000054401, -8.899770914925154148E-15 ) ) ;
#4827=CARTESIAN_POINT ( 'NONE',  ( 204.7255155853154918, 2.069022353175566931, -3.025685634606110952 ) ) ;
#4829=ORIENTED_EDGE ( 'NONE', *, *, #1276, .T. ) ;
#4830=CARTESIAN_POINT ( 'NONE',  ( 209.3941655698034197, 12.18747614486168906, -11.94626573465116692 ) ) ;
#4838=CARTESIAN_POINT ( 'NONE',  ( 208.2336538649943236, 4.094446933302576142, -25.81526893633797570 ) ) ;
#4843=DIRECTION ( 'NONE',  ( 0.5000000000000054401, -0.8660254037844354880, 0.000000000000000000 ) ) ;
#4845=ORIENTED_EDGE ( 'NONE', *, *, #17940, .F. ) ;
#4847=EDGE_CURVE ( 'NONE', #11315, #20129, #3485, .T. ) ;
#4848=VERTEX_POINT ( 'NONE', #451 ) ;
#4850=DIRECTION ( 'NONE',  ( 0.2961981327260292396, 0.1710100716628399076, 0.9396926207859056523 ) ) ;
#4851=CARTESIAN_POINT ( 'NONE',  ( 195.0878360447208593, 3.573686361083222796, -14.00607376310509444 ) ) ;
#4853=CONICAL_SURFACE ( 'NONE', #15035, 13.07248899748297433, 0.6693469023067423196 ) ;
#4854=ORIENTED_EDGE ( 'NONE', *, *, #15000, .T. ) ;
#4860=B_SPLINE_CURVE_WITH_KNOTS ( 'NONE', 3,
 ( #3304, #3610, #9752, #1714 ),
 .UNSPECIFIED., .F., .F.,
 ( 4, 4 ),
 ( 3.309335659841317687E-07, 0.0008543166715495293479 ),
 .UNSPECIFIED. ) ;
#4869=CARTESIAN_POINT ( 'NONE',  ( 206.3904739784022695, 10.45329399600358400, -11.31442923650852883 ) ) ;
#4874=EDGE_CURVE ( 'NONE', #4395, #6174, #14240, .T. ) ;
#4875=CARTESIAN_POINT ( 'NONE',  ( 208.0845375091750213, 4.265953788936775126, -1.899081834577966754 ) ) ;
#4887=DIRECTION ( 'NONE',  ( -0.7500000000000014433, -0.4330127018922259596, -0.4999999999999919509 ) ) ;
#4889=CARTESIAN_POINT ( 'NONE',  ( 211.2398691629905159, 12.72204434944011986, -24.79563718815145279 ) ) ;
#4891=DIRECTION ( 'NONE',  ( 0.3886714912512188591, 0.2243995901002276971, -0.8936326403234180482 ) ) ;
#4895=EDGE_LOOP ( 'NONE', ( #4845, #3011, #15915, #15122 ) ) ;
#4905=ORIENTED_EDGE ( 'NONE', *, *, #20501, .F. ) ;
#4909=LINE ( 'NONE', #3220, #12949 ) ;
#4915=ORIENTED_EDGE ( 'NONE', *, *, #10307, .T. ) ;
#4916=CARTESIAN_POINT ( 'NONE',  ( 207.8564944041415288, 11.29970128344166369, -11.99421842325719467 ) ) ;
#4917=VERTEX_POINT ( 'NONE', #8382 ) ;
#4920=CARTESIAN_POINT ( 'NONE',  ( 209.3577037357181894, 3.480325248439694263, -14.00000000000005507 ) ) ;
#4921=AXIS2_PLACEMENT_3D ( 'NONE', #16438, #11993, #440 ) ;
#4923=CARTESIAN_POINT ( 'NONE',  ( 209.1177676012032407, 5.377710327540435209, -26.45271578590685380 ) ) ;
#4932=CONICAL_SURFACE ( 'NONE', #12730, 13.07248899748297433, 0.6693469023067423196 ) ;
#4937=DIRECTION ( 'NONE',  ( 0.5000000000000049960, -0.8660254037844357100, 0.000000000000000000 ) ) ;
#4941=VERTEX_POINT ( 'NONE', #654 ) ;
#4945=ORIENTED_EDGE ( 'NONE', *, *, #5947, .T. ) ;
#4950=AXIS2_PLACEMENT_3D ( 'NONE', #18786, #5719, #4039 ) ;
#4959=CARTESIAN_POINT ( 'NONE',  ( 216.6640881527418401, 8.961760438719156951, -23.53124788243930610 ) ) ;
#4961=LINE ( 'NONE', #108, #10236 ) ;
#4965=VERTEX_POINT ( 'NONE', #8914 ) ;
#4970=DIRECTION ( 'NONE',  ( 0.5566703992264088185, 0.3213938048432679051, -0.7660444431189864511 ) ) ;
#4975=EDGE_CURVE ( 'NONE', #8807, #20547, #11855, .T. ) ;
#4978=ADVANCED_FACE ( 'NONE', ( #15514 ), #7417, .F. ) ;
#4982=ADVANCED_FACE ( 'NONE', ( #13906 ), #12101, .T. ) ;
#4985=LINE ( 'NONE', #12966, #15714 ) ;
#4987=VERTEX_POINT ( 'NONE', #13597 ) ;
#4989=ADVANCED_FACE ( 'NONE', ( #20052 ), #10146, .T. ) ;
#4994=VECTOR ( 'NONE', #4343, 1000.000000000000227 ) ;
#4998=EDGE_CURVE ( 'NONE', #18930, #12331, #15610, .T. ) ;
#5000=EDGE_LOOP ( 'NONE', ( #2473, #17932, #3278, #19368, #13783, #6281 ) ) ;
#5005=VECTOR ( 'NONE', #14351, 1000.000000000000114 ) ;
#5007=CARTESIAN_POINT ( 'NONE',  ( 195.2378745322255611, 8.138335620992030783, -7.515250618841283092 ) ) ;
#5009=EDGE_CURVE ( 'NONE', #340, #791, #18570, .T. ) ;
#5010=CARTESIAN_POINT ( 'NONE',  ( 213.5545353545354601, 14.58946676000514486, -21.69368824361360382 ) ) ;
#5015=DIRECTION ( 'NONE',  ( -0.5000000000000054401, 0.8660254037844354880, -0.000000000000000000 ) ) ;
#5019=VECTOR ( 'NONE', #6472, 1000.000000000000000 ) ;
#5020=DIRECTION ( 'NONE',  ( -0.7235536692358585098, -0.4177439057064706307, 0.5495089780708131144 ) ) ;
#5024=PRODUCT_DEFINITION_FORMATION_WITH_SPECIFIED_SOURCE ( 'ANY', '', #12121, .NOT_KNOWN. ) ;
#5027=DIRECTION ( 'NONE',  ( -0.8660254037844355990, -0.5000000000000054401, 0.000000000000000000 ) ) ;
#5032=VERTEX_POINT ( 'NONE', #16980 ) ;
#5035=DIRECTION ( 'NONE',  ( -0.5000000000000054401, 0.8660254037844354880, -0.000000000000000000 ) ) ;
#5039=ORIENTED_EDGE ( 'NONE', *, *, #16901, .F. ) ;
#5040=ORIENTED_EDGE ( 'NONE', *, *, #19252, .T. ) ;
#5042=CARTESIAN_POINT ( 'NONE',  ( 201.4983898220421850, 0.4634396488479761711, -22.82042918318446212 ) ) ;
#5044=VERTEX_POINT ( 'NONE', #17189 ) ;
#5045=EDGE_LOOP ( 'NONE', ( #20045, #3314, #3913 ) ) ;
#5049=CARTESIAN_POINT ( 'NONE',  ( 201.9167561165444056, 0.4473843177916839164, -14.00000000000005507 ) ) ;
#5050=ORIENTED_EDGE ( 'NONE', *, *, #2121, .T. ) ;
#5051=AXIS2_PLACEMENT_3D ( 'NONE', #18943, #12696, #2839 ) ;
#5052=ORIENTED_EDGE ( 'NONE', *, *, #8061, .T. ) ;
#5060=CARTESIAN_POINT ( 'NONE',  ( 208.0983737146324870, 5.661548828456886895, -14.00000000000005507 ) ) ;
#5061=ORIENTED_EDGE ( 'NONE', *, *, #7329, .F. ) ;
#5063=VECTOR ( 'NONE', #8503, 1000.000000000000000 ) ;
#5069=AXIS2_PLACEMENT_3D ( 'NONE', #8542, #6940, #700 ) ;
#5072=DIRECTION ( 'NONE',  ( -0.5000000000000049960, 0.8660254037844358210, -0.000000000000000000 ) ) ;
#5080=DIRECTION ( 'NONE',  ( 0.8660254037844355990, 0.5000000000000054401, 0.000000000000000000 ) ) ;
#5089=DIRECTION ( 'NONE',  ( 0.7739085681710395903, 0.4468163201617135760, 0.4487991802004505648 ) ) ;
#5091=ORIENTED_EDGE ( 'NONE', *, *, #6283, .T. ) ;
#5092=CARTESIAN_POINT ( 'NONE',  ( 200.4364383576235866, 6.484680665789935183, -3.188775577416750995 ) ) ;
#5094=AXIS2_PLACEMENT_3D ( 'NONE', #14839, #11525, #17584 ) ;
#5097=ORIENTED_EDGE ( 'NONE', *, *, #3830, .T. ) ;
#5098=ORIENTED_EDGE ( 'NONE', *, *, #15669, .F. ) ;
#5101=ORIENTED_EDGE ( 'NONE', *, *, #6789, .T. ) ;
#5102=ORIENTED_EDGE ( 'NONE', *, *, #3972, .T. ) ;
#5107=DIRECTION ( 'NONE',  ( -0.5000000000000049960, 0.8660254037844358210, -0.000000000000000000 ) ) ;
#5108=EDGE_CURVE ( 'NONE', #16512, #255, #5449, .T. ) ;
#5109=VECTOR ( 'NONE', #5124, 1000.000000000000000 ) ;
#5110=CARTESIAN_POINT ( 'NONE',  ( 209.4254563108873413, 4.782534396259779719, -2.187257959407755248 ) ) ;
#5115=CARTESIAN_POINT ( 'NONE',  ( 188.6991442264338446, 14.97787164915609104, -11.13829696442576811 ) ) ;
#5117=LINE ( 'NONE', #6815, #7779 ) ;
#5120=ADVANCED_FACE ( 'NONE', ( #10041 ), #11200, .T. ) ;
#5121=EDGE_LOOP ( 'NONE', ( #18026, #14518, #5347 ) ) ;
#5122=EDGE_CURVE ( 'NONE', #18502, #8117, #19612, .T. ) ;
#5124=DIRECTION ( 'NONE',  ( 0.8426815769442658199, 0.4865224352899167326, -0.2306158707424411092 ) ) ;
#5125=CARTESIAN_POINT ( 'NONE',  ( 219.1667714839435632, 10.92189157256192900, -15.42246552719623587 ) ) ;
#5126=CONICAL_SURFACE ( 'NONE', #16995, 10.85470691220533190, 0.8171114040043576665 ) ;
#5127=AXIS2_PLACEMENT_3D ( 'NONE', #4348, #17493, #10800 ) ;
#5130=DIRECTION ( 'NONE',  ( 0.9885408208161367005, 0.000000000000000000, -0.1509537862398905028 ) ) ;
#5131=EDGE_CURVE ( 'NONE', #4941, #4987, #8360, .T. ) ;
#5135=ORIENTED_EDGE ( 'NONE', *, *, #13192, .T. ) ;
#5136=PLANE ( 'NONE',  #20393 ) ;
#5139=EDGE_CURVE ( 'NONE', #17374, #20019, #2707, .T. ) ;
#5142=DIRECTION ( 'NONE',  ( -0.6518835024542816159, 0.000000000000000000, 0.7583191275630192241 ) ) ;
#5143=CIRCLE ( 'NONE', #2460, 1.003313105759049417 ) ;
#5145=ORIENTED_EDGE ( 'NONE', *, *, #15109, .T. ) ;
#5148=CARTESIAN_POINT ( 'NONE',  ( 215.9755601355957424, 15.98724606906508683, -13.98704593443257771 ) ) ;
#5149=CARTESIAN_POINT ( 'NONE',  ( 200.3972727712213668, 6.993117665730062882, -3.627429155984474907 ) ) ;
#5150=VERTEX_POINT ( 'NONE', #16533 ) ;
#5158=CARTESIAN_POINT ( 'NONE',  ( 208.4761278624580711, 5.007259451653140125, -14.00000000000005507 ) ) ;
#5164=EDGE_LOOP ( 'NONE', ( #19040, #1390, #998, #1524 ) ) ;
#5165=CARTESIAN_POINT ( 'NONE',  ( 210.6089461623840009, 5.465822580604545955, -25.65046807331635748 ) ) ;
#5172=VERTEX_POINT ( 'NONE', #9835 ) ;
#5175=ORIENTED_EDGE ( 'NONE', *, *, #13805, .F. ) ;
#5176=LINE ( 'NONE', #6656, #9693 ) ;
#5178=CARTESIAN_POINT ( 'NONE',  ( 218.1033169702945997, 10.30790582283579759, -19.52417598135495425 ) ) ;
#5186=PLANE ( 'NONE',  #3478 ) ;
#5188=DIRECTION ( 'NONE',  ( -0.8137976813493728034, -0.4698463103929603757, -0.3420201433256622736 ) ) ;
#5190=CARTESIAN_POINT ( 'NONE',  ( 198.5343390728978932, -1.505455072869313238, -12.62839849932143643 ) ) ;
#5192=CARTESIAN_POINT ( 'NONE',  ( 215.9194406937061217, 8.531838027793467560, -5.321846656828220112 ) ) ;
#5202=FACE_OUTER_BOUND ( 'NONE', #14623, .T. ) ;
#5203=ORIENTED_EDGE ( 'NONE', *, *, #1995, .T. ) ;
#5210=VECTOR ( 'NONE', #5107, 1000.000000000000227 ) ;
#5216=DIRECTION ( 'NONE',  ( -0.9987303135603810000, 0.000000000000000000, -0.05037619254750287656 ) ) ;
#5224=ADVANCED_FACE ( 'NONE', ( #5276 ), #18225, .F. ) ;
#5226=VECTOR ( 'NONE', #2617, 1000.000000000000000 ) ;
#5232=EDGE_CURVE ( 'NONE', #18162, #11248, #16853, .T. ) ;
#5238=AXIS2_PLACEMENT_3D ( 'NONE', #9173, #10875, #10989 ) ;
#5239=CARTESIAN_POINT ( 'NONE',  ( 208.3092871949524749, 11.56112132310348528, -12.02050488595160438 ) ) ;
#5243=ORIENTED_EDGE ( 'NONE', *, *, #2865, .T. ) ;
#5244=ORIENTED_EDGE ( 'NONE', *, *, #13250, .F. ) ;
#5245=ORIENTED_EDGE ( 'NONE', *, *, #13128, .F. ) ;
#5246=CARTESIAN_POINT ( 'NONE',  ( 201.0525450381139194, 0.7212519096665224172, -23.06309126349794525 ) ) ;
#5255=CARTESIAN_POINT ( 'NONE',  ( 212.5077365114557040, 18.10909508356834863, -22.49869731917979365 ) ) ;
#5260=AXIS2_PLACEMENT_3D ( 'NONE', #13352, #18430, #15067 ) ;
#5261=CARTESIAN_POINT ( 'NONE',  ( 215.9066831210195687, 15.94747990615854505, -12.62152863576173090 ) ) ;
#5262=EDGE_CURVE ( 'NONE', #12427, #11581, #14847, .T. ) ;
#5263=CARTESIAN_POINT ( 'NONE',  ( 209.8762589913677061, 12.46581291157636429, -13.00118852497347355 ) ) ;
#5267=ADVANCED_FACE ( 'NONE', ( #19912 ), #5692, .T. ) ;
#5274=ORIENTED_EDGE ( 'NONE', *, *, #1350, .T. ) ;
#5276=FACE_OUTER_BOUND ( 'NONE', #10013, .T. ) ;
#5278=CARTESIAN_POINT ( 'NONE',  ( 212.9548847052525957, 4.941433797637768244, -14.00000000000005507 ) ) ;
#5281=CARTESIAN_POINT ( 'NONE',  ( 213.5545353545354601, 14.58946676000514486, -21.69368824361360382 ) ) ;
#5283=CARTESIAN_POINT ( 'NONE',  ( 191.8105349496822782, 16.77423392077770004, -4.915515517929134326 ) ) ;
#5288=ORIENTED_EDGE ( 'NONE', *, *, #20924, .T. ) ;
#5290=DIRECTION ( 'NONE',  ( -0.9367698044638387289, 0.000000000000000000, 0.3499461864984122483 ) ) ;
#5291=FACE_OUTER_BOUND ( 'NONE', #12189, .T. ) ;
#5298=VERTEX_POINT ( 'NONE', #5378 ) ;
#5299=ORIENTED_EDGE ( 'NONE', *, *, #13692, .F. ) ;
#5304=EDGE_LOOP ( 'NONE', ( #18606, #16668, #901, #18200 ) ) ;
#5306=CARTESIAN_POINT ( 'NONE',  ( 198.4658173668363190, 5.877991368080599521, -5.291540431471293715 ) ) ;
#5307=CARTESIAN_POINT ( 'NONE',  ( 218.0493302439821548, 9.761530332989567071, -8.625373497621339425 ) ) ;
#5312=AXIS2_PLACEMENT_3D ( 'NONE', #10766, #9174, #19254 ) ;
#5326=CARTESIAN_POINT ( 'NONE',  ( 206.4681030732283205, 9.967063913005945963, -26.45271578590685380 ) ) ;
#5331=AXIS2_PLACEMENT_3D ( 'NONE', #6055, #20693, #15738 ) ;
#5338=CARTESIAN_POINT ( 'NONE',  ( 212.9202825050182923, 6.800273240212296955, -24.96223045542567931 ) ) ;
#5339=CARTESIAN_POINT ( 'NONE',  ( 195.8472345282168874, 4.366151861308305016, -18.11117897393217646 ) ) ;
#5340=ADVANCED_FACE ( 'NONE', ( #13881 ), #5805, .F. ) ;
#5342=CARTESIAN_POINT ( 'NONE',  ( 208.1005406747554787, 4.017593997085510793, -27.13030671846408737 ) ) ;
#5347=ORIENTED_EDGE ( 'NONE', *, *, #16416, .T. ) ;
#5349=DIRECTION ( 'NONE',  ( -0.5000000000000054401, 0.8660254037844354880, -0.000000000000000000 ) ) ;
#5351=ORIENTED_EDGE ( 'NONE', *, *, #2161, .T. ) ;
#5352=ORIENTED_EDGE ( 'NONE', *, *, #12394, .T. ) ;
#5359=CARTESIAN_POINT ( 'NONE',  ( 199.3787015603994917, 6.051018721616807206, -4.128377653168135986 ) ) ;
#5360=EDGE_LOOP ( 'NONE', ( #10412, #4540, #5677, #18072 ) ) ;
#5362=DIRECTION ( 'NONE',  ( -0.5000000000000049960, 0.8660254037844357100, -0.000000000000000000 ) ) ;
#5364=CARTESIAN_POINT ( 'NONE',  ( 195.2174643819972744, 4.002553897860817500, -13.98704593443225797 ) ) ;
#5368=VERTEX_POINT ( 'NONE', #13570 ) ;
#5369=ADVANCED_FACE ( 'NONE', ( #16638 ), #15390, .T. ) ;
#5372=VERTEX_POINT ( 'NONE', #13781 ) ;
#5373=ORIENTED_EDGE ( 'NONE', *, *, #19650, .T. ) ;
#5378=CARTESIAN_POINT ( 'NONE',  ( 199.0852767235472527, -1.187371071960172664, -9.928836400542227381 ) ) ;
#5380=EDGE_CURVE ( 'NONE', #2174, #2247, #14597, .T. ) ;
#5382=VERTEX_POINT ( 'NONE', #18862 ) ;
#5383=CARTESIAN_POINT ( 'NONE',  ( 205.6089461623839441, 14.12607661844890039, -25.65046807331635748 ) ) ;
#5385=CARTESIAN_POINT ( 'NONE',  ( 208.8107687779841228, 4.427644383670616079, -14.00000000000005507 ) ) ;
#5392=FACE_OUTER_BOUND ( 'NONE', #20518, .T. ) ;
#5396=CARTESIAN_POINT ( 'NONE',  ( 199.2144802262915846, 21.04890371929339921, -14.00000000000005507 ) ) ;
#5397=LINE ( 'NONE', #13483, #10884 ) ;
#5399=EDGE_CURVE ( 'NONE', #5150, #835, #7504, .T. ) ;
#5401=DIRECTION ( 'NONE',  ( 0.8660254037844355990, 0.5000000000000054401, 0.000000000000000000 ) ) ;
#5414=CARTESIAN_POINT ( 'NONE',  ( 196.1661066256804986, 4.019203490823548997, -8.415281845791808379 ) ) ;
#5415=VECTOR ( 'NONE', #4335, 1000.000000000000227 ) ;
#5418=DIRECTION ( 'NONE',  ( 0.8426815769442655979, 0.4865224352899170102, -0.2306158707424410814 ) ) ;
#5419=CARTESIAN_POINT ( 'NONE',  ( 199.3161926515599589, -0.7964524749548287375, -19.43577154980779298 ) ) ;
#5420=ORIENTED_EDGE ( 'NONE', *, *, #14113, .T. ) ;
#5422=CARTESIAN_POINT ( 'NONE',  ( 197.6529114527598381, 5.408659919762685675, -6.286464976498783663 ) ) ;
#5423=CARTESIAN_POINT ( 'NONE',  ( 196.3164214246273218, 4.637037042251114904, -19.36714384557513924 ) ) ;
#5436=CONICAL_SURFACE ( 'NONE', #11902, 10.85470691220533190, 0.8171114040043576665 ) ;
#5437=EDGE_CURVE ( 'NONE', #6217, #5656, #20752, .T. ) ;
#5444=CARTESIAN_POINT ( 'NONE',  ( 205.0662616026534693, 10.91332106064940888, -14.00000000000005507 ) ) ;
#5448=ORIENTED_EDGE ( 'NONE', *, *, #18902, .T. ) ;
#5449=B_SPLINE_CURVE_WITH_KNOTS ( 'NONE', 3,
 ( #8037, #11549, #3592, #18122 ),
 .UNSPECIFIED., .F., .F.,
 ( 4, 4 ),
 ( 0.0001020613991901207350, 0.0009560471371670607125 ),
 .UNSPECIFIED. ) ;
#5450=ORIENTED_EDGE ( 'NONE', *, *, #4034, .T. ) ;
#5451=ORIENTED_EDGE ( 'NONE', *, *, #2952, .T. ) ;
#5455=ADVANCED_FACE ( 'NONE', ( #15588 ), #15286, .T. ) ;
#5464=CARTESIAN_POINT ( 'NONE',  ( 209.0038672028605049, 11.96213727764292756, -16.47016555539322269 ) ) ;
#5466=ORIENTED_EDGE ( 'NONE', *, *, #13945, .T. ) ;
#5471=AXIS2_PLACEMENT_3D ( 'NONE', #6807, #14899, #567 ) ;
#5472=AXIS2_PLACEMENT_3D ( 'NONE', #14302, #12697, #19155 ) ;
#5475=CARTESIAN_POINT ( 'NONE',  ( 207.0496559082687043, 3.410865394267065032, -2.341985411376944271 ) ) ;
#5476=ORIENTED_EDGE ( 'NONE', *, *, #19219, .T. ) ;
#5478=LINE ( 'NONE', #14957, #17133 ) ;
#5479=ADVANCED_FACE ( 'NONE', ( #17480 ), #12404, .F. ) ;
#5483=ORIENTED_EDGE ( 'NONE', *, *, #19229, .T. ) ;
#5488=CIRCLE ( 'NONE', #10218, 4.389613146203297234 ) ;
#5489=EDGE_CURVE ( 'NONE', #772, #18586, #1164, .T. ) ;
#5495=CARTESIAN_POINT ( 'NONE',  ( 205.8264633344831225, 9.596613037118636669, -14.00000000000005507 ) ) ;
#5501=CARTESIAN_POINT ( 'NONE',  ( 205.0662616026534693, 10.91332106064940888, -14.00000000000005507 ) ) ;
#5502=AXIS2_PLACEMENT_3D ( 'NONE', #5060, #8348, #13559 ) ;
#5506=DIRECTION ( 'NONE',  ( -0.5000000000000054401, 0.8660254037844354880, -0.000000000000000000 ) ) ;
#5507=CARTESIAN_POINT ( 'NONE',  ( 215.9066831210195687, 15.94747990615854505, -12.62152863576173090 ) ) ;
#5511=ORIENTED_EDGE ( 'NONE', *, *, #6157, .T. ) ;
#5513=DIRECTION ( 'NONE',  ( 0.8660254037844352659, 0.5000000000000056621, 0.000000000000000000 ) ) ;
#5519=CIRCLE ( 'NONE', #14698, 4.389613146203297234 ) ;
#5521=VERTEX_POINT ( 'NONE', #3054 ) ;
#5523=EDGE_CURVE ( 'NONE', #10176, #9778, #4318, .T. ) ;
#5525=CARTESIAN_POINT ( 'NONE',  ( 211.7650478275019168, 6.133298188171013798, -25.44774858730800560 ) ) ;
#5526=CARTESIAN_POINT ( 'NONE',  ( 219.1556129512320013, 10.40024295182009517, -13.98474561060134747 ) ) ;
#5530=DIRECTION ( 'NONE',  ( -0.5000000000000054401, 0.8660254037844354880, -0.000000000000000000 ) ) ;
#5531=DIRECTION ( 'NONE',  ( -0.5000000000000049960, 0.8660254037844357100, -0.000000000000000000 ) ) ;
#5532=ORIENTED_EDGE ( 'NONE', *, *, #11081, .F. ) ;
#5533=VECTOR ( 'NONE', #8257, 1000.000000000000227 ) ;
#5534=VECTOR ( 'NONE', #9628, 1000.000000000000114 ) ;
#5540=ORIENTED_EDGE ( 'NONE', *, *, #10434, .F. ) ;
#5541=ORIENTED_EDGE ( 'NONE', *, *, #5679, .F. ) ;
#5548=ORIENTED_EDGE ( 'NONE', *, *, #7269, .F. ) ;
#5561=CARTESIAN_POINT ( 'NONE',  ( 202.6438527999323185, 0.8671737836725290638, -4.409371045252821197 ) ) ;
#5567=DIRECTION ( 'NONE',  ( 0.5000000000000054401, -0.8660254037844354880, 0.000000000000000000 ) ) ;
#5568=ORIENTED_EDGE ( 'NONE', *, *, #8290, .F. ) ;
#5571=ORIENTED_EDGE ( 'NONE', *, *, #19483, .T. ) ;
#5574=EDGE_CURVE ( 'NONE', #1000, #13448, #11524, .T. ) ;
#5575=VECTOR ( 'NONE', #12538, 1000.000000000000227 ) ;
#5578=CARTESIAN_POINT ( 'NONE',  ( 209.4254563108873413, 4.782534396259798370, -2.075899210536075401 ) ) ;
#5582=ORIENTED_EDGE ( 'NONE', *, *, #20624, .T. ) ;
#5590=VERTEX_POINT ( 'NONE', #19678 ) ;
#5591=VECTOR ( 'NONE', #10582, 999.9999999999998863 ) ;
#5592=ORIENTED_EDGE ( 'NONE', *, *, #15285, .T. ) ;
#5594=AXIS2_PLACEMENT_3D ( 'NONE', #1816, #7858, #11458 ) ;
#5601=CARTESIAN_POINT ( 'NONE',  ( 211.7650478275019168, 6.133298188171013798, -25.44774858730800560 ) ) ;
#5602=DIRECTION ( 'NONE',  ( -0.5000000000000054401, 0.8660254037844354880, -0.000000000000000000 ) ) ;
#5607=DIRECTION ( 'NONE',  ( -0.8660254037844354880, -0.5000000000000055511, 0.000000000000000000 ) ) ;
#5609=CIRCLE ( 'NONE', #16129, 7.960520131757807150 ) ;
#5618=AXIS2_PLACEMENT_3D ( 'NONE', #10529, #17115, #17014 ) ;
#5628=FACE_BOUND ( 'NONE', #16060, .T. ) ;
#5630=FACE_OUTER_BOUND ( 'NONE', #17961, .T. ) ;
#5631=DIRECTION ( 'NONE',  ( -0.8660254037844357100, -0.5000000000000051070, 0.000000000000000000 ) ) ;
#5632=EDGE_LOOP ( 'NONE', ( #1624, #11668, #192, #1021, #8427, #13723 ) ) ;
#5636=DIRECTION ( 'NONE',  ( -1.000000000000000000, 0.000000000000000000, 0.000000000000000000 ) ) ;
#5637=EDGE_CURVE ( 'NONE', #1337, #8365, #7087, .T. ) ;
#5643=CARTESIAN_POINT ( 'NONE',  ( 209.3577037357181894, 3.480325248439696040, -14.00000000000005507 ) ) ;
#5646=CARTESIAN_POINT ( 'NONE',  ( 208.8577037357181894, 4.346350652224124644, -14.00000000000005507 ) ) ;
#5649=CARTESIAN_POINT ( 'NONE',  ( 219.5332756341046547, 10.61828660343948272, -18.44761907388206623 ) ) ;
#5650=ORIENTED_EDGE ( 'NONE', *, *, #9084, .F. ) ;
#5651=AXIS2_PLACEMENT_3D ( 'NONE', #7372, #925, #6958 ) ;
#5654=EDGE_CURVE ( 'NONE', #18696, #20283, #11220, .T. ) ;
#5656=VERTEX_POINT ( 'NONE', #9915 ) ;
#5658=LINE ( 'NONE', #13739, #18544 ) ;
#5663=VERTEX_POINT ( 'NONE', #11323 ) ;
#5674=DIRECTION ( 'NONE',  ( 0.7739085681710340392, 0.4468163201617105229, -0.4487991802004632214 ) ) ;
#5677=ORIENTED_EDGE ( 'NONE', *, *, #19471, .T. ) ;
#5679=EDGE_CURVE ( 'NONE', #19959, #20444, #19276, .T. ) ;
#5682=PLANE ( 'NONE',  #2487 ) ;
#5684=CARTESIAN_POINT ( 'NONE',  ( 199.2655634166889911, -1.083282501143478793, -21.18305361806749332 ) ) ;
#5686=ORIENTED_EDGE ( 'NONE', *, *, #478, .T. ) ;
#5687=DIRECTION ( 'NONE',  ( -0.5000000000000049960, 0.8660254037844357100, -0.000000000000000000 ) ) ;
#5690=VERTEX_POINT ( 'NONE', #15968 ) ;
#5691=ORIENTED_EDGE ( 'NONE', *, *, #2704, .T. ) ;
#5692=CYLINDRICAL_SURFACE ( 'NONE', #10502, 4.999999999999973355 ) ;
#5696=VERTEX_POINT ( 'NONE', #10857 ) ;
#5697=EDGE_CURVE ( 'NONE', #15357, #2200, #16289, .T. ) ;
#5705=DIRECTION ( 'NONE',  ( 0.8944271909999147452, 0.000000000000000000, -0.4472135954999602592 ) ) ;
#5706=CARTESIAN_POINT ( 'NONE',  ( 199.1738290307970374, -1.136245373532171588, -9.972943347741736630 ) ) ;
#5707=ORIENTED_EDGE ( 'NONE', *, *, #7586, .F. ) ;
#5709=DIRECTION ( 'NONE',  ( -1.000000000000000000, 0.000000000000000000, 0.000000000000000000 ) ) ;
#5710=CARTESIAN_POINT ( 'NONE',  ( 208.0983737146324870, 5.661548828456886895, -14.00000000000005507 ) ) ;
#5714=ORIENTED_EDGE ( 'NONE', *, *, #12001, .F. ) ;
#5716=LINE ( 'NONE', #8703, #864 ) ;
#5719=DIRECTION ( 'NONE',  ( -0.1503837331804321054, -0.08682408883346430517, 0.9848077530122086864 ) ) ;
#5720=AXIS2_PLACEMENT_3D ( 'NONE', #1658, #9695, #17360 ) ;
#5722=CARTESIAN_POINT ( 'NONE',  ( 202.6226596002730389, 0.8549378841442712984, -23.57241037536569195 ) ) ;
#5724=CARTESIAN_POINT ( 'NONE',  ( 205.5965122587965084, 9.994899983462953941, -14.00000000000005507 ) ) ;
#5726=DIRECTION ( 'NONE',  ( -0.8296432542242783148, -0.4789947561577510560, -0.2868032327110804358 ) ) ;
#5727=EDGE_CURVE ( 'NONE', #11917, #10920, #6327, .T. ) ;
#5731=AXIS2_PLACEMENT_3D ( 'NONE', #6170, #4593, #12551 ) ;
#5733=DIRECTION ( 'NONE',  ( -0.8645602258681710506, -0.4991540791356393614, 0.05814482891047953461 ) ) ;
#5740=EDGE_LOOP ( 'NONE', ( #5175, #18566, #14082, #13221, #3538, #20278 ) ) ;
#5742=VECTOR ( 'NONE', #5978, 1000.000000000000114 ) ;
#5748=EDGE_CURVE ( 'NONE', #7006, #10440, #11546, .T. ) ;
#5751=DIRECTION ( 'NONE',  ( -0.8660254037844355990, -0.5000000000000054401, 4.435979565408006148E-14 ) ) ;
#5755=CARTESIAN_POINT ( 'NONE',  ( 198.3351478706185276, -1.493051479916005730, -13.98983052576385866 ) ) ;
#5756=AXIS2_PLACEMENT_3D ( 'NONE', #12400, #9083, #940 ) ;
#5757=DIRECTION ( 'NONE',  ( -0.5000000000000054401, 0.8660254037844354880, -0.000000000000000000 ) ) ;
#5759=EDGE_LOOP ( 'NONE', ( #13009, #18702, #13212, #8419 ) ) ;
#5762=ADVANCED_FACE ( 'NONE', ( #4607 ), #17440, .F. ) ;
#5768=EDGE_CURVE ( 'NONE', #20411, #8176, #43, .T. ) ;
#5769=ORIENTED_EDGE ( 'NONE', *, *, #10182, .T. ) ;
#5773=AXIS2_PLACEMENT_3D ( 'NONE', #16712, #17603, #2190 ) ;
#5777=DIRECTION ( 'NONE',  ( 0.8660254037844355990, 0.5000000000000054401, 1.074925455818303755E-13 ) ) ;
#5783=AXIS2_PLACEMENT_3D ( 'NONE', #574, #20173, #5636 ) ;
#5784=CARTESIAN_POINT ( 'NONE',  ( 210.1178786253386193, 12.07426281049857408, -2.551678190571530891 ) ) ;
#5792=CARTESIAN_POINT ( 'NONE',  ( 201.1037701599415755, 22.13968577106347269, -1.717498466822861225 ) ) ;
#5805=PLANE ( 'NONE',  #1036 ) ;
#5820=LINE ( 'NONE', #2662, #12052 ) ;
#5822=LINE ( 'NONE', #10598, #19548 ) ;
#5825=ORIENTED_EDGE ( 'NONE', *, *, #3981, .T. ) ;
#5830=VERTEX_POINT ( 'NONE', #4398 ) ;
#5831=ORIENTED_EDGE ( 'NONE', *, *, #20924, .F. ) ;
#5836=DIRECTION ( 'NONE',  ( -0.2483788854152946257, -0.1434016163555414947, 0.9579895123154918979 ) ) ;
#5841=CARTESIAN_POINT ( 'NONE',  ( 208.0983737146324870, 5.661548828456886895, -14.00000000000005507 ) ) ;
#5844=DIRECTION ( 'NONE',  ( -0.5000000000000055511, 0.8660254037844354880, 0.000000000000000000 ) ) ;
#5845=CARTESIAN_POINT ( 'NONE',  ( 205.5965122587965084, 9.994899983462952164, -14.00000000000005507 ) ) ;
#5846=CARTESIAN_POINT ( 'NONE',  ( 205.3906008270068071, 3.225829587143459243, -2.044871543906942701 ) ) ;
#5852=VECTOR ( 'NONE', #6163, 1000.000000000000114 ) ;
#5856=ADVANCED_FACE ( 'NONE', ( #6811 ), #6473, .T. ) ;
#5859=VERTEX_POINT ( 'NONE', #5010 ) ;
#5867=AXIS2_PLACEMENT_3D ( 'NONE', #3509, #6777, #5290 ) ;
#5884=CIRCLE ( 'NONE', #17754, 11.98469917212512215 ) ;
#5887=ORIENTED_EDGE ( 'NONE', *, *, #16146, .F. ) ;
#5888=EDGE_CURVE ( 'NONE', #16315, #7807, #8824, .T. ) ;
#5889=FACE_OUTER_BOUND ( 'NONE', #1534, .T. ) ;
#5894=ADVANCED_FACE ( 'NONE', ( #5630 ), #13614, .T. ) ;
#5895=CARTESIAN_POINT ( 'NONE',  ( 196.8823445864675534, 4.963772932080226852, -7.502777792348571673 ) ) ;
#5899=CARTESIAN_POINT ( 'NONE',  ( 218.9852377222535154, 11.07469685814948157, -16.89203719259520753 ) ) ;
#5903=CARTESIAN_POINT ( 'NONE',  ( 205.0662616026534693, 10.91332106064940888, -14.00000000000005507 ) ) ;
#5904=CARTESIAN_POINT ( 'NONE',  ( 200.8894739819445192, 11.40128808463920329, -25.34310559273323804 ) ) ;
#5908=ORIENTED_EDGE ( 'NONE', *, *, #1252, .F. ) ;
#5915=AXIS2_PLACEMENT_3D ( 'NONE', #392, #14826, #16297 ) ;
#5917=ADVANCED_FACE ( 'NONE', ( #12227 ), #18708, .T. ) ;
#5919=DIRECTION ( 'NONE',  ( 0.5000000000000049960, -0.8660254037844358210, 0.000000000000000000 ) ) ;
#5926=ORIENTED_EDGE ( 'NONE', *, *, #14356, .T. ) ;
#5929=ORIENTED_EDGE ( 'NONE', *, *, #11454, .F. ) ;
#5931=ORIENTED_EDGE ( 'NONE', *, *, #3923, .T. ) ;
#5936=LINE ( 'NONE', #12436, #11988 ) ;
#5940=CARTESIAN_POINT ( 'NONE',  ( 205.0662616026534693, 10.91332106064940888, -14.00000000000005507 ) ) ;
#5942=ORIENTED_EDGE ( 'NONE', *, *, #19125, .F. ) ;
#5945=DIRECTION ( 'NONE',  ( 0.5000000000000051070, -0.8660254037844359321, 0.000000000000000000 ) ) ;
#5946=PLANE ( 'NONE',  #19654 ) ;
#5947=EDGE_CURVE ( 'NONE', #19425, #3223, #20268, .T. ) ;
#5948=DIRECTION ( 'NONE',  ( 0.2961981327260175823, 0.1710100716628329964, -0.9396926207859105373 ) ) ;
#5949=ORIENTED_EDGE ( 'NONE', *, *, #2123, .T. ) ;
#5950=DIRECTION ( 'NONE',  ( -0.7951984747223580507, -0.4591080534401394408, 0.3960797660391671138 ) ) ;
#5951=DIRECTION ( 'NONE',  ( -0.8660254037844355990, -0.5000000000000054401, 0.000000000000000000 ) ) ;
#5952=AXIS2_PLACEMENT_3D ( 'NONE', #18367, #244, #6685 ) ;
#5956=VERTEX_POINT ( 'NONE', #10399 ) ;
#5958=DIRECTION ( 'NONE',  ( 0.5000000000000054401, -0.8660254037844354880, 0.000000000000000000 ) ) ;
#5963=ADVANCED_FACE ( 'NONE', ( #568 ), #18694, .F. ) ;
#5967=CARTESIAN_POINT ( 'NONE',  ( 201.4752803508637271, 7.615505632025055149, -24.99940654434229970 ) ) ;
#5968=ORIENTED_EDGE ( 'NONE', *, *, #9109, .F. ) ;
#5969=DIRECTION ( 'NONE',  ( -0.7951984747223626027, -0.4591080534401424385, -0.3960797660391544017 ) ) ;
#5971=VERTEX_POINT ( 'NONE', #17101 ) ;
#5975=DIRECTION ( 'NONE',  ( 0.5943026915289566503, 0.3431208189343674109, -0.7273736415730548410 ) ) ;
#5978=DIRECTION ( 'NONE',  ( 0.5566703992264184775, 0.3213938048432737893, 0.7660444431189769032 ) ) ;
#5982=ORIENTED_EDGE ( 'NONE', *, *, #977, .T. ) ;
#5985=DIRECTION ( 'NONE',  ( -0.7739085681710340392, -0.4468163201617105229, 0.4487991802004632214 ) ) ;
#5986=DIRECTION ( 'NONE',  ( 0.8660254037844355990, 0.5000000000000054401, 9.734124438199387596E-15 ) ) ;
#5993=EDGE_CURVE ( 'NONE', #15249, #13448, #9029, .T. ) ;
#5996=CARTESIAN_POINT ( 'NONE',  ( 198.6508758837858579, -1.438172513732599578, -19.95367855226118436 ) ) ;
#5997=CARTESIAN_POINT ( 'NONE',  ( 219.2049426021622764, 11.20154352970703471, -12.53629070788368338 ) ) ;
#5999=VECTOR ( 'NONE', #3342, 1000.000000000000000 ) ;
#6000=B_SPLINE_CURVE_WITH_KNOTS ( 'NONE', 3,
 ( #2160, #10397, #11802, #3628 ),
 .UNSPECIFIED., .F., .F.,
 ( 4, 4 ),
 ( 1.854400302564232594E-06, 0.0008558401382852200449 ),
 .UNSPECIFIED. ) ;
#6001=VERTEX_POINT ( 'NONE', #10293 ) ;
#6002=ORIENTED_EDGE ( 'NONE', *, *, #5727, .T. ) ;
#6007=VERTEX_POINT ( 'NONE', #15530 ) ;
#6013=B_SPLINE_CURVE_WITH_KNOTS ( 'NONE', 3,
 ( #5261, #13239, #1998, #19686 ),
 .UNSPECIFIED., .F., .F.,
 ( 4, 4 ),
 ( 0.0001336956365395343524, 0.0008063464285820690254 ),
 .UNSPECIFIED. ) ;
#6014=ORIENTED_EDGE ( 'NONE', *, *, #12550, .F. ) ;
#6015=ORIENTED_EDGE ( 'NONE', *, *, #5768, .F. ) ;
#6018=ADVANCED_FACE ( 'NONE', ( #3733 ), #11557, .T. ) ;
#6027=DIRECTION ( 'NONE',  ( -0.5943026915289653100, -0.3431208189343725179, -0.7273736415730454041 ) ) ;
#6030=CARTESIAN_POINT ( 'NONE',  ( 208.4761278624580711, 5.007259451653140125, -14.00000000000005507 ) ) ;
#6031=DIRECTION ( 'NONE',  ( 0.8660254037844355990, 0.5000000000000054401, -2.642119490368404866E-15 ) ) ;
#6033=VERTEX_POINT ( 'NONE', #7433 ) ;
#6035=EDGE_CURVE ( 'NONE', #12385, #9708, #4147, .T. ) ;
#6036=ORIENTED_EDGE ( 'NONE', *, *, #20170, .F. ) ;
#6038=CIRCLE ( 'NONE', #13851, 11.98469917212512215 ) ;
#6039=ORIENTED_EDGE ( 'NONE', *, *, #7836, .T. ) ;
#6041=LINE ( 'NONE', #1082, #13743 ) ;
#6044=LINE ( 'NONE', #20258, #10261 ) ;
#6047=CARTESIAN_POINT ( 'NONE',  ( 196.1289531908403490, 19.26747385478372721, -2.044871543906938705 ) ) ;
#6049=VECTOR ( 'NONE', #14453, 1000.000000000000114 ) ;
#6055=CARTESIAN_POINT ( 'NONE',  ( 210.6527207509366519, 17.03810123488167605, -3.480441514389755575 ) ) ;
#6057=CARTESIAN_POINT ( 'NONE',  ( 195.4946457851292507, 4.162584655573419390, -16.75125533358848884 ) ) ;
#6061=ORIENTED_EDGE ( 'NONE', *, *, #561, .F. ) ;
#6064=AXIS2_PLACEMENT_3D ( 'NONE', #2080, #14820, #6508 ) ;
#6068=CARTESIAN_POINT ( 'NONE',  ( 208.8107687779841228, 4.427644383670616079, -14.00000000000005507 ) ) ;
#6069=CARTESIAN_POINT ( 'NONE',  ( 196.7914626300884322, 9.035300127502988943, -22.62267072728657169 ) ) ;
#6080=VECTOR ( 'NONE', #2636, 1000.000000000000227 ) ;
#6082=ORIENTED_EDGE ( 'NONE', *, *, #17593, .T. ) ;
#6084=B_SPLINE_CURVE_WITH_KNOTS ( 'NONE', 3,
 ( #19301, #19403, #11140, #19199 ),
 .UNSPECIFIED., .F., .F.,
 ( 4, 4 ),
 ( 2.916652380847781525E-07, 0.0006729424572906142791 ),
 .UNSPECIFIED. ) ;
#6087=LINE ( 'NONE', #15464, #2474 ) ;
#6090=VECTOR ( 'NONE', #18060, 1000.000000000000227 ) ;
#6092=EDGE_CURVE ( 'NONE', #18827, #13693, #15964, .T. ) ;
#6095=AXIS2_PLACEMENT_3D ( 'NONE', #15016, #19850, #5216 ) ;
#6096=FACE_OUTER_BOUND ( 'NONE', #5304, .T. ) ;
#6097=AXIS2_PLACEMENT_3D ( 'NONE', #3691, #16221, #1697 ) ;
#6100=DIRECTION ( 'NONE',  ( 0.8660254037844355990, 0.5000000000000054401, 0.000000000000000000 ) ) ;
#6102=AXIS2_PLACEMENT_3D ( 'NONE', #17621, #11145, #1405 ) ;
#6104=VERTEX_POINT ( 'NONE', #10947 ) ;
#6105=ORIENTED_EDGE ( 'NONE', *, *, #6263, .T. ) ;
#6106=AXIS2_PLACEMENT_3D ( 'NONE', #17372, #2853, #9288 ) ;
#6107=FACE_OUTER_BOUND ( 'NONE', #16086, .T. ) ;
#6108=CARTESIAN_POINT ( 'NONE',  ( 198.1555906521723784, 9.822879808262255708, -2.579136038830115218 ) ) ;
#6113=DIRECTION ( 'NONE',  ( 0.5000000000000054401, -0.8660254037844354880, 0.000000000000000000 ) ) ;
#6120=EDGE_LOOP ( 'NONE', ( #15718, #18928, #1167, #18298 ) ) ;
#6123=CARTESIAN_POINT ( 'NONE',  ( 194.9230649354363152, 18.57125394591359679, -2.551678190571418092 ) ) ;
#6125=CARTESIAN_POINT ( 'NONE',  ( 209.9477407942357843, 12.50708294970442402, -13.58165309559974254 ) ) ;
#6133=FACE_OUTER_BOUND ( 'NONE', #4442, .T. ) ;
#6137=CARTESIAN_POINT ( 'NONE',  ( 214.5332756341045979, 19.27854064128383982, -18.44761907388206978 ) ) ;
#6141=EDGE_CURVE ( 'NONE', #18407, #19279, #20475, .T. ) ;
#6145=CONICAL_SURFACE ( 'NONE', #3108, 10.85470691220533190, 0.8171114040043576665 ) ;
#6146=ADVANCED_FACE ( 'NONE', ( #12545 ), #5946, .F. ) ;
#6148=DIRECTION ( 'NONE',  ( -0.1997192025788217806, -0.1153079353712217758, -0.9730448705798236952 ) ) ;
#6151=VECTOR ( 'NONE', #3844, 1000.000000000000227 ) ;
#6157=EDGE_CURVE ( 'NONE', #19244, #19592, #9554, .T. ) ;
#6158=EDGE_CURVE ( 'NONE', #8779, #9213, #19214, .T. ) ;
#6160=DIRECTION ( 'NONE',  ( 0.5000000000000051070, -0.8660254037844355990, -4.163336342344335178E-17 ) ) ;
#6163=DIRECTION ( 'NONE',  ( -0.1005394128318083530, -0.05804645706261224447, 0.9932383577419438003 ) ) ;
#6166=ORIENTED_EDGE ( 'NONE', *, *, #6799, .F. ) ;
#6169=DIRECTION ( 'NONE',  ( 0.1997192025788092906, 0.1153079353712144900, -0.9730448705798270259 ) ) ;
#6170=CARTESIAN_POINT ( 'NONE',  ( 208.8107687779841228, 4.427644383670616079, -14.00000000000005507 ) ) ;
#6171=DIRECTION ( 'NONE',  ( -0.5000000000000049960, 0.8660254037844358210, -0.000000000000000000 ) ) ;
#6173=VERTEX_POINT ( 'NONE', #9335 ) ;
#6174=VERTEX_POINT ( 'NONE', #12445 ) ;
#6180=LINE ( 'NONE', #12768, #1920 ) ;
#6184=ORIENTED_EDGE ( 'NONE', *, *, #1593, .F. ) ;
#6188=DIRECTION ( 'NONE',  ( -0.8660254037844355990, -0.5000000000000054401, -9.734124438199387596E-15 ) ) ;
#6190=PLANE ( 'NONE',  #19624 ) ;
#6197=DIRECTION ( 'NONE',  ( 0.9367698044638387289, 0.000000000000000000, -0.3499461864984122483 ) ) ;
#6199=CARTESIAN_POINT ( 'NONE',  ( 209.6971420603676677, 12.36239970324706050, -2.990331769139234375 ) ) ;
#6200=CARTESIAN_POINT ( 'NONE',  ( 200.4259095341650152, 0.1018498810115307518, -6.098918798390397633 ) ) ;
#6202=CIRCLE ( 'NONE', #10597, 12.47473710546057823 ) ;
#6203=ORIENTED_EDGE ( 'NONE', *, *, #6679, .F. ) ;
#6204=LINE ( 'NONE', #14506, #2700 ) ;
#6205=CYLINDRICAL_SURFACE ( 'NONE', #5472, 12.47473710546057646 ) ;
#6208=CARTESIAN_POINT ( 'NONE',  ( 207.4817114093494297, 25.82199186828477266, -22.03054070023868860 ) ) ;
#6210=EDGE_CURVE ( 'NONE', #15437, #1522, #2999, .T. ) ;
#6211=ORIENTED_EDGE ( 'NONE', *, *, #6646, .F. ) ;
#6217=VERTEX_POINT ( 'NONE', #19611 ) ;
#6218=ORIENTED_EDGE ( 'NONE', *, *, #6755, .F. ) ;
#6232=CARTESIAN_POINT ( 'NONE',  ( 203.7027818574982518, 1.478546760110915903, -24.25943249057081630 ) ) ;
#6246=CARTESIAN_POINT ( 'NONE',  ( 198.5374064076044078, -1.503684146350823703, -15.40190399002796440 ) ) ;
#6247=ORIENTED_EDGE ( 'NONE', *, *, #4998, .T. ) ;
#6250=DIRECTION ( 'NONE',  ( -0.8660254037844357100, -0.5000000000000051070, 0.000000000000000000 ) ) ;
#6256=DIRECTION ( 'NONE',  ( 0.5000000000000054401, -0.8660254037844353769, 2.220446049250312588E-16 ) ) ;
#6257=DIRECTION ( 'NONE',  ( -0.5000000000000053291, 0.8660254037844354880, 0.000000000000000000 ) ) ;
#6261=CIRCLE ( 'NONE', #7963, 12.47473710546057823 ) ;
#6263=EDGE_CURVE ( 'NONE', #18877, #6425, #12168, .T. ) ;
#6265=CARTESIAN_POINT ( 'NONE',  ( 196.4296119619006618, 4.702387629415611947, -19.29168348739290195 ) ) ;
#6274=EDGE_LOOP ( 'NONE', ( #6568, #19367, #8343, #6623, #16757, #13496 ) ) ;
#6277=CONICAL_SURFACE ( 'NONE', #5594, 10.85470691220533190, 0.8171114040043576665 ) ;
#6279=CARTESIAN_POINT ( 'NONE',  ( 195.3740178925880002, 3.738913527986503560, -11.16670872502617584 ) ) ;
#6281=ORIENTED_EDGE ( 'NONE', *, *, #13154, .T. ) ;
#6282=CARTESIAN_POINT ( 'NONE',  ( 208.0983737146324870, 5.661548828456886895, -14.00000000000005507 ) ) ;
#6283=EDGE_CURVE ( 'NONE', #10758, #2805, #13930, .T. ) ;
#6285=CARTESIAN_POINT ( 'NONE',  ( 199.6917776511935472, -0.3220013592427101723, -7.237580838289900953 ) ) ;
#6286=DIRECTION ( 'NONE',  ( 0.5000000000000054401, -0.8660254037844354880, 0.000000000000000000 ) ) ;
#6288=ADVANCED_FACE ( 'NONE', ( #19508 ), #3401, .F. ) ;
#6291=VECTOR ( 'NONE', #6854, 1000.000000000000114 ) ;
#6293=AXIS2_PLACEMENT_3D ( 'NONE', #6751, #2116, #421 ) ;
#6295=EDGE_CURVE ( 'NONE', #13147, #8980, #4860, .T. ) ;
#6296=VERTEX_POINT ( 'NONE', #10061 ) ;
#6298=CARTESIAN_POINT ( 'NONE',  ( 205.5965122587965084, 9.994899983462953941, -14.00000000000005507 ) ) ;
#6302=EDGE_CURVE ( 'NONE', #4567, #15885, #9658, .T. ) ;
#6304=AXIS2_PLACEMENT_3D ( 'NONE', #12998, #12791, #4825 ) ;
#6308=EDGE_CURVE ( 'NONE', #13300, #694, #17331, .T. ) ;
#6309=B_SPLINE_CURVE_WITH_KNOTS ( 'NONE', 3,
 ( #12533, #14141, #2885, #5722 ),
 .UNSPECIFIED., .F., .F.,
 ( 4, 4 ),
 ( 3.854193985120393637E-07, 0.0008543711573788317915 ),
 .UNSPECIFIED. ) ;
#6314=VERTEX_POINT ( 'NONE', #4031 ) ;
#6321=CARTESIAN_POINT ( 'NONE',  ( 195.2889461848653525, 4.043823935988862139, -15.40420431385919464 ) ) ;
#6324=ORIENTED_EDGE ( 'NONE', *, *, #11708, .F. ) ;
#6327=B_SPLINE_CURVE_WITH_KNOTS ( 'NONE', 3,
 ( #7882, #17657, #20496, #9574 ),
 .UNSPECIFIED., .F., .F.,
 ( 4, 4 ),
 ( 9.323472578458188095E-06, 0.0008633092105634442145 ),
 .UNSPECIFIED. ) ;
#6329=LINE ( 'NONE', #12827, #7071 ) ;
#6334=VERTEX_POINT ( 'NONE', #15406 ) ;
#6338=CARTESIAN_POINT ( 'NONE',  ( 195.7881298832096775, 4.155017874419543844, -18.15810777665835474 ) ) ;
#6342=ADVANCED_FACE ( 'NONE', ( #5291 ), #16994, .T. ) ;
#6346=B_SPLINE_CURVE_WITH_KNOTS ( 'NONE', 3,
 ( #11654, #19797, #303, #13351 ),
 .UNSPECIFIED., .F., .F.,
 ( 4, 4 ),
 ( 2.759414894645841475E-07, 0.0006729267335475704655 ),
 .UNSPECIFIED. ) ;
#6347=VECTOR ( 'NONE', #4577, 1000.000000000000114 ) ;
#6353=CARTESIAN_POINT ( 'NONE',  ( 205.8264633344831225, 9.596613037118636669, -14.00000000000005507 ) ) ;
#6361=DIRECTION ( 'NONE',  ( -0.5000000000000054401, 0.8660254037844354880, -0.000000000000000000 ) ) ;
#6377=CARTESIAN_POINT ( 'NONE',  ( 196.8850361132133173, 4.788316981587917631, -20.67833249884100510 ) ) ;
#6378=EDGE_CURVE ( 'NONE', #18388, #18856, #19821, .T. ) ;
#6390=ORIENTED_EDGE ( 'NONE', *, *, #17809, .T. ) ;
#6392=EDGE_CURVE ( 'NONE', #3291, #3585, #5397, .T. ) ;
#6395=DIRECTION ( 'NONE',  ( 0.3430151393149145078, 0.1980398830195854720, 0.9182161068802695558 ) ) ;
#6396=DIRECTION ( 'NONE',  ( -0.8660254037844349329, -0.5000000000000064393, 0.000000000000000000 ) ) ;
#6401=ORIENTED_EDGE ( 'NONE', *, *, #12785, .F. ) ;
#6403=EDGE_CURVE ( 'NONE', #10058, #3882, #20247, .T. ) ;
#6405=ADVANCED_FACE ( 'NONE', ( #15091 ), #19685, .T. ) ;
#6413=ORIENTED_EDGE ( 'NONE', *, *, #17184, .T. ) ;
#6414=ORIENTED_EDGE ( 'NONE', *, *, #10583, .T. ) ;
#6416=FACE_OUTER_BOUND ( 'NONE', #9423, .T. ) ;
#6419=ORIENTED_EDGE ( 'NONE', *, *, #10793, .T. ) ;
#6425=VERTEX_POINT ( 'NONE', #6892 ) ;
#6427=ORIENTED_EDGE ( 'NONE', *, *, #12987, .T. ) ;
#6430=AXIS2_PLACEMENT_3D ( 'NONE', #16430, #14860, #13148 ) ;
#6431=LINE ( 'NONE', #11430, #15561 ) ;
#6432=VECTOR ( 'NONE', #17937, 1000.000000000000114 ) ;
#6433=CARTESIAN_POINT ( 'NONE',  ( 209.8909370991932235, 2.556737970610013733, -14.00000000000005507 ) ) ;
#6440=ORIENTED_EDGE ( 'NONE', *, *, #2828, .T. ) ;
#6444=VERTEX_POINT ( 'NONE', #5507 ) ;
#6446=AXIS2_PLACEMENT_3D ( 'NONE', #18293, #3556, #10001 ) ;
#6449=VERTEX_POINT ( 'NONE', #8697 ) ;
#6453=VERTEX_POINT ( 'NONE', #15196 ) ;
#6457=DIRECTION ( 'NONE',  ( 0.2483788854153066994, 0.1434016163555488221, 0.9579895123154877901 ) ) ;
#6461=CARTESIAN_POINT ( 'NONE',  ( 203.7294658059541064, 23.22871929987706707, -14.00000000000005507 ) ) ;
#6463=EDGE_LOOP ( 'NONE', ( #5968, #9389, #2535, #17994, #13596, #19936 ) ) ;
#6465=AXIS2_PLACEMENT_3D ( 'NONE', #20706, #5958, #15747 ) ;
#6467=FACE_OUTER_BOUND ( 'NONE', #11632, .T. ) ;
#6469=VECTOR ( 'NONE', #6171, 1000.000000000000227 ) ;
#6471=CARTESIAN_POINT ( 'NONE',  ( 199.2144802262915846, 21.04890371929339921, -14.00000000000005507 ) ) ;
#6472=DIRECTION ( 'NONE',  ( 0.4758887346169383692, 0.2747544890354036706, -0.8354878114129394850 ) ) ;
#6473=CONICAL_SURFACE ( 'NONE', #11918, 13.07248899748297433, 0.6693469023067423196 ) ;
#6475=ORIENTED_EDGE ( 'NONE', *, *, #9374, .F. ) ;
#6476=CARTESIAN_POINT ( 'NONE',  ( 214.2619155600624481, 14.99787291208556539, -20.59651891138172530 ) ) ;
#6477=ORIENTED_EDGE ( 'NONE', *, *, #1068, .T. ) ;
#6480=ORIENTED_EDGE ( 'NONE', *, *, #15516, .T. ) ;
#6483=AXIS2_PLACEMENT_3D ( 'NONE', #9972, #8822, #7015 ) ;
#6484=CARTESIAN_POINT ( 'NONE',  ( 208.4761278624580711, 5.007259451653140125, -14.00000000000005507 ) ) ;
#6486=CONICAL_SURFACE ( 'NONE', #15670, 4.389613146203297234, 1.047197551196619614 ) ;
#6487=B_SPLINE_CURVE_WITH_KNOTS ( 'NONE', 3,
 ( #2525, #8771, #15372, #10563 ),
 .UNSPECIFIED., .F., .F.,
 ( 4, 4 ),
 ( 2.740756717971691198E-07, 0.0006729248677300605315 ),
 .UNSPECIFIED. ) ;
#6490=FACE_OUTER_BOUND ( 'NONE', #12913, .T. ) ;
#6491=ORIENTED_EDGE ( 'NONE', *, *, #1006, .F. ) ;
#6495=ORIENTED_EDGE ( 'NONE', *, *, #17003, .T. ) ;
#6496=CARTESIAN_POINT ( 'NONE',  ( 209.9464292287906630, 27.24499736481567069, -15.43274561385901400 ) ) ;
#6497=CONICAL_SURFACE ( 'NONE', #19701, 4.999999999999944933, 1.566852922939436121 ) ;
#6506=ORIENTED_EDGE ( 'NONE', *, *, #315, .F. ) ;
#6508=DIRECTION ( 'NONE',  ( 0.8660254037844355990, 0.5000000000000054401, 0.000000000000000000 ) ) ;
#6519=ORIENTED_EDGE ( 'NONE', *, *, #11860, .F. ) ;
#6520=ORIENTED_EDGE ( 'NONE', *, *, #5993, .T. ) ;
#6529=CONICAL_SURFACE ( 'NONE', #472, 13.07248899748297433, 0.6693469023067423196 ) ;
#6533=LINE ( 'NONE', #11647, #14153 ) ;
#6534=FACE_OUTER_BOUND ( 'NONE', #7907, .T. ) ;
#6536=DIRECTION ( 'NONE',  ( 0.5000000000000058842, -0.8660254037844351549, 0.000000000000000000 ) ) ;
#6545=ORIENTED_EDGE ( 'NONE', *, *, #20760, .T. ) ;
#6551=EDGE_CURVE ( 'NONE', #8176, #5372, #14659, .T. ) ;
#6557=ORIENTED_EDGE ( 'NONE', *, *, #8622, .F. ) ;
#6565=LINE ( 'NONE', #13481, #14934 ) ;
#6568=ORIENTED_EDGE ( 'NONE', *, *, #5122, .F. ) ;
#6581=EDGE_CURVE ( 'NONE', #3518, #1818, #18881, .T. ) ;
#6586=CARTESIAN_POINT ( 'NONE',  ( 198.4292936038012840, 5.502877782304041787, -22.95081059697375991 ) ) ;
#6591=CARTESIAN_POINT ( 'NONE',  ( 200.1605181682011221, -0.5665801344454006738, -7.448751785191272567 ) ) ;
#6595=ORIENTED_EDGE ( 'NONE', *, *, #18053, .F. ) ;
#6608=DIRECTION ( 'NONE',  ( 0.5000000000000054401, -0.8660254037844354880, 0.000000000000000000 ) ) ;
#6610=EDGE_CURVE ( 'NONE', #14942, #9307, #18090, .T. ) ;
#6614=ORIENTED_EDGE ( 'NONE', *, *, #8251, .T. ) ;
#6615=AXIS2_PLACEMENT_3D ( 'NONE', #3085, #14446, #10813 ) ;
#6619=AXIS2_PLACEMENT_3D ( 'NONE', #11209, #12911, #19365 ) ;
#6623=ORIENTED_EDGE ( 'NONE', *, *, #4208, .F. ) ;
#6624=ORIENTED_EDGE ( 'NONE', *, *, #14833, .F. ) ;
#6634=EDGE_LOOP ( 'NONE', ( #7373, #5450, #18106, #86 ) ) ;
#6639=EDGE_CURVE ( 'NONE', #8949, #7633, #19874, .T. ) ;
#6641=DIRECTION ( 'NONE',  ( -0.8601696498176567562, -0.4966191788709768962, -0.1160929141252230179 ) ) ;
#6643=CARTESIAN_POINT ( 'NONE',  ( 205.0662616026534693, 10.91332106064940888, -14.00000000000005507 ) ) ;
#6646=EDGE_CURVE ( 'NONE', #1746, #20139, #11431, .T. ) ;
#6656=CARTESIAN_POINT ( 'NONE',  ( 196.7640869814540565, 9.019494789394645551, -5.407152407593843968 ) ) ;
#6657=EDGE_LOOP ( 'NONE', ( #3854, #11901, #8984, #12141 ) ) ;
#6658=EDGE_CURVE ( 'NONE', #9199, #11172, #12834, .T. ) ;
#6662=CARTESIAN_POINT ( 'NONE',  ( 213.0703269268611848, 13.95588231258707701, -22.95081059697398373 ) ) ;
#6669=LINE ( 'NONE', #16442, #12895 ) ;
#6670=DIRECTION ( 'NONE',  ( -0.8660254037844354880, -0.5000000000000055511, 0.000000000000000000 ) ) ;
#6672=EDGE_CURVE ( 'NONE', #15862, #20176, #10167, .T. ) ;
#6679=EDGE_CURVE ( 'NONE', #7529, #1461, #275, .T. ) ;
#6680=VECTOR ( 'NONE', #17383, 1000.000000000000227 ) ;
#6682=ORIENTED_EDGE ( 'NONE', *, *, #13159, .T. ) ;
#6683=ORIENTED_EDGE ( 'NONE', *, *, #4219, .F. ) ;
#6685=DIRECTION ( 'NONE',  ( -0.8660254037844357100, -0.5000000000000049960, 0.000000000000000000 ) ) ;
#6691=ORIENTED_EDGE ( 'NONE', *, *, #2234, .T. ) ;
#6693=CARTESIAN_POINT ( 'NONE',  ( 196.7929107858857094, 4.381089041447214782, -20.84195174293567376 ) ) ;
#6696=DIRECTION ( 'NONE',  ( -0.7235536692358652822, -0.4177439057064742944, -0.5495089780708012350 ) ) ;
#6701=CARTESIAN_POINT ( 'NONE',  ( 200.2378745322256464, -0.5219184168523266498, -7.515250618841284869 ) ) ;
#6707=DIRECTION ( 'NONE',  ( -0.8660254037844355990, -0.5000000000000055511, 0.000000000000000000 ) ) ;
#6711=LINE ( 'NONE', #6125, #18428 ) ;
#6720=CARTESIAN_POINT ( 'NONE',  ( 201.0270608673618256, -0.06628147382068544369, -4.392917125964748593 ) ) ;
#6722=LINE ( 'NONE', #8544, #10310 ) ;
#6723=ORIENTED_EDGE ( 'NONE', *, *, #16286, .F. ) ;
#6725=B_SPLINE_CURVE_WITH_KNOTS ( 'NONE', 3,
 ( #19881, #13649, #15253, #2402 ),
 .UNSPECIFIED., .F., .F.,
 ( 4, 4 ),
 ( 7.737990982947961127E-05, 0.0009313656478097689061 ),
 .UNSPECIFIED. ) ;
#6728=CARTESIAN_POINT ( 'NONE',  ( 204.2095024616932051, 2.543922127990230209, -25.46066938576250038 ) ) ;
#6730=ORIENTED_EDGE ( 'NONE', *, *, #4070, .F. ) ;
#6738=ORIENTED_EDGE ( 'NONE', *, *, #17861, .F. ) ;
#6743=CARTESIAN_POINT ( 'NONE',  ( 212.9202825050182923, 6.800273240212296955, -24.96223045542567931 ) ) ;
#6744=ADVANCED_FACE ( 'NONE', ( #19666 ), #3086, .T. ) ;
#6748=AXIS2_PLACEMENT_3D ( 'NONE', #11541, #13042, #19693 ) ;
#6751=CARTESIAN_POINT ( 'NONE',  ( 208.4761278624580711, 5.007259451653140125, -14.00000000000005507 ) ) ;
#6755=EDGE_CURVE ( 'NONE', #2132, #19734, #19773, .T. ) ;
#6758=ADVANCED_FACE ( 'NONE', ( #15040, #9525 ), #6939, .F. ) ;
#6767=B_SPLINE_CURVE_WITH_KNOTS ( 'NONE', 3,
 ( #1359, #20533, #1048, #19166 ),
 .UNSPECIFIED., .F., .F.,
 ( 4, 4 ),
 ( 0.0001125711301185649063, 0.0007852219221655419622 ),
 .UNSPECIFIED. ) ;
#6769=CARTESIAN_POINT ( 'NONE',  ( 210.5941221282246545, 5.457263920492195552, -2.233628351993232730 ) ) ;
#6773=ADVANCED_FACE ( 'NONE', ( #10106 ), #17649, .T. ) ;
#6777=DIRECTION ( 'NONE',  ( -0.3430151393149145078, -0.1980398830195854720, -0.9182161068802695558 ) ) ;
#6778=CARTESIAN_POINT ( 'NONE',  ( 198.2719933611348040, -1.399321216369431298, -12.59769448420646043 ) ) ;
#6781=CIRCLE ( 'NONE', #11205, 11.98469917212512215 ) ;
#6783=DIRECTION ( 'NONE',  ( -0.8660254037844357100, -0.5000000000000051070, 0.000000000000000000 ) ) ;
#6789=EDGE_CURVE ( 'NONE', #10758, #5372, #695, .T. ) ;
#6790=ORIENTED_EDGE ( 'NONE', *, *, #7718, .F. ) ;
#6791=ORIENTED_EDGE ( 'NONE', *, *, #15669, .T. ) ;
#6792=CIRCLE ( 'NONE', #9172, 7.960520131757803597 ) ;
#6794=ORIENTED_EDGE ( 'NONE', *, *, #19895, .F. ) ;
#6797=B_SPLINE_CURVE_WITH_KNOTS ( 'NONE', 3,
 ( #6907, #13392, #2362, #5414 ),
 .UNSPECIFIED., .F., .F.,
 ( 4, 4 ),
 ( 7.495004023226334094E-05, 0.0007476008322856125647 ),
 .UNSPECIFIED. ) ;
#6798=CARTESIAN_POINT ( 'NONE',  ( 208.5840039954387066, 11.71972914181512060, -2.522505859538486828 ) ) ;
#6799=EDGE_CURVE ( 'NONE', #2132, #14589, #6781, .T. ) ;
#6800=VERTEX_POINT ( 'NONE', #19870 ) ;
#6806=AXIS2_PLACEMENT_3D ( 'NONE', #13311, #8523, #13204 ) ;
#6807=CARTESIAN_POINT ( 'NONE',  ( 208.4761278624580711, 5.007259451653140125, -14.00000000000005507 ) ) ;
#6811=FACE_OUTER_BOUND ( 'NONE', #17568, .T. ) ;
#6813=EDGE_LOOP ( 'NONE', ( #11508, #5831, #13834, #11138, #18127, #11633 ) ) ;
#6815=CARTESIAN_POINT ( 'NONE',  ( 207.4656388362385826, 11.07404071609863117, -10.98795432269212391 ) ) ;
#6821=ORIENTED_EDGE ( 'NONE', *, *, #16319, .F. ) ;
#6824=CARTESIAN_POINT ( 'NONE',  ( 208.8107687779841228, 4.427644383670616079, -14.00000000000005507 ) ) ;
#6834=EDGE_LOOP ( 'NONE', ( #16517, #19878, #13153, #17698 ) ) ;
#6838=DIRECTION ( 'NONE',  ( 0.5000000000000049960, -0.8660254037844358210, 0.000000000000000000 ) ) ;
#6841=VECTOR ( 'NONE', #5418, 1000.000000000000114 ) ;
#6845=ORIENTED_EDGE ( 'NONE', *, *, #18489, .T. ) ;
#6848=FACE_OUTER_BOUND ( 'NONE', #630, .T. ) ;
#6849=CARTESIAN_POINT ( 'NONE',  ( 205.8264633344831225, 9.596613037118636669, -14.00000000000005507 ) ) ;
#6854=DIRECTION ( 'NONE',  ( 0.8296432542242783148, 0.4789947561577510560, 0.2868032327110804358 ) ) ;
#6859=B_SPLINE_CURVE_WITH_KNOTS ( 'NONE', 3,
 ( #68, #163, #8306, #4827 ),
 .UNSPECIFIED., .F., .F.,
 ( 4, 4 ),
 ( 3.603418170169278305E-07, 0.0008543460797983053016 ),
 .UNSPECIFIED. ) ;
#6861=EDGE_CURVE ( 'NONE', #15101, #16061, #2187, .T. ) ;
#6865=DIRECTION ( 'NONE',  ( -0.8660254037844357100, -0.5000000000000051070, 0.000000000000000000 ) ) ;
#6866=FACE_OUTER_BOUND ( 'NONE', #4067, .T. ) ;
#6868=VERTEX_POINT ( 'NONE', #9054 ) ;
#6877=CARTESIAN_POINT ( 'NONE',  ( 193.8427921854145097, 7.332884452518919183, -11.24974199967268262 ) ) ;
#6879=AXIS2_PLACEMENT_3D ( 'NONE', #8920, #15520, #13914 ) ;
#6881=DIRECTION ( 'NONE',  ( 0.7951984747223579397, 0.4591080534401397184, -0.3960797660391670583 ) ) ;
#6882=AXIS2_PLACEMENT_3D ( 'NONE', #14877, #5506, #5607 ) ;
#6886=EDGE_CURVE ( 'NONE', #20843, #18617, #3199, .T. ) ;
#6888=LINE ( 'NONE', #19816, #12285 ) ;
#6889=EDGE_LOOP ( 'NONE', ( #18345, #11274, #20774, #266 ) ) ;
#6892=CARTESIAN_POINT ( 'NONE',  ( 197.7473131227538659, -1.187024626400782656, -12.53629070788332989 ) ) ;
#6899=ORIENTED_EDGE ( 'NONE', *, *, #20447, .F. ) ;
#6901=ADVANCED_FACE ( 'NONE', ( #14462 ), #20293, .F. ) ;
#6906=CARTESIAN_POINT ( 'NONE',  ( 198.4513784989219971, 5.692645179619979068, -5.166194743381255172 ) ) ;
#6907=CARTESIAN_POINT ( 'NONE',  ( 196.3264911765913041, 4.642850816258196289, -8.609703802792473937 ) ) ;
#6914=ORIENTED_EDGE ( 'NONE', *, *, #1276, .F. ) ;
#6920=EDGE_LOOP ( 'NONE', ( #8863, #2231, #7508, #5243 ) ) ;
#6926=AXIS2_PLACEMENT_3D ( 'NONE', #356, #15105, #3727 ) ;
#6929=ORIENTED_EDGE ( 'NONE', *, *, #13487, .F. ) ;
#6934=DIRECTION ( 'NONE',  ( 0.5000000000000054401, -0.8660254037844354880, 0.000000000000000000 ) ) ;
#6938=EDGE_CURVE ( 'NONE', #15862, #3973, #9155, .T. ) ;
#6939=PLANE ( 'NONE',  #5773 ) ;
#6940=DIRECTION ( 'NONE',  ( -0.5000000000000051070, 0.8660254037844359321, -0.000000000000000000 ) ) ;
#6942=EDGE_CURVE ( 'NONE', #17033, #6453, #1342, .T. ) ;
#6943=ORIENTED_EDGE ( 'NONE', *, *, #13888, .T. ) ;
#6950=ORIENTED_EDGE ( 'NONE', *, *, #8206, .F. ) ;
#6951=ORIENTED_EDGE ( 'NONE', *, *, #4235, .T. ) ;
#6955=ORIENTED_EDGE ( 'NONE', *, *, #15291, .T. ) ;
#6956=EDGE_CURVE ( 'NONE', #8118, #11210, #20497, .T. ) ;
#6958=DIRECTION ( 'NONE',  ( -0.8660254037844354880, -0.5000000000000055511, 0.000000000000000000 ) ) ;
#6960=AXIS2_PLACEMENT_3D ( 'NONE', #1599, #2435, #2544 ) ;
#6961=AXIS2_PLACEMENT_3D ( 'NONE', #17916, #20768, #12627 ) ;
#6964=DIRECTION ( 'NONE',  ( 0.6946590618905411629, 0.4010615963775225890, -0.5971585917027958379 ) ) ;
#6966=DIRECTION ( 'NONE',  ( 0.7739085681710337061, 0.4468163201617106339, -0.4487991802004634989 ) ) ;
#6968=CARTESIAN_POINT ( 'NONE',  ( 188.7053703664960551, 14.98146631279701602, -16.89203719259486647 ) ) ;
#6970=ORIENTED_EDGE ( 'NONE', *, *, #9586, .F. ) ;
#6976=CIRCLE ( 'NONE', #12745, 11.94520687646042667 ) ;
#6977=CARTESIAN_POINT ( 'NONE',  ( 218.5623757963967080, 10.31533654458964477, -18.15054426878737104 ) ) ;
#6978=CIRCLE ( 'NONE', #13428, 11.94520687646042667 ) ;
#6980=B_SPLINE_CURVE_WITH_KNOTS ( 'NONE', 3,
 ( #5338, #13427, #2084, #16597 ),
 .UNSPECIFIED., .F., .F.,
 ( 4, 4 ),
 ( 2.451646831110292017E-05, 0.0008785022062956360364 ),
 .UNSPECIFIED. ) ;
#6986=CARTESIAN_POINT ( 'NONE',  ( 205.0662616026534693, 10.91332106064940888, -14.00000000000005507 ) ) ;
#6989=DIRECTION ( 'NONE',  ( 0.5000000000000054401, -0.8660254037844354880, 0.000000000000000000 ) ) ;
#6991=CARTESIAN_POINT ( 'NONE',  ( 213.6457381091975662, 14.64212269496015750, -5.449056122693788140 ) ) ;
#6992=ORIENTED_EDGE ( 'NONE', *, *, #6672, .F. ) ;
#6994=PLANE ( 'NONE',  #5867 ) ;
#6996=ORIENTED_EDGE ( 'NONE', *, *, #18939, .T. ) ;
#6999=PLANE ( 'NONE',  #2225 ) ;
#7004=CIRCLE ( 'NONE', #4646, 11.98469917212512215 ) ;
#7006=VERTEX_POINT ( 'NONE', #12964 ) ;
#7007=CONICAL_SURFACE ( 'NONE', #13129, 10.85470691220533190, 0.8171114040043576665 ) ;
#7009=ORIENTED_EDGE ( 'NONE', *, *, #14237, .F. ) ;
#7013=CARTESIAN_POINT ( 'NONE',  ( 218.1074424443701503, 10.31028766640382344, -8.485309299592367793 ) ) ;
#7015=DIRECTION ( 'NONE',  ( 0.5000000000000053291, -0.8660254037844354880, 0.000000000000000000 ) ) ;
#7016=ADVANCED_FACE ( 'NONE', ( #19411 ), #10538, .T. ) ;
#7017=CARTESIAN_POINT ( 'NONE',  ( 203.2336538649942668, 12.75470097114692969, -25.81526893633797570 ) ) ;
#7022=CONICAL_SURFACE ( 'NONE', #16524, 10.85470691220533190, 0.8171114040043576665 ) ;
#7031=CARTESIAN_POINT ( 'NONE',  ( 202.6756539743620920, 0.8855342002901112064, -23.47937149798923073 ) ) ;
#7033=CARTESIAN_POINT ( 'NONE',  ( 209.7467543128910847, 12.39104335059658091, -13.30618937499484922 ) ) ;
#7038=ORIENTED_EDGE ( 'NONE', *, *, #14627, .F. ) ;
#7040=EDGE_CURVE ( 'NONE', #4535, #12762, #3608, .T. ) ;
#7042=DIRECTION ( 'NONE',  ( -0.6299240516454520655, -0.3636868207865263658, 0.6862416378687372642 ) ) ;
#7049=DIRECTION ( 'NONE',  ( -0.3886714912512297393, -0.2243995901002339699, -0.8936326403234117199 ) ) ;
#7050=CARTESIAN_POINT ( 'NONE',  ( 208.8107687779841228, 4.427644383670616079, -14.00000000000005507 ) ) ;
#7056=CARTESIAN_POINT ( 'NONE',  ( 212.4556053886519749, 4.037449897911128183, -14.00000000000005507 ) ) ;
#7057=ADVANCED_FACE ( 'NONE', ( #19506 ), #3302, .F. ) ;
#7059=ORIENTED_EDGE ( 'NONE', *, *, #18100, .F. ) ;
#7071=VECTOR ( 'NONE', #1583, 1000.000000000000000 ) ;
#7075=DIRECTION ( 'NONE',  ( 0.8660254037844355990, 0.5000000000000054401, 0.000000000000000000 ) ) ;
#7079=CARTESIAN_POINT ( 'NONE',  ( 209.3909370991932235, 3.422763374394450775, -14.00000000000005507 ) ) ;
#7083=ORIENTED_EDGE ( 'NONE', *, *, #7992, .T. ) ;
#7084=CIRCLE ( 'NONE', #5051, 11.98469917212512215 ) ;
#7087=B_SPLINE_CURVE_WITH_KNOTS ( 'NONE', 3,
 ( #11423, #17789, #19376, #3361 ),
 .UNSPECIFIED., .F., .F.,
 ( 4, 4 ),
 ( 0.0001237509890165146265, 0.0007964017810610974930 ),
 .UNSPECIFIED. ) ;
#7090=EDGE_CURVE ( 'NONE', #19498, #18324, #6565, .T. ) ;
#7099=CARTESIAN_POINT ( 'NONE',  ( 218.6326489791658503, 10.87112965241456841, -18.25196083293883120 ) ) ;
#7100=EDGE_LOOP ( 'NONE', ( #16429, #10555, #4427, #12723 ) ) ;
#7107=VERTEX_POINT ( 'NONE', #18242 ) ;
#7108=DIRECTION ( 'NONE',  ( -0.5000000000000053291, 0.8660254037844354880, 0.000000000000000000 ) ) ;
#7111=ORIENTED_EDGE ( 'NONE', *, *, #15060, .F. ) ;
#7113=AXIS2_PLACEMENT_3D ( 'NONE', #13507, #19954, #4275 ) ;
#7118=CARTESIAN_POINT ( 'NONE',  ( 199.2144802262915846, 21.04890371929339921, -14.00000000000005507 ) ) ;
#7120=CARTESIAN_POINT ( 'NONE',  ( 200.8534188064670900, 11.38047161937165974, -2.669358488461094137 ) ) ;
#7122=CARTESIAN_POINT ( 'NONE',  ( 207.8344881237125890, 4.636808575765666518, -26.45271578590683248 ) ) ;
#7125=CARTESIAN_POINT ( 'NONE',  ( 198.8278877809574965, -0.5631545566074300790, -19.61257667712936126 ) ) ;
#7126=ORIENTED_EDGE ( 'NONE', *, *, #18283, .F. ) ;
#7133=AXIS2_PLACEMENT_3D ( 'NONE', #10973, #7984, #12680 ) ;
#7136=DIRECTION ( 'NONE',  ( -0.8660254037844355990, -0.5000000000000053291, 0.000000000000000000 ) ) ;
#7142=AXIS2_PLACEMENT_3D ( 'NONE', #7994, #12996, #9473 ) ;
#7143=CARTESIAN_POINT ( 'NONE',  ( 205.5965122587965084, 9.994899983462953941, -14.00000000000005507 ) ) ;
#7144=ORIENTED_EDGE ( 'NONE', *, *, #6551, .T. ) ;
#7152=CARTESIAN_POINT ( 'NONE',  ( 198.7478178127443016, -1.382203064952688409, -11.23040475586387821 ) ) ;
#7156=ORIENTED_EDGE ( 'NONE', *, *, #39, .F. ) ;
#7157=VERTEX_POINT ( 'NONE', #19717 ) ;
#7167=CARTESIAN_POINT ( 'NONE',  ( 208.9378540577313004, 11.39297530874010000, -25.94618751764496878 ) ) ;
#7170=ORIENTED_EDGE ( 'NONE', *, *, #9457, .F. ) ;
#7173=CARTESIAN_POINT ( 'NONE',  ( 204.9818247258934321, 9.640009970873842704, -2.036337243043272238 ) ) ;
#7175=DIRECTION ( 'NONE',  ( -0.8660254037844354880, -0.5000000000000055511, 0.000000000000000000 ) ) ;
#7176=VECTOR ( 'NONE', #3842, 999.9999999999998863 ) ;
#7177=EDGE_CURVE ( 'NONE', #844, #19176, #6669, .T. ) ;
#7183=EDGE_CURVE ( 'NONE', #11306, #3323, #11674, .T. ) ;
#7184=CARTESIAN_POINT ( 'NONE',  ( 201.7640869814541134, 0.3592407515502875626, -5.407152407593845744 ) ) ;
#7188=ORIENTED_EDGE ( 'NONE', *, *, #20111, .T. ) ;
#7203=LINE ( 'NONE', #4243, #2348 ) ;
#7205=DIRECTION ( 'NONE',  ( 0.8660254037844355990, 0.5000000000000054401, 4.449885457462577074E-15 ) ) ;
#7206=CARTESIAN_POINT ( 'NONE',  ( 199.1867014016590076, -1.128813506749884343, -18.06789442459577799 ) ) ;
#7207=EDGE_CURVE ( 'NONE', #2978, #12472, #10849, .T. ) ;
#7208=EDGE_CURVE ( 'NONE', #2903, #772, #4069, .T. ) ;
#7210=ORIENTED_EDGE ( 'NONE', *, *, #8358, .T. ) ;
#7214=ORIENTED_EDGE ( 'NONE', *, *, #20234, .T. ) ;
#7216=EDGE_CURVE ( 'NONE', #12547, #14158, #5822, .T. ) ;
#7220=AXIS2_PLACEMENT_3D ( 'NONE', #3041, #19157, #14510 ) ;
#7228=ORIENTED_EDGE ( 'NONE', *, *, #15109, .F. ) ;
#7229=CARTESIAN_POINT ( 'NONE',  ( 209.3577037357181894, 3.480325248439696040, -14.00000000000005507 ) ) ;
#7249=CIRCLE ( 'NONE', #148, 12.47473710546057823 ) ;
#7251=ORIENTED_EDGE ( 'NONE', *, *, #10984, .T. ) ;
#7264=ORIENTED_EDGE ( 'NONE', *, *, #12783, .T. ) ;
#7269=EDGE_CURVE ( 'NONE', #3223, #10497, #2664, .T. ) ;
#7271=FACE_OUTER_BOUND ( 'NONE', #157, .T. ) ;
#7272=CIRCLE ( 'NONE', #12047, 11.94520687646042667 ) ;
#7273=DIRECTION ( 'NONE',  ( -0.9294597282054694043, 0.3689235878121848722, 0.000000000000000000 ) ) ;
#7277=EDGE_CURVE ( 'NONE', #5590, #4064, #2315, .T. ) ;
#7279=ORIENTED_EDGE ( 'NONE', *, *, #20794, .F. ) ;
#7282=FACE_OUTER_BOUND ( 'NONE', #13044, .T. ) ;
#7288=VERTEX_POINT ( 'NONE', #20351 ) ;
#7289=DIRECTION ( 'NONE',  ( -0.8660254037844357100, -0.5000000000000051070, 0.000000000000000000 ) ) ;
#7299=DIRECTION ( 'NONE',  ( -0.5000000000000051070, 0.8660254037844359321, -0.000000000000000000 ) ) ;
#7301=CARTESIAN_POINT ( 'NONE',  ( 209.6893306017078373, 12.35788975548706148, -12.44595276995722877 ) ) ;
#7306=CIRCLE ( 'NONE', #17807, 1.000000000000000888 ) ;
#7319=AXIS2_PLACEMENT_3D ( 'NONE', #12459, #18917, #7975 ) ;
#7320=CARTESIAN_POINT ( 'NONE',  ( 196.1523298472990007, 4.542298725908849200, -18.76170504960097318 ) ) ;
#7322=VECTOR ( 'NONE', #10204, 999.9999999999998863 ) ;
#7329=EDGE_CURVE ( 'NONE', #15055, #4567, #19521, .T. ) ;
#7331=DIRECTION ( 'NONE',  ( -0.5000000000000049960, 0.8660254037844357100, -0.000000000000000000 ) ) ;
#7337=CONICAL_SURFACE ( 'NONE', #20552, 13.07248899748297433, 0.6693469023067423196 ) ;
#7344=ORIENTED_EDGE ( 'NONE', *, *, #7441, .F. ) ;
#7354=DIRECTION ( 'NONE',  ( -0.7743856023693681534, 0.000000000000000000, -0.6327139470906508745 ) ) ;
#7355=CARTESIAN_POINT ( 'NONE',  ( 207.0013954503587286, 3.383002205901548098, -25.76107385416581508 ) ) ;
#7362=DIRECTION ( 'NONE',  ( 0.5000000000000054401, -0.8660254037844354880, 0.000000000000000000 ) ) ;
#7364=ORIENTED_EDGE ( 'NONE', *, *, #7329, .T. ) ;
#7365=ORIENTED_EDGE ( 'NONE', *, *, #3990, .T. ) ;
#7366=FACE_OUTER_BOUND ( 'NONE', #5045, .T. ) ;
#7372=CARTESIAN_POINT ( 'NONE',  ( 208.0983737146324870, 5.661548828456886895, -14.00000000000005507 ) ) ;
#7373=ORIENTED_EDGE ( 'NONE', *, *, #17861, .T. ) ;
#7374=CARTESIAN_POINT ( 'NONE',  ( 208.0983737146324870, 5.661548828456886895, -14.00000000000005507 ) ) ;
#7375=CIRCLE ( 'NONE', #10418, 2.961423854602166283 ) ;
#7381=EDGE_CURVE ( 'NONE', #8117, #425, #9694, .T. ) ;
#7387=ORIENTED_EDGE ( 'NONE', *, *, #2171, .F. ) ;
#7394=ORIENTED_EDGE ( 'NONE', *, *, #12518, .T. ) ;
#7398=CARTESIAN_POINT ( 'NONE',  ( 203.7831613941889088, 8.947961373646505123, -25.80036831778739881 ) ) ;
#7399=FACE_OUTER_BOUND ( 'NONE', #4200, .T. ) ;
#7400=CARTESIAN_POINT ( 'NONE',  ( 212.9607779367323417, 18.37065867240589156, -8.669480444820855780 ) ) ;
#7403=DIRECTION ( 'NONE',  ( 0.5171545105027484102, 0.2985792958513954209, -0.8021231927550452889 ) ) ;
#7404=CARTESIAN_POINT ( 'NONE',  ( 209.4102522745655506, 3.389308509292514149, -14.00000000000005507 ) ) ;
#7415=ORIENTED_EDGE ( 'NONE', *, *, #14357, .F. ) ;
#7417=PLANE ( 'NONE',  #18971 ) ;
#7418=CARTESIAN_POINT ( 'NONE',  ( 196.8817620068315080, 4.786426675387034813, -7.327415643059290495 ) ) ;
#7420=EDGE_CURVE ( 'NONE', #14942, #14915, #7004, .T. ) ;
#7422=DIRECTION ( 'NONE',  ( -0.1997192025788214198, -0.1153079353712215815, -0.9730448705798235842 ) ) ;
#7428=EDGE_CURVE ( 'NONE', #12664, #1475, #4659, .T. ) ;
#7430=CARTESIAN_POINT ( 'NONE',  ( 209.9266392777186923, 12.49489998346296460, -14.00000000000005507 ) ) ;
#7432=FACE_OUTER_BOUND ( 'NONE', #2723, .T. ) ;
#7433=CARTESIAN_POINT ( 'NONE',  ( 210.7598317367304332, 3.058394523489540884, -14.00000000000005507 ) ) ;
#7434=CARTESIAN_POINT ( 'NONE',  ( 205.6843207647078771, 2.880188005405192264, -2.388950188371906869 ) ) ;
#7441=EDGE_CURVE ( 'NONE', #8757, #10193, #14854, .T. ) ;
#7445=CIRCLE ( 'NONE', #10482, 12.47473710546057823 ) ;
#7449=ORIENTED_EDGE ( 'NONE', *, *, #4244, .T. ) ;
#7455=CARTESIAN_POINT ( 'NONE',  ( 195.7326308045045380, 3.945958789216395424, -9.783550055872323625 ) ) ;
#7456=EDGE_CURVE ( 'NONE', #3353, #2978, #6346, .T. ) ;
#7457=AXIS2_PLACEMENT_3D ( 'NONE', #9750, #11359, #543 ) ;
#7459=AXIS2_PLACEMENT_3D ( 'NONE', #6108, #19066, #16001 ) ;
#7462=ORIENTED_EDGE ( 'NONE', *, *, #18872, .F. ) ;
#7463=DIRECTION ( 'NONE',  ( 0.6946590618905412740, 0.4010615963775223669, -0.5971585917027958379 ) ) ;
#7471=VERTEX_POINT ( 'NONE', #5165 ) ;
#7475=ORIENTED_EDGE ( 'NONE', *, *, #5888, .F. ) ;
#7477=CARTESIAN_POINT ( 'NONE',  ( 217.9607779367323985, 9.710404634561534465, -8.669480444820854004 ) ) ;
#7484=DIRECTION ( 'NONE',  ( 0.8660254037844355990, 0.5000000000000054401, 0.000000000000000000 ) ) ;
#7491=DIRECTION ( 'NONE',  ( 0.5000000000000054401, -0.8660254037844354880, 0.000000000000000000 ) ) ;
#7494=CARTESIAN_POINT ( 'NONE',  ( 214.9776847560361830, 7.988114983668789471, -4.409371045253012156 ) ) ;
#7495=VECTOR ( 'NONE', #2868, 999.9999999999998863 ) ;
#7497=ORIENTED_EDGE ( 'NONE', *, *, #4342, .F. ) ;
#7499=CARTESIAN_POINT ( 'NONE',  ( 204.9818247258934321, 9.640009970873835599, -14.00000000000005507 ) ) ;
#7504=LINE ( 'NONE', #2646, #5415 ) ;
#7508=ORIENTED_EDGE ( 'NONE', *, *, #5523, .T. ) ;
#7511=DIRECTION ( 'NONE',  ( -0.5000000000000051070, 0.8660254037844359321, -0.000000000000000000 ) ) ;
#7514=B_SPLINE_CURVE_WITH_KNOTS ( 'NONE', 3,
 ( #1453, #11092, #11198, #14301 ),
 .UNSPECIFIED., .F., .F.,
 ( 4, 4 ),
 ( 3.280426939088333109E-07, 0.0006729788347424356214 ),
 .UNSPECIFIED. ) ;
#7518=DIRECTION ( 'NONE',  ( -0.5000000000000054401, 0.8660254037844354880, -0.000000000000000000 ) ) ;
#7524=AXIS2_PLACEMENT_3D ( 'NONE', #16993, #13060, #14561 ) ;
#7526=ADVANCED_FACE ( 'NONE', ( #110 ), #2003, .F. ) ;
#7527=CONICAL_SURFACE ( 'NONE', #18375, 38.65920715899539317, 0.03863996524032856789 ) ;
#7529=VERTEX_POINT ( 'NONE', #3487 ) ;
#7535=LINE ( 'NONE', #14027, #2849 ) ;
#7536=EDGE_LOOP ( 'NONE', ( #1452, #8223, #9526, #10707, #5451, #12166 ) ) ;
#7537=EDGE_CURVE ( 'NONE', #1461, #16239, #13548, .T. ) ;
#7541=DIRECTION ( 'NONE',  ( -0.5000000000000049960, 0.8660254037844357100, -0.000000000000000000 ) ) ;
#7547=CARTESIAN_POINT ( 'NONE',  ( 212.8532021079397225, 7.019143578708644249, -2.867675856073738760 ) ) ;
#7548=CARTESIAN_POINT ( 'NONE',  ( 209.3577481411911663, 3.480248335904243095, -14.00000000000005507 ) ) ;
#7549=ADVANCED_BREP_SHAPE_REPRESENTATION ( '', ( #17843, #18233 ), #3328 ) ;
#7557=DIRECTION ( 'NONE',  ( 0.5000000000000057732, -0.8660254037844352659, -1.942890293094023699E-16 ) ) ;
#7562=ADVANCED_FACE ( 'NONE', ( #14955 ), #18218, .T. ) ;
#7565=AXIS2_PLACEMENT_3D ( 'NONE', #13891, #18658, #15397 ) ;
#7567=VECTOR ( 'NONE', #8480, 1000.000000000000114 ) ;
#7571=DIRECTION ( 'NONE',  ( 0.5000000000000051070, -0.8660254037844359321, 0.000000000000000000 ) ) ;
#7573=DIRECTION ( 'NONE',  ( 0.5000000000000049960, -0.8660254037844358210, 0.000000000000000000 ) ) ;
#7576=ORIENTED_EDGE ( 'NONE', *, *, #14862, .T. ) ;
#7584=FACE_OUTER_BOUND ( 'NONE', #4534, .T. ) ;
#7585=VECTOR ( 'NONE', #14221, 1000.000000000000227 ) ;
#7586=EDGE_CURVE ( 'NONE', #8365, #9396, #12173, .T. ) ;
#7588=CARTESIAN_POINT ( 'NONE',  ( 200.8946500511725333, -0.1427288941911568354, -6.310089745291766583 ) ) ;
#7589=VERTEX_POINT ( 'NONE', #10351 ) ;
#7592=B_SPLINE_CURVE_WITH_KNOTS ( 'NONE', 3,
 ( #15080, #15183, #5178, #19597 ),
 .UNSPECIFIED., .F., .F.,
 ( 4, 4 ),
 ( 5.109387134629360757E-05, 0.0009050796093292725166 ),
 .UNSPECIFIED. ) ;
#7601=ORIENTED_EDGE ( 'NONE', *, *, #6263, .F. ) ;
#7606=EDGE_CURVE ( 'NONE', #15581, #8339, #19905, .T. ) ;
#7608=ORIENTED_EDGE ( 'NONE', *, *, #17135, .T. ) ;
#7609=ORIENTED_EDGE ( 'NONE', *, *, #13714, .F. ) ;
#7610=ORIENTED_EDGE ( 'NONE', *, *, #19445, .F. ) ;
#7616=ORIENTED_EDGE ( 'NONE', *, *, #13154, .F. ) ;
#7619=DIRECTION ( 'NONE',  ( -0.8296432542242749841, -0.4789947561577487245, 0.2868032327110942581 ) ) ;
#7623=CARTESIAN_POINT ( 'NONE',  ( 211.9531851547456540, 13.48791688690614521, -4.253719131806259490 ) ) ;
#7628=CARTESIAN_POINT ( 'NONE',  ( 202.2239086947344617, 1.139925180369061097, -4.138477629886050835 ) ) ;
#7633=VERTEX_POINT ( 'NONE', #7184 ) ;
#7634=AXIS2_PLACEMENT_3D ( 'NONE', #3503, #10053, #8586 ) ;
#7642=ORIENTED_EDGE ( 'NONE', *, *, #2394, .T. ) ;
#7644=DIRECTION ( 'NONE',  ( -0.5000000000000049960, 0.8660254037844358210, -0.000000000000000000 ) ) ;
#7647=AXIS2_PLACEMENT_3D ( 'NONE', #4667, #12841, #11137 ) ;
#7651=DIRECTION ( 'NONE',  ( 0.5000000000000051070, -0.8660254037844359321, 0.000000000000000000 ) ) ;
#7660=EDGE_LOOP ( 'NONE', ( #20749, #18221, #10464, #20438 ) ) ;
#7662=CIRCLE ( 'NONE', #19502, 1.000000000000000888 ) ;
#7669=CARTESIAN_POINT ( 'NONE',  ( 218.7874248973968179, 10.18766947982593862, -16.70797078425240301 ) ) ;
#7674=VECTOR ( 'NONE', #13258, 1000.000000000000227 ) ;
#7675=CARTESIAN_POINT ( 'NONE',  ( 219.5005434568853673, 10.59938867211075042, -9.448537646917804622 ) ) ;
#7679=CARTESIAN_POINT ( 'NONE',  ( 214.9776847560361830, 7.988114983668789471, -4.409371045253012156 ) ) ;
#7686=CARTESIAN_POINT ( 'NONE',  ( 200.4130575059754733, 6.471181724797008705, -24.79563718815128226 ) ) ;
#7691=ORIENTED_EDGE ( 'NONE', *, *, #9457, .T. ) ;
#7693=CIRCLE ( 'NONE', #1284, 12.47473710546057823 ) ;
#7696=CARTESIAN_POINT ( 'NONE',  ( 210.9359965013291003, 12.90064274403945532, -3.481206571632993629 ) ) ;
#7702=VECTOR ( 'NONE', #3420, 1000.000000000000114 ) ;
#7703=VERTEX_POINT ( 'NONE', #16939 ) ;
#7706=CARTESIAN_POINT ( 'NONE',  ( 195.3764439868359943, 3.740314234153661488, -16.84511136304289991 ) ) ;
#7707=PLANE ( 'NONE',  #19655 ) ;
#7718=EDGE_CURVE ( 'NONE', #17213, #1051, #8288, .T. ) ;
#7719=ADVANCED_FACE ( 'NONE', ( #10570 ), #10127, .T. ) ;
#7720=EDGE_LOOP ( 'NONE', ( #18727, #12927, #2981, #10137 ) ) ;
#7722=CARTESIAN_POINT ( 'NONE',  ( 193.8010743977839354, 17.92347240697177568, -24.79563718815128226 ) ) ;
#7725=CARTESIAN_POINT ( 'NONE',  ( 211.7854512130869580, 13.56808555472074751, -4.379064819896290928 ) ) ;
#7733=ORIENTED_EDGE ( 'NONE', *, *, #2828, .F. ) ;
#7736=B_SPLINE_CURVE_WITH_KNOTS ( 'NONE', 3,
 ( #10922, #7628, #16973, #20352 ),
 .UNSPECIFIED., .F., .F.,
 ( 4, 4 ),
 ( 4.203583919701888644E-07, 0.0008544060963714298707 ),
 .UNSPECIFIED. ) ;
#7747=DIRECTION ( 'NONE',  ( -0.5000000000000049960, 0.8660254037844357100, -0.000000000000000000 ) ) ;
#7753=CARTESIAN_POINT ( 'NONE',  ( 206.2654030616020293, 10.38108426852119415, -14.49413924534530551 ) ) ;
#7757=CARTESIAN_POINT ( 'NONE',  ( 212.1242269781990899, 6.340670367513290273, -26.58724934764018855 ) ) ;
#7763=VERTEX_POINT ( 'NONE', #7494 ) ;
#7769=CARTESIAN_POINT ( 'NONE',  ( 201.0525450381139194, 0.7212519096665224172, -23.06309126349794525 ) ) ;
#7770=CARTESIAN_POINT ( 'NONE',  ( 208.4761278624580711, 5.007259451653140125, -14.00000000000005507 ) ) ;
#7776=ORIENTED_EDGE ( 'NONE', *, *, #18872, .T. ) ;
#7777=CARTESIAN_POINT ( 'NONE',  ( 212.9190227734775078, 14.22255340025794190, -23.49337750257581803 ) ) ;
#7778=LINE ( 'NONE', #3222, #16174 ) ;
#7779=VECTOR ( 'NONE', #16686, 1000.000000000000114 ) ;
#7782=ORIENTED_EDGE ( 'NONE', *, *, #11895, .T. ) ;
#7784=EDGE_CURVE ( 'NONE', #15951, #4803, #11099, .T. ) ;
#7785=ORIENTED_EDGE ( 'NONE', *, *, #14511, .T. ) ;
#7787=FACE_OUTER_BOUND ( 'NONE', #2904, .T. ) ;
#7791=DIRECTION ( 'NONE',  ( 0.5000000000000054401, -0.8660254037844354880, 0.000000000000000000 ) ) ;
#7796=EDGE_LOOP ( 'NONE', ( #8087, #4179, #4809, #5274 ) ) ;
#7799=DIRECTION ( 'NONE',  ( 0.8645602258681718277, 0.4991540791356397500, 0.05814482891046558743 ) ) ;
#7806=ORIENTED_EDGE ( 'NONE', *, *, #6755, .T. ) ;
#7807=VERTEX_POINT ( 'NONE', #5997 ) ;
#7811=CARTESIAN_POINT ( 'NONE',  ( 209.9156946368443357, 16.61257900951069288, -4.494676796018852727 ) ) ;
#7813=EDGE_LOOP ( 'NONE', ( #9275, #14784, #14965, #3182, #7415, #13670, #2218, #8373, #178, #7616, #2742, #17036, #11607, #10336, #1308, #10303, #13769, #2597, #8191, #6491, #18080, #3724, #9862, #14963, #2265, #12944, #10585, #20747, #9450, #8569, #12945, #15777, #11740, #3647, #3419, #9736, #20900, #6595, #6899, #2428, #17660, #18258, #12818, #19848, #17787, #2128, #13564, #14069, #9562, #1838, #7462, #13107, #19567, #5098, #7938, #4905, #4541, #18119, #17610, #13269, #19345, #20125, #7126, #16949, #17839, #6475, #6794, #10669, #14013, #6950, #4576, #16704, #3799, #20430, #18951, #12817, #12201, #5548, #15691, #1822, #7962, #14725, #3562, #7111, #5908, #14539, #1736, #712, #17502, #6203, #9982, #14017, #7871, #15184, #20332, #13654, #1133, #1004, #9264, #5540, #1059, #19976, #10379, #717, #8315, #11015, #17287, #6061 ) ) ;
#7816=CARTESIAN_POINT ( 'NONE',  ( 216.7268875047958829, 8.998017661532479394, -6.310089745291985963 ) ) ;
#7819=CARTESIAN_POINT ( 'NONE',  ( 202.6305150283801026, 8.282480684066333865, -25.48492467622465441 ) ) ;
#7824=EDGE_CURVE ( 'NONE', #2011, #12209, #9125, .T. ) ;
#7828=EDGE_CURVE ( 'NONE', #16338, #600, #2738, .T. ) ;
#7834=DIRECTION ( 'NONE',  ( 0.1503837331804443733, 0.08682408883347179918, 0.9848077530122060219 ) ) ;
#7835=DIRECTION ( 'NONE',  ( 0.5000000000000054401, -0.8660254037844354880, 0.000000000000000000 ) ) ;
#7836=EDGE_CURVE ( 'NONE', #15363, #694, #19059, .T. ) ;
#7837=ORIENTED_EDGE ( 'NONE', *, *, #2261, .T. ) ;
#7846=AXIS2_PLACEMENT_3D ( 'NONE', #4493, #12451, #14155 ) ;
#7853=ADVANCED_FACE ( 'NONE', ( #1355 ), #17152, .F. ) ;
#7856=CARTESIAN_POINT ( 'NONE',  ( 208.5367637565365726, 11.69245497716839566, -11.22024895763578556 ) ) ;
#7857=ORIENTED_EDGE ( 'NONE', *, *, #14172, .T. ) ;
#7858=DIRECTION ( 'NONE',  ( 0.5000000000000054401, -0.8660254037844354880, 0.000000000000000000 ) ) ;
#7859=CARTESIAN_POINT ( 'NONE',  ( 210.7763206480203166, 12.98546375133203767, -24.38552490958320718 ) ) ;
#7860=EDGE_CURVE ( 'NONE', #3143, #20843, #12150, .T. ) ;
#7862=DIRECTION ( 'NONE',  ( -0.8660254037844355990, -0.5000000000000054401, 8.343535232742331521E-16 ) ) ;
#7864=FACE_OUTER_BOUND ( 'NONE', #4262, .T. ) ;
#7865=ORIENTED_EDGE ( 'NONE', *, *, #589, .F. ) ;
#7871=ORIENTED_EDGE ( 'NONE', *, *, #8069, .F. ) ;
#7872=ORIENTED_EDGE ( 'NONE', *, *, #15618, .T. ) ;
#7875=CARTESIAN_POINT ( 'NONE',  ( 215.5731683782092034, 15.75492507961826227, -16.70797078425240301 ) ) ;
#7876=ORIENTED_EDGE ( 'NONE', *, *, #8104, .F. ) ;
#7879=CARTESIAN_POINT ( 'NONE',  ( 198.7478178127443016, -1.382203064952688409, -11.23040475586387821 ) ) ;
#7882=CARTESIAN_POINT ( 'NONE',  ( 210.6201421056092897, 5.472286561439484665, -25.76107385416583639 ) ) ;
#7884=CIRCLE ( 'NONE', #457, 11.98469917212512215 ) ;
#7889=ORIENTED_EDGE ( 'NONE', *, *, #15805, .F. ) ;
#7892=CARTESIAN_POINT ( 'NONE',  ( 200.8776667170992027, -0.1525342266901607846, -21.66653917424381603 ) ) ;
#7893=PLANE ( 'NONE',  #4109 ) ;
#7894=CARTESIAN_POINT ( 'NONE',  ( 207.4990653133776277, 25.83201114944695220, -5.993340328401894901 ) ) ;
#7896=CARTESIAN_POINT ( 'NONE',  ( 200.6602785227575225, -0.02044413540491671344, -6.204501730076046329 ) ) ;
#7899=VERTEX_POINT ( 'NONE', #20939 ) ;
#7900=CARTESIAN_POINT ( 'NONE',  ( 197.5856452450873917, 5.015797175299181454, -21.91826003371427944 ) ) ;
#7907=EDGE_LOOP ( 'NONE', ( #2391, #9683, #1315, #18520, #17641, #13929 ) ) ;
#7911=DIRECTION ( 'NONE',  ( 0.5000000000000052180, -0.8660254037844355990, -1.665334536937734318E-16 ) ) ;
#7915=EDGE_LOOP ( 'NONE', ( #834, #17418, #937, #20601 ) ) ;
#7917=DIRECTION ( 'NONE',  ( 0.5330816498126389469, -0.8460638005688666530, 0.000000000000000000 ) ) ;
#7918=DIRECTION ( 'NONE',  ( 0.9736467517689000317, -0.2280614013152375275, 0.000000000000000000 ) ) ;
#7921=EDGE_LOOP ( 'NONE', ( #4815, #10742, #9481, #6390 ) ) ;
#7927=CARTESIAN_POINT ( 'NONE',  ( 199.6438684810882762, -0.8648679703767148119, -19.29168348739290906 ) ) ;
#7930=ORIENTED_EDGE ( 'NONE', *, *, #20095, .T. ) ;
#7932=CARTESIAN_POINT ( 'NONE',  ( 203.6701878702990598, 1.459728612827534855, -3.762296834228767928 ) ) ;
#7933=CARTESIAN_POINT ( 'NONE',  ( 195.6699422177752581, 3.732742836357164862, -18.25196083293855054 ) ) ;
#7938=ORIENTED_EDGE ( 'NONE', *, *, #20264, .F. ) ;
#7942=FACE_OUTER_BOUND ( 'NONE', #13543, .T. ) ;
#7945=EDGE_LOOP ( 'NONE', ( #6951, #637, #19787, #11696 ) ) ;
#7948=ADVANCED_FACE ( 'NONE', ( #1976 ), #1349, .F. ) ;
#7951=CARTESIAN_POINT ( 'NONE',  ( 206.6806582365933878, 10.62083195558484405, -12.63579004172483877 ) ) ;
#7954=CARTESIAN_POINT ( 'NONE',  ( 195.0230325291159090, 3.359249353468287680, -14.01558723443171850 ) ) ;
#7957=ADVANCED_FACE ( 'NONE', ( #11513 ), #11310, .F. ) ;
#7959=FACE_OUTER_BOUND ( 'NONE', #12809, .T. ) ;
#7961=AXIS2_PLACEMENT_3D ( 'NONE', #6986, #16544, #5080 ) ;
#7962=ORIENTED_EDGE ( 'NONE', *, *, #3134, .F. ) ;
#7963=AXIS2_PLACEMENT_3D ( 'NONE', #18239, #15300, #19924 ) ;
#7964=DIRECTION ( 'NONE',  ( 0.5000000000000051070, -0.8660254037844359321, 0.000000000000000000 ) ) ;
#7965=EDGE_CURVE ( 'NONE', #3973, #12454, #19667, .T. ) ;
#7973=VERTEX_POINT ( 'NONE', #83 ) ;
#7975=DIRECTION ( 'NONE',  ( 0.8660254037844352659, 0.5000000000000056621, 0.000000000000000000 ) ) ;
#7978=VECTOR ( 'NONE', #15490, 1000.000000000000114 ) ;
#7980=CIRCLE ( 'NONE', #6293, 12.47473710546057823 ) ;
#7984=DIRECTION ( 'NONE',  ( -0.5000000000000051070, 0.8660254037844359321, -0.000000000000000000 ) ) ;
#7986=ORIENTED_EDGE ( 'NONE', *, *, #1246, .T. ) ;
#7991=DIRECTION ( 'NONE',  ( -0.5000000000000051070, 0.8660254037844359321, -0.000000000000000000 ) ) ;
#7992=EDGE_CURVE ( 'NONE', #19959, #844, #14512, .T. ) ;
#7994=CARTESIAN_POINT ( 'NONE',  ( 208.8107687779841228, 4.427644383670616079, -14.00000000000005507 ) ) ;
#8013=ORIENTED_EDGE ( 'NONE', *, *, #11585, .F. ) ;
#8017=CARTESIAN_POINT ( 'NONE',  ( 216.0745536026543334, 15.96406172101338683, -13.99136402100517174 ) ) ;
#8018=DIRECTION ( 'NONE',  ( -1.060575238724903217E-16, -6.123233995736827666E-17, 1.000000000000000000 ) ) ;
#8022=PLANE ( 'NONE',  #20611 ) ;
#8025=CARTESIAN_POINT ( 'NONE',  ( 211.0559258593130210, 13.14689389533870312, -25.15632882797110526 ) ) ;
#8029=VECTOR ( 'NONE', #18510, 1000.000000000000227 ) ;
#8031=CARTESIAN_POINT ( 'NONE',  ( 198.6293134455681013, -1.450621593242038099, -12.64773574313024440 ) ) ;
#8036=VERTEX_POINT ( 'NONE', #4838 ) ;
#8037=CARTESIAN_POINT ( 'NONE',  ( 199.0943133668587564, -1.182153763511707867, -18.09983247376283089 ) ) ;
#8041=ORIENTED_EDGE ( 'NONE', *, *, #1901, .F. ) ;
#8047=CARTESIAN_POINT ( 'NONE',  ( 208.8107687779841228, 4.427644383670616079, -14.00000000000005507 ) ) ;
#8050=EDGE_CURVE ( 'NONE', #13300, #15277, #17889, .T. ) ;
#8053=LINE ( 'NONE', #11263, #9884 ) ;
#8056=CARTESIAN_POINT ( 'NONE',  ( 199.2542003381766449, 10.45716240621115745, -1.942038651984764330 ) ) ;
#8057=VECTOR ( 'NONE', #7644, 1000.000000000000227 ) ;
#8058=ORIENTED_EDGE ( 'NONE', *, *, #8050, .F. ) ;
#8059=DIRECTION ( 'NONE',  ( -0.8660254037844354880, -0.5000000000000055511, 0.000000000000000000 ) ) ;
#8061=EDGE_CURVE ( 'NONE', #6334, #791, #11207, .T. ) ;
#8062=FACE_OUTER_BOUND ( 'NONE', #16745, .T. ) ;
#8064=ORIENTED_EDGE ( 'NONE', *, *, #14113, .F. ) ;
#8066=DIRECTION ( 'NONE',  ( -0.000000000000000000, -0.000000000000000000, 1.000000000000000000 ) ) ;
#8067=UNCERTAINTY_MEASURE_WITH_UNIT (LENGTH_MEASURE( 1.000000000000000082E-05 ), #11108, 'distance_accuracy_value', 'NONE');
#8069=EDGE_CURVE ( 'NONE', #9213, #19498, #10825, .T. ) ;
#8070=CARTESIAN_POINT ( 'NONE',  ( 205.8264633344831225, 9.596613037118636669, -14.00000000000005507 ) ) ;
#8077=DIRECTION ( 'NONE',  ( 0.8660254037844357100, 0.5000000000000049960, -3.055037149610301786E-16 ) ) ;
#8082=CARTESIAN_POINT ( 'NONE',  ( 203.8492256719332829, 8.809093698002534722, -2.035916199211759370 ) ) ;
#8084=VECTOR ( 'NONE', #11305, 999.9999999999998863 ) ;
#8086=CARTESIAN_POINT ( 'NONE',  ( 202.0125913935839037, 12.04972022458082037, -25.65046807331631129 ) ) ;
#8087=ORIENTED_EDGE ( 'NONE', *, *, #13951, .F. ) ;
#8092=DIRECTION ( 'NONE',  ( 0.5000000000000054401, -0.8660254037844354880, 0.000000000000000000 ) ) ;
#8097=CARTESIAN_POINT ( 'NONE',  ( 201.5598379337182848, 7.133275713455735634, -25.46066938576250394 ) ) ;
#8100=ORIENTED_EDGE ( 'NONE', *, *, #5009, .F. ) ;
#8104=EDGE_CURVE ( 'NONE', #4228, #3143, #2030, .T. ) ;
#8109=ORIENTED_EDGE ( 'NONE', *, *, #19233, .F. ) ;
#8112=DIRECTION ( 'NONE',  ( -0.5000000000000051070, 0.8660254037844359321, -0.000000000000000000 ) ) ;
#8117=VERTEX_POINT ( 'NONE', #10220 ) ;
#8118=VERTEX_POINT ( 'NONE', #13741 ) ;
#8119=DIRECTION ( 'NONE',  ( 0.5000000000000051070, -0.8660254037844359321, 0.000000000000000000 ) ) ;
#8121=FACE_OUTER_BOUND ( 'NONE', #19919, .T. ) ;
#8122=VECTOR ( 'NONE', #5950, 999.9999999999998863 ) ;
#8129=AXIS2_PLACEMENT_3D ( 'NONE', #5904, #15894, #15698 ) ;
#8136=DIRECTION ( 'NONE',  ( -0.5000000000000049960, 0.8660254037844358210, -0.000000000000000000 ) ) ;
#8137=AXIS2_PLACEMENT_3D ( 'NONE', #19369, #16501, #1879 ) ;
#8144=CARTESIAN_POINT ( 'NONE',  ( 197.5418782473972499, 4.813505606965178707, -5.993340328401664863 ) ) ;
#8145=VECTOR ( 'NONE', #16598, 1000.000000000000114 ) ;
#8150=AXIS2_PLACEMENT_3D ( 'NONE', #920, #4410, #5777 ) ;
#8151=VECTOR ( 'NONE', #19140, 1000.000000000000114 ) ;
#8158=DIRECTION ( 'NONE',  ( -0.4330127018922214077, -0.2500000000000045519, -0.8660254037844363761 ) ) ;
#8159=CARTESIAN_POINT ( 'NONE',  ( 199.4425753138606296, -0.2082645440182918917, -20.84195174293567376 ) ) ;
#8166=AXIS2_PLACEMENT_3D ( 'NONE', #8056, #5089, #19413 ) ;
#8167=EDGE_LOOP ( 'NONE', ( #3633, #19169, #7497, #18001 ) ) ;
#8172=ORIENTED_EDGE ( 'NONE', *, *, #7208, .T. ) ;
#8176=VERTEX_POINT ( 'NONE', #2510 ) ;
#8182=VERTEX_POINT ( 'NONE', #15453 ) ;
#8183=LINE ( 'NONE', #20904, #7702 ) ;
#8185=AXIS2_PLACEMENT_3D ( 'NONE', #5007, #17652, #15963 ) ;
#8190=DIRECTION ( 'NONE',  ( 0.5000000000000054401, -0.8660254037844354880, 0.000000000000000000 ) ) ;
#8191=ORIENTED_EDGE ( 'NONE', *, *, #20007, .F. ) ;
#8195=B_SPLINE_CURVE_WITH_KNOTS ( 'NONE', 3,
 ( #17190, #19935, #7418, #12211 ),
 .UNSPECIFIED., .F., .F.,
 ( 4, 4 ),
 ( 4.589663078223623554E-07, 0.0006731097583619476436 ),
 .UNSPECIFIED. ) ;
#8197=ORIENTED_EDGE ( 'NONE', *, *, #7183, .F. ) ;
#8201=CARTESIAN_POINT ( 'NONE',  ( 188.4110409874304253, 14.81153516656304880, -14.00000000000005507 ) ) ;
#8202=CARTESIAN_POINT ( 'NONE',  ( 218.9922241104002012, 10.30591036058324583, -12.64773574313060678 ) ) ;
#8206=EDGE_CURVE ( 'NONE', #19279, #4064, #1439, .T. ) ;
#8209=CIRCLE ( 'NONE', #16028, 0.004059536337672174817 ) ;
#8210=ORIENTED_EDGE ( 'NONE', *, *, #20794, .T. ) ;
#8215=CARTESIAN_POINT ( 'NONE',  ( 213.3673372177917997, 7.058380398974537506, -1.942038651984889785 ) ) ;
#8223=ORIENTED_EDGE ( 'NONE', *, *, #11804, .F. ) ;
#8227=CARTESIAN_POINT ( 'NONE',  ( 209.8577037357181894, 2.614299844655262106, -14.00000000000005507 ) ) ;
#8230=ORIENTED_EDGE ( 'NONE', *, *, #1187, .F. ) ;
#8232=LINE ( 'NONE', #11328, #8705 ) ;
#8236=FACE_OUTER_BOUND ( 'NONE', #6463, .T. ) ;
#8238=CARTESIAN_POINT ( 'NONE',  ( 199.3200586684138784, -0.7942204290835060965, -8.555339712719925771 ) ) ;
#8239=VECTOR ( 'NONE', #18234, 1000.000000000000227 ) ;
#8241=AXIS2_PLACEMENT_3D ( 'NONE', #859, #18982, #5709 ) ;
#8244=CARTESIAN_POINT ( 'NONE',  ( 198.0727098700125168, 9.775028566371592120, -25.36561010639676184 ) ) ;
#8248=ORIENTED_EDGE ( 'NONE', *, *, #8809, .T. ) ;
#8249=CARTESIAN_POINT ( 'NONE',  ( 218.9522255890561553, 10.79802344239516998, -11.16899820387762432 ) ) ;
#8251=EDGE_CURVE ( 'NONE', #13321, #5971, #15980, .T. ) ;
#8257=DIRECTION ( 'NONE',  ( 0.5000000000000053291, -0.8660254037844355990, -3.330669073875468142E-16 ) ) ;
#8258=ORIENTED_EDGE ( 'NONE', *, *, #20082, .T. ) ;
#8264=ORIENTED_EDGE ( 'NONE', *, *, #12215, .F. ) ;
#8269=DIRECTION ( 'NONE',  ( -0.5000000000000054401, 0.8660254037844354880, -0.000000000000000000 ) ) ;
#8274=ORIENTED_EDGE ( 'NONE', *, *, #17841, .F. ) ;
#8275=EDGE_LOOP ( 'NONE', ( #3462, #2591, #12397, #1775 ) ) ;
#8278=ORIENTED_EDGE ( 'NONE', *, *, #13805, .T. ) ;
#8281=CARTESIAN_POINT ( 'NONE',  ( 196.7929107858857094, 4.381089041447214782, -20.84195174293567376 ) ) ;
#8288=CIRCLE ( 'NONE', #1695, 12.47473710546057823 ) ;
#8290=EDGE_CURVE ( 'NONE', #7763, #15950, #13162, .T. ) ;
#8292=ORIENTED_EDGE ( 'NONE', *, *, #8050, .T. ) ;
#8296=AXIS2_PLACEMENT_3D ( 'NONE', #18735, #18838, #5986 ) ;
#8299=VERTEX_POINT ( 'NONE', #9468 ) ;
#8301=DIRECTION ( 'NONE',  ( 0.8660254037844355990, 0.5000000000000054401, 0.000000000000000000 ) ) ;
#8302=CARTESIAN_POINT ( 'NONE',  ( 215.4747034159835550, 15.16702704537912183, -19.61257667712965258 ) ) ;
#8303=AXIS2_PLACEMENT_3D ( 'NONE', #9101, #7518, #10917 ) ;
#8306=CARTESIAN_POINT ( 'NONE',  ( 204.5452479762167002, 2.222544024343242608, -2.867675856073625518 ) ) ;
#8308=PLANE ( 'NONE',  #10988 ) ;
#8310=B_SPLINE_CURVE_WITH_KNOTS ( 'NONE', 3,
 ( #4310, #2931, #9372, #14076 ),
 .UNSPECIFIED., .F., .F.,
 ( 4, 4 ),
 ( 2.816680711552148146E-07, 0.0006729324601260043559 ),
 .UNSPECIFIED. ) ;
#8315=ORIENTED_EDGE ( 'NONE', *, *, #15986, .F. ) ;
#8318=CARTESIAN_POINT ( 'NONE',  ( 215.2040058117673595, 19.66578688991103974, -14.05525385477321620 ) ) ;
#8331=ORIENTED_EDGE ( 'NONE', *, *, #1068, .F. ) ;
#8336=VECTOR ( 'NONE', #9248, 1000.000000000000114 ) ;
#8339=VERTEX_POINT ( 'NONE', #14176 ) ;
#8340=CIRCLE ( 'NONE', #20519, 12.47473710546057823 ) ;
#8341=PLANE ( 'NONE',  #4313 ) ;
#8343=ORIENTED_EDGE ( 'NONE', *, *, #16651, .F. ) ;
#8346=DIRECTION ( 'NONE',  ( 0.6299240516454519545, 0.3636868207865264768, -0.6862416378687370422 ) ) ;
#8348=DIRECTION ( 'NONE',  ( -0.5000000000000054401, 0.8660254037844354880, -0.000000000000000000 ) ) ;
#8354=ORIENTED_EDGE ( 'NONE', *, *, #1647, .T. ) ;
#8358=EDGE_CURVE ( 'NONE', #11939, #8182, #9113, .T. ) ;
#8359=VERTEX_POINT ( 'NONE', #16076 ) ;
#8360=LINE ( 'NONE', #212, #3081 ) ;
#8362=DIRECTION ( 'NONE',  ( 0.8660254037844355990, 0.5000000000000054401, 0.000000000000000000 ) ) ;
#8364=LINE ( 'NONE', #2020, #8239 ) ;
#8365=VERTEX_POINT ( 'NONE', #11489 ) ;
#8368=DIRECTION ( 'NONE',  ( -0.5000000000000051070, 0.8660254037844359321, -0.000000000000000000 ) ) ;
#8373=ORIENTED_EDGE ( 'NONE', *, *, #15859, .F. ) ;
#8376=CARTESIAN_POINT ( 'NONE',  ( 215.9002224801550085, 8.520742387026412956, -22.69908973750352743 ) ) ;
#8382=CARTESIAN_POINT ( 'NONE',  ( 211.5875185857062206, 6.803621723274593691, -25.94618751764496878 ) ) ;
#8387=VERTEX_POINT ( 'NONE', #14701 ) ;
#8388=ORIENTED_EDGE ( 'NONE', *, *, #8831, .F. ) ;
#8394=DIRECTION ( 'NONE',  ( 0.5000000000000027756, -0.8660254037844372643, 0.000000000000000000 ) ) ;
#8408=CARTESIAN_POINT ( 'NONE',  ( 192.7739465146478040, 17.33045984715094434, -24.01557619556968248 ) ) ;
#8414=CARTESIAN_POINT ( 'NONE',  ( 214.5005434568852820, 19.25964270995510930, -9.448537646917806399 ) ) ;
#8419=ORIENTED_EDGE ( 'NONE', *, *, #4324, .T. ) ;
#8420=DIRECTION ( 'NONE',  ( 0.8660254037844352659, 0.5000000000000056621, 0.000000000000000000 ) ) ;
#8424=CARTESIAN_POINT ( 'NONE',  ( 211.6495311407713018, 17.61360998178372483, -6.376588578941996488 ) ) ;
#8427=ORIENTED_EDGE ( 'NONE', *, *, #12346, .T. ) ;
#8439=EDGE_CURVE ( 'NONE', #15581, #10176, #7445, .T. ) ;
#8441=EDGE_CURVE ( 'NONE', #11248, #13321, #14389, .T. ) ;
#8443=CIRCLE ( 'NONE', #20295, 11.98469917212512215 ) ;
#8445=VECTOR ( 'NONE', #3044, 999.9999999999998863 ) ;
#8460=ORIENTED_EDGE ( 'NONE', *, *, #1995, .F. ) ;
#8474=ADVANCED_FACE ( 'NONE', ( #17760 ), #9681, .F. ) ;
#8478=ORIENTED_EDGE ( 'NONE', *, *, #14298, .F. ) ;
#8479=DIRECTION ( 'NONE',  ( 0.7499999999999954481, 0.4330127018922224624, -0.5000000000000038858 ) ) ;
#8480=DIRECTION ( 'NONE',  ( 0.5000000000000052180, -0.8660254037844355990, 8.326672684688672821E-17 ) ) ;
#8484=EDGE_CURVE ( 'NONE', #19224, #15281, #10840, .T. ) ;
#8497=VECTOR ( 'NONE', #4850, 1000.000000000000227 ) ;
#8503=DIRECTION ( 'NONE',  ( -0.5943026915289565393, -0.3431208189343671333, 0.7273736415730550631 ) ) ;
#8505=EDGE_LOOP ( 'NONE', ( #2057, #7837, #4515, #16851 ) ) ;
#8511=AXIS2_PLACEMENT_3D ( 'NONE', #9723, #1797, #19285 ) ;
#8517=DIRECTION ( 'NONE',  ( 0.4758887346169486388, 0.2747544890354095548, 0.8354878114129317135 ) ) ;
#8518=CARTESIAN_POINT ( 'NONE',  ( 206.7681187495013262, 14.79532522365839675, -2.669358488461178069 ) ) ;
#8520=ORIENTED_EDGE ( 'NONE', *, *, #16319, .T. ) ;
#8522=DIRECTION ( 'NONE',  ( -0.7235536692358650601, -0.4177439057064745165, -0.5495089780708014571 ) ) ;
#8523=DIRECTION ( 'NONE',  ( -0.5000000000000051070, 0.8660254037844359321, -0.000000000000000000 ) ) ;
#8524=DIRECTION ( 'NONE',  ( -0.8660254037844357100, -0.5000000000000051070, 0.000000000000000000 ) ) ;
#8525=ADVANCED_FACE ( 'NONE', ( #13302 ), #3636, .F. ) ;
#8539=AXIS2_PLACEMENT_3D ( 'NONE', #16887, #5530, #12018 ) ;
#8542=CARTESIAN_POINT ( 'NONE',  ( 208.8107687779841228, 4.427644383670616079, -14.00000000000005507 ) ) ;
#8543=AXIS2_PLACEMENT_3D ( 'NONE', #18414, #4309, #4520 ) ;
#8544=CARTESIAN_POINT ( 'NONE',  ( 197.3251902926419348, 19.95812166752348205, -1.717498466822807490 ) ) ;
#8546=ORIENTED_EDGE ( 'NONE', *, *, #1901, .T. ) ;
#8553=CARTESIAN_POINT ( 'NONE',  ( 217.3836630237427983, 9.377207184193595779, -7.515250618841534447 ) ) ;
#8556=CARTESIAN_POINT ( 'NONE',  ( 215.2334520059837359, 15.55878974066576070, -9.972943347742017295 ) ) ;
#8564=CARTESIAN_POINT ( 'NONE',  ( 206.4411508673863409, 9.951503049707822512, -1.545471579934816875 ) ) ;
#8565=CARTESIAN_POINT ( 'NONE',  ( 208.0983737146324870, 5.661548828456886895, -14.00000000000005507 ) ) ;
#8567=EDGE_CURVE ( 'NONE', #10275, #14507, #370, .T. ) ;
#8569=ORIENTED_EDGE ( 'NONE', *, *, #16067, .F. ) ;
#8571=VECTOR ( 'NONE', #16350, 1000.000000000000227 ) ;
#8573=EDGE_LOOP ( 'NONE', ( #3620, #8058, #20714, #8197, #5686, #12069 ) ) ;
#8576=DIRECTION ( 'NONE',  ( -0.5000000000000054401, 0.8660254037844354880, -0.000000000000000000 ) ) ;
#8580=EDGE_CURVE ( 'NONE', #12707, #19959, #2168, .T. ) ;
#8581=FACE_OUTER_BOUND ( 'NONE', #12239, .T. ) ;
#8583=VECTOR ( 'NONE', #5836, 1000.000000000000000 ) ;
#8586=DIRECTION ( 'NONE',  ( 0.8660254037844355990, 0.5000000000000054401, 8.343535232742331521E-16 ) ) ;
#8589=DIRECTION ( 'NONE',  ( -0.2961981327260172492, -0.1710100716628330242, 0.9396926207859107594 ) ) ;
#8600=EDGE_LOOP ( 'NONE', ( #2424, #3212, #17838, #4076 ) ) ;
#8601=ADVANCED_FACE ( 'NONE', ( #13509 ), #17965, .T. ) ;
#8602=EDGE_LOOP ( 'NONE', ( #18865, #19274, #18155, #9062 ) ) ;
#8603=CARTESIAN_POINT ( 'NONE',  ( 212.8872982515398178, 6.781229772587438198, -24.85758746085098991 ) ) ;
#8604=ORIENTED_EDGE ( 'NONE', *, *, #9485, .T. ) ;
#8607=CARTESIAN_POINT ( 'NONE',  ( 211.7854512130869580, 13.56808555472074751, -4.379064819896290928 ) ) ;
#8613=CIRCLE ( 'NONE', #11331, 4.999999999999968026 ) ;
#8619=CARTESIAN_POINT ( 'NONE',  ( 206.6806582365933593, 10.62083195558481741, -15.36420995827523228 ) ) ;
#8622=EDGE_CURVE ( 'NONE', #16061, #15437, #4050, .T. ) ;
#8624=ORIENTED_EDGE ( 'NONE', *, *, #1780, .T. ) ;
#8629=DIRECTION ( 'NONE',  ( -0.8660254037844355990, -0.5000000000000054401, 0.000000000000000000 ) ) ;
#8642=EDGE_CURVE ( 'NONE', #13417, #18641, #8813, .T. ) ;
#8655=ORIENTED_EDGE ( 'NONE', *, *, #11982, .F. ) ;
#8664=CIRCLE ( 'NONE', #3922, 12.47473710546057823 ) ;
#8667=AXIS2_PLACEMENT_3D ( 'NONE', #2216, #8778, #15275 ) ;
#8668=CARTESIAN_POINT ( 'NONE',  ( 199.2144802262915846, 21.04890371929339921, -14.00000000000005507 ) ) ;
#8669=LINE ( 'NONE', #18425, #11595 ) ;
#8674=ORIENTED_EDGE ( 'NONE', *, *, #6308, .F. ) ;
#8679=ORIENTED_EDGE ( 'NONE', *, *, #20264, .T. ) ;
#8683=VERTEX_POINT ( 'NONE', #17420 ) ;
#8686=ORIENTED_EDGE ( 'NONE', *, *, #14345, .F. ) ;
#8692=CARTESIAN_POINT ( 'NONE',  ( 198.5772061109008746, 5.942301689450959046, -22.62267072728657169 ) ) ;
#8697=CARTESIAN_POINT ( 'NONE',  ( 204.9818247258934321, 9.640009970873835599, -2.187257959407756136 ) ) ;
#8701=ORIENTED_EDGE ( 'NONE', *, *, #6886, .T. ) ;
#8702=CARTESIAN_POINT ( 'NONE',  ( 194.1867014016589508, 7.531440531094472313, -18.06789442459577444 ) ) ;
#8703=CARTESIAN_POINT ( 'NONE',  ( 220.1214136286681651, 10.95784823292136956, -12.41782726985285379 ) ) ;
#8704=ORIENTED_EDGE ( 'NONE', *, *, #20892, .T. ) ;
#8705=VECTOR ( 'NONE', #9719, 1000.000000000000227 ) ;
#8707=EDGE_CURVE ( 'NONE', #15290, #10440, #4276, .T. ) ;
#8712=CARTESIAN_POINT ( 'NONE',  ( 218.8737197432240293, 10.23749183229395676, -11.23040475586419085 ) ) ;
#8713=LINE ( 'NONE', #15211, #562 ) ;
#8716=CARTESIAN_POINT ( 'NONE',  ( 207.9638137018049804, 4.453860881324136045, -26.27710986211782895 ) ) ;
#8718=AXIS2_PLACEMENT_3D ( 'NONE', #6069, #17117, #12565 ) ;
#8719=CARTESIAN_POINT ( 'NONE',  ( 220.2040058117674164, 11.00553285206667908, -14.05525385477321443 ) ) ;
#8720=ORIENTED_EDGE ( 'NONE', *, *, #10687, .T. ) ;
#8724=PRODUCT_DEFINITION ( 'UNKNOWN', '', #5024, #16159 ) ;
#8728=ORIENTED_EDGE ( 'NONE', *, *, #13128, .T. ) ;
#8730=ORIENTED_EDGE ( 'NONE', *, *, #12948, .T. ) ;
#8737=CARTESIAN_POINT ( 'NONE',  ( 212.5692528822464737, 18.14461157680397108, -5.585956497640101048 ) ) ;
#8738=EDGE_CURVE ( 'NONE', #255, #13116, #18996, .T. ) ;
#8749=LINE ( 'NONE', #15355, #5226 ) ;
#8752=ORIENTED_EDGE ( 'NONE', *, *, #12097, .F. ) ;
#8757=VERTEX_POINT ( 'NONE', #9298 ) ;
#8763=PLANE ( 'NONE',  #16142 ) ;
#8767=EDGE_CURVE ( 'NONE', #330, #3291, #13933, .T. ) ;
#8770=VECTOR ( 'NONE', #16210, 1000.000000000000227 ) ;
#8771=CARTESIAN_POINT ( 'NONE',  ( 205.1351227324282718, 9.374490034856508558, -1.709088388254546453 ) ) ;
#8772=EDGE_CURVE ( 'NONE', #9311, #16889, #12658, .T. ) ;
#8773=LINE ( 'NONE', #5263, #17682 ) ;
#8778=DIRECTION ( 'NONE',  ( -0.4330127018922209636, -0.2500000000000048850, -0.8660254037844363761 ) ) ;
#8779=VERTEX_POINT ( 'NONE', #1619 ) ;
#8784=CONICAL_SURFACE ( 'NONE', #6064, 10.85470691220533190, 0.8171114040043576665 ) ;
#8787=CARTESIAN_POINT ( 'NONE',  ( 217.4886294373914382, 9.953015810246625961, -20.75355104716125609 ) ) ;
#8788=ORIENTED_EDGE ( 'NONE', *, *, #6672, .T. ) ;
#8795=DIRECTION ( 'NONE',  ( 0.5000000000000026645, -0.8660254037844370423, 0.000000000000000000 ) ) ;
#8796=B_SPLINE_CURVE_WITH_KNOTS ( 'NONE', 3,
 ( #7859, #1408, #24, #4889 ),
 .UNSPECIFIED., .F., .F.,
 ( 4, 4 ),
 ( 0.0001045099009071127032, 0.0007771606929556430007 ),
 .UNSPECIFIED. ) ;
#8797=DIRECTION ( 'NONE',  ( 0.5000000000000052180, -0.8660254037844355990, 1.665334536937734318E-16 ) ) ;
#8807=VERTEX_POINT ( 'NONE', #9661 ) ;
#8809=EDGE_CURVE ( 'NONE', #20124, #7899, #18250, .T. ) ;
#8813=CIRCLE ( 'NONE', #11529, 4.999999999999968026 ) ;
#8819=CARTESIAN_POINT ( 'NONE',  ( 218.0783914157424590, 10.03590803213535132, -8.555339712720195777 ) ) ;
#8820=VECTOR ( 'NONE', #7918, 1000.000000000000114 ) ;
#8822=DIRECTION ( 'NONE',  ( -0.8296432542242747621, -0.4789947561577490021, 0.2868032327110945912 ) ) ;
#8823=VECTOR ( 'NONE', #1194, 1000.000000000000114 ) ;
#8824=LINE ( 'NONE', #2263, #6151 ) ;
#8828=DIRECTION ( 'NONE',  ( 0.5000000000000054401, -0.8660254037844353769, 2.220446049250312588E-16 ) ) ;
#8831=EDGE_CURVE ( 'NONE', #5298, #8387, #14444, .T. ) ;
#8834=ORIENTED_EDGE ( 'NONE', *, *, #4362, .T. ) ;
#8839=B_SPLINE_CURVE_WITH_KNOTS ( 'NONE', 3,
 ( #11041, #9022, #2468, #2680 ),
 .UNSPECIFIED., .F., .F.,
 ( 4, 4 ),
 ( 3.309335659996554474E-07, 0.0008543166715507651216 ),
 .UNSPECIFIED. ) ;
#8842=VECTOR ( 'NONE', #15645, 1000.000000000000227 ) ;
#8844=ORIENTED_EDGE ( 'NONE', *, *, #17003, .F. ) ;
#8845=VECTOR ( 'NONE', #3335, 1000.000000000000114 ) ;
#8852=ADVANCED_FACE ( 'NONE', ( #7282 ), #12294, .T. ) ;
#8862=EDGE_LOOP ( 'NONE', ( #10658, #11734, #11664, #3961, #7889, #15793 ) ) ;
#8863=ORIENTED_EDGE ( 'NONE', *, *, #8998, .T. ) ;
#8865=CARTESIAN_POINT ( 'NONE',  ( 215.9002224801550085, 8.520742387026412956, -22.69908973750352743 ) ) ;
#8867=DIRECTION ( 'NONE',  ( 0.5000000000000057732, -0.8660254037844352659, 0.000000000000000000 ) ) ;
#8869=ORIENTED_EDGE ( 'NONE', *, *, #10043, .F. ) ;
#8870=AXIS2_PLACEMENT_3D ( 'NONE', #2615, #12365, #15246 ) ;
#8871=ADVANCED_FACE ( 'NONE', ( #4120 ), #16556, .T. ) ;
#8873=CONICAL_SURFACE ( 'NONE', #20047, 13.07248899748297433, 0.6693469023067423196 ) ;
#8874=EDGE_CURVE ( 'NONE', #17245, #6449, #1047, .T. ) ;
#8878=B_SPLINE_CURVE_WITH_KNOTS ( 'NONE', 3,
 ( #8967, #515, #4105, #2311 ),
 .UNSPECIFIED., .F., .F.,
 ( 4, 4 ),
 ( 6.866270341935863685E-05, 0.0009226484414006754300 ),
 .UNSPECIFIED. ) ;
#8889=CARTESIAN_POINT ( 'NONE',  ( 218.9706616721823025, 10.29346128107372316, -19.95367855226146148 ) ) ;
#8894=EDGE_LOOP ( 'NONE', ( #10301, #16922, #14962, #3883, #2327, #20177 ) ) ;
#8895=ORIENTED_EDGE ( 'NONE', *, *, #11184, .T. ) ;
#8897=LINE ( 'NONE', #13786, #13490 ) ;
#8898=CARTESIAN_POINT ( 'NONE',  ( 216.6495311407713871, 8.953355943939367734, -6.376588578941993823 ) ) ;
#8903=CARTESIAN_POINT ( 'NONE',  ( 213.9706616721822456, 18.95371531891807848, -19.95367855226146503 ) ) ;
#8906=ORIENTED_EDGE ( 'NONE', *, *, #6283, .F. ) ;
#8910=ORIENTED_EDGE ( 'NONE', *, *, #16314, .T. ) ;
#8914=CARTESIAN_POINT ( 'NONE',  ( 200.2088966793999987, 0.2341713026616738524, -22.03054070023845767 ) ) ;
#8919=B_SPLINE_CURVE_WITH_KNOTS ( 'NONE', 3,
 ( #10470, #3912, #17170, #11875 ),
 .UNSPECIFIED., .F., .F.,
 ( 4, 4 ),
 ( 9.556227013665790057E-07, 0.0006736064147440891034 ),
 .UNSPECIFIED. ) ;
#8920=CARTESIAN_POINT ( 'NONE',  ( 213.3033847652179134, 18.56846281705820090, -6.724618537539641672 ) ) ;
#8922=CARTESIAN_POINT ( 'NONE',  ( 208.8107687779841228, 4.427644383670616079, -14.00000000000005507 ) ) ;
#8925=DIRECTION ( 'NONE',  ( -0.8660254037844354880, -0.5000000000000055511, 0.000000000000000000 ) ) ;
#8942=PLANE ( 'NONE',  #4626 ) ;
#8945=EDGE_LOOP ( 'NONE', ( #9111, #1235, #13673, #8655, #20742, #11974 ) ) ;
#8948=CARTESIAN_POINT ( 'NONE',  ( 208.3092871949524181, 11.56112132310344798, -15.97949511404853062 ) ) ;
#8949=VERTEX_POINT ( 'NONE', #15888 ) ;
#8960=EDGE_LOOP ( 'NONE', ( #11870, #1570, #6970, #18957 ) ) ;
#8964=CARTESIAN_POINT ( 'NONE',  ( 195.2378745322255611, 8.138335620992030783, -7.515250618841283092 ) ) ;
#8967=CARTESIAN_POINT ( 'NONE',  ( 203.6269058993112253, 1.434739755226664970, -3.662783021451444299 ) ) ;
#8971=CIRCLE ( 'NONE', #7634, 12.47473710546057823 ) ;
#8975=CIRCLE ( 'NONE', #18128, 12.47473710546057823 ) ;
#8976=CARTESIAN_POINT ( 'NONE',  ( 208.2331971963490389, 26.25586238970118558, -7.132002368301439077 ) ) ;
#8979=EDGE_LOOP ( 'NONE', ( #18406, #6520, #16445, #12629, #19704, #3136 ) ) ;
#8980=VERTEX_POINT ( 'NONE', #10892 ) ;
#8984=ORIENTED_EDGE ( 'NONE', *, *, #6295, .T. ) ;
#8988=ADVANCED_FACE ( 'NONE', ( #6107 ), #11104, .F. ) ;
#8993=CIRCLE ( 'NONE', #5260, 12.47473710546057823 ) ;
#8995=DIRECTION ( 'NONE',  ( -0.5000000000000054401, 0.8660254037844354880, -0.000000000000000000 ) ) ;
#8998=EDGE_CURVE ( 'NONE', #3962, #15581, #9429, .T. ) ;
#9001=CARTESIAN_POINT ( 'NONE',  ( 213.9089852488071983, 7.886307274364415143, -3.346771071760026750 ) ) ;
#9006=DIRECTION ( 'NONE',  ( -0.5000000000000054401, 0.8660254037844354880, -0.000000000000000000 ) ) ;
#9013=EDGE_LOOP ( 'NONE', ( #17695, #4146, #12309, #10682, #7785, #5931 ) ) ;
#9017=EDGE_CURVE ( 'NONE', #3518, #16137, #13246, .T. ) ;
#9020=ORIENTED_EDGE ( 'NONE', *, *, #13779, .T. ) ;
#9022=CARTESIAN_POINT ( 'NONE',  ( 211.6378943349726853, 6.575092323907928638, -2.216907231065539552 ) ) ;
#9024=CARTESIAN_POINT ( 'NONE',  ( 201.2821527570645230, 0.5962021362443539196, -5.050953241461257903 ) ) ;
#9026=DIRECTION ( 'NONE',  ( 0.5000000000000054401, -0.8660254037844354880, 0.000000000000000000 ) ) ;
#9028=EDGE_CURVE ( 'NONE', #7589, #1433, #18311, .T. ) ;
#9029=LINE ( 'NONE', #2366, #9548 ) ;
#9031=B_SPLINE_CURVE_WITH_KNOTS ( 'NONE', 3,
 ( #13021, #20946, #12916, #9500 ),
 .UNSPECIFIED., .F., .F.,
 ( 4, 4 ),
 ( 0.0001038643694185014657, 0.0009578501073958695404 ),
 .UNSPECIFIED. ) ;
#9035=VECTOR ( 'NONE', #20853, 1000.000000000000227 ) ;
#9037=DIRECTION ( 'NONE',  ( 0.5000000000000054401, -0.8660254037844354880, 0.000000000000000000 ) ) ;
#9046=LINE ( 'NONE', #20285, #8336 ) ;
#9048=ORIENTED_EDGE ( 'NONE', *, *, #6035, .F. ) ;
#9051=B_SPLINE_CURVE_WITH_KNOTS ( 'NONE', 3,
 ( #7125, #9129, #5419, #13820 ),
 .UNSPECIFIED., .F., .F.,
 ( 4, 4 ),
 ( 6.440264276912068765E-07, 0.0008546297644052478458 ),
 .UNSPECIFIED. ) ;
#9054=CARTESIAN_POINT ( 'NONE',  ( 200.4885253383106374, 7.045802359903295731, -24.25943249057081630 ) ) ;
#9061=CARTESIAN_POINT ( 'NONE',  ( 208.8107687779840944, 4.427644383670621409, -14.00000000000005507 ) ) ;
#9062=ORIENTED_EDGE ( 'NONE', *, *, #744, .F. ) ;
#9065=ADVANCED_FACE ( 'NONE', ( #6848 ), #14625, .F. ) ;
#9072=CYLINDRICAL_SURFACE ( 'NONE', #9452, 4.999999999999973355 ) ;
#9080=VERTEX_POINT ( 'NONE', #13332 ) ;
#9082=DIRECTION ( 'NONE',  ( -0.8660254037844357100, -0.5000000000000051070, 0.000000000000000000 ) ) ;
#9083=DIRECTION ( 'NONE',  ( 0.5000000000000054401, -0.8660254037844354880, 0.000000000000000000 ) ) ;
#9084=EDGE_CURVE ( 'NONE', #9311, #17484, #10444, .T. ) ;
#9085=LINE ( 'NONE', #7811, #9409 ) ;
#9092=ORIENTED_EDGE ( 'NONE', *, *, #16231, .F. ) ;
#9100=FACE_OUTER_BOUND ( 'NONE', #13183, .T. ) ;
#9101=CARTESIAN_POINT ( 'NONE',  ( 205.8264633344831225, 9.596613037118636669, -14.00000000000005507 ) ) ;
#9105=DIRECTION ( 'NONE',  ( -0.8660254037844355990, -0.5000000000000054401, -2.753366626804969431E-14 ) ) ;
#9109=EDGE_CURVE ( 'NONE', #20898, #17666, #15553, .T. ) ;
#9111=ORIENTED_EDGE ( 'NONE', *, *, #5262, .F. ) ;
#9113=B_SPLINE_CURVE_WITH_KNOTS ( 'NONE', 3,
 ( #12784, #8082, #14592, #16376 ),
 .UNSPECIFIED., .F., .F.,
 ( 4, 4 ),
 ( 2.602969390140976553E-05, 0.0006986804859590750897 ),
 .UNSPECIFIED. ) ;
#9114=CARTESIAN_POINT ( 'NONE',  ( 205.0662616026534693, 10.91332106064940888, -14.00000000000005507 ) ) ;
#9116=DIRECTION ( 'NONE',  ( -0.1997192025788092906, -0.1153079353712144900, 0.9730448705798270259 ) ) ;
#9119=LINE ( 'NONE', #20468, #6347 ) ;
#9124=CARTESIAN_POINT ( 'NONE',  ( 218.7787453705537928, 10.18265835266665675, -11.24974199967301836 ) ) ;
#9125=B_SPLINE_CURVE_WITH_KNOTS ( 'NONE', 3,
 ( #15688, #1152, #17573, #19264 ),
 .UNSPECIFIED., .F., .F.,
 ( 4, 4 ),
 ( 9.760775661998381803E-05, 0.0009515934945975094679 ),
 .UNSPECIFIED. ) ;
#9129=CARTESIAN_POINT ( 'NONE',  ( 199.0720388946177195, -0.6798076971790223411, -19.52417598135467713 ) ) ;
#9130=EDGE_LOOP ( 'NONE', ( #3867, #5887, #11048, #13853, #16717, #15358 ) ) ;
#9134=LINE ( 'NONE', #12347, #9535 ) ;
#9138=ORIENTED_EDGE ( 'NONE', *, *, #5262, .T. ) ;
#9150=CARTESIAN_POINT ( 'NONE',  ( 201.4958824572256333, 7.627400263678961068, -2.990331769139143780 ) ) ;
#9151=CONICAL_SURFACE ( 'NONE', #18308, 13.07248899748297433, 0.6693469023067423196 ) ;
#9155=LINE ( 'NONE', #908, #13577 ) ;
#9159=EDGE_LOOP ( 'NONE', ( #6414, #11892, #5145, #60 ) ) ;
#9160=ORIENTED_EDGE ( 'NONE', *, *, #13405, .F. ) ;
#9163=EDGE_CURVE ( 'NONE', #6425, #12475, #16302, .T. ) ;
#9168=CARTESIAN_POINT ( 'NONE',  ( 200.4167038695724443, 7.004336215593725434, -24.38552490958304020 ) ) ;
#9170=AXIS2_PLACEMENT_3D ( 'NONE', #16997, #10191, #15424 ) ;
#9171=CARTESIAN_POINT ( 'NONE',  ( 200.4154830772234561, 6.826621486618904555, -24.52223341984387872 ) ) ;
#9172=AXIS2_PLACEMENT_3D ( 'NONE', #9061, #7991, #11604 ) ;
#9173=CARTESIAN_POINT ( 'NONE',  ( 205.8264633344831225, 9.596613037118636669, -14.00000000000005507 ) ) ;
#9174=DIRECTION ( 'NONE',  ( -0.5000000000000049960, 0.8660254037844357100, -0.000000000000000000 ) ) ;
#9180=VECTOR ( 'NONE', #7917, 1000.000000000000000 ) ;
#9182=AXIS2_PLACEMENT_3D ( 'NONE', #106, #1584, #6536 ) ;
#9183=CARTESIAN_POINT ( 'NONE',  ( 208.4761278624580711, 5.007259451653140125, -14.00000000000005507 ) ) ;
#9185=VERTEX_POINT ( 'NONE', #5148 ) ;
#9190=ORIENTED_EDGE ( 'NONE', *, *, #15245, .T. ) ;
#9199=VERTEX_POINT ( 'NONE', #20945 ) ;
#9211=CARTESIAN_POINT ( 'NONE',  ( 215.8239785704504072, 15.89973041162422440, -14.39661757960083222 ) ) ;
#9213=VERTEX_POINT ( 'NONE', #5561 ) ;
#9217=ORIENTED_EDGE ( 'NONE', *, *, #14237, .T. ) ;
#9222=DIRECTION ( 'NONE',  ( 0.4758887346169484722, 0.2747544890354094993, 0.8354878114129318245 ) ) ;
#9223=ORIENTED_EDGE ( 'NONE', *, *, #19471, .F. ) ;
#9228=DIRECTION ( 'NONE',  ( -0.8660254037844357100, -0.5000000000000049960, 0.000000000000000000 ) ) ;
#9232=DIRECTION ( 'NONE',  ( 0.8660254037844352659, 0.5000000000000056621, 0.000000000000000000 ) ) ;
#9243=VERTEX_POINT ( 'NONE', #2401 ) ;
#9244=FACE_OUTER_BOUND ( 'NONE', #10737, .T. ) ;
#9248=DIRECTION ( 'NONE',  ( 0.8528685319524385022, 0.4924038765061083955, -0.1736481776669413224 ) ) ;
#9251=EDGE_CURVE ( 'NONE', #112, #3900, #707, .T. ) ;
#9252=CARTESIAN_POINT ( 'NONE',  ( 201.5219881633594525, 7.288445818786272845, -2.697891510991471176 ) ) ;
#9254=AXIS2_PLACEMENT_3D ( 'NONE', #2561, #9006, #6031 ) ;
#9259=DIRECTION ( 'NONE',  ( 0.5000000000000054401, -0.8660254037844354880, 0.000000000000000000 ) ) ;
#9262=CARTESIAN_POINT ( 'NONE',  ( 214.9645700193949267, 8.238142410745643573, -4.273921076953424603 ) ) ;
#9264=ORIENTED_EDGE ( 'NONE', *, *, #14603, .F. ) ;
#9266=VERTEX_POINT ( 'NONE', #18299 ) ;
#9270=DIRECTION ( 'NONE',  ( -0.8660254037844354880, -0.5000000000000055511, 0.000000000000000000 ) ) ;
#9272=ADVANCED_FACE ( 'NONE', ( #10332 ), #13539, .T. ) ;
#9275=ORIENTED_EDGE ( 'NONE', *, *, #3179, .F. ) ;
#9276=PLANE ( 'NONE',  #14559 ) ;
#9281=CONICAL_SURFACE ( 'NONE', #13034, 10.85470691220533190, 0.8171114040043576665 ) ;
#9283=DIRECTION ( 'NONE',  ( -0.5000000000000049960, 0.8660254037844358210, -0.000000000000000000 ) ) ;
#9286=ORIENTED_EDGE ( 'NONE', *, *, #4874, .F. ) ;
#9287=DIRECTION ( 'NONE',  ( -0.6634139481689433904, -0.3830222215594970003, -0.6427876096865293709 ) ) ;
#9288=DIRECTION ( 'NONE',  ( 0.8660254037844355990, 0.5000000000000054401, 1.237624392856779246E-14 ) ) ;
#9295=EDGE_LOOP ( 'NONE', ( #19035, #14000, #606, #7144 ) ) ;
#9298=CARTESIAN_POINT ( 'NONE',  ( 212.7427532632225962, 7.470596775315875071, -25.46066938576263894 ) ) ;
#9299=CARTESIAN_POINT ( 'NONE',  ( 208.7495889232816353, 11.81532964447897704, -12.17435723916119272 ) ) ;
#9304=B_SPLINE_CURVE_WITH_KNOTS ( 'NONE', 3,
 ( #2590, #7434, #13928, #5846 ),
 .UNSPECIFIED., .F., .F.,
 ( 4, 4 ),
 ( 4.349761613911982071E-05, 0.0008974833541226746782 ),
 .UNSPECIFIED. ) ;
#9305=LINE ( 'NONE', #17177, #16844 ) ;
#9307=VERTEX_POINT ( 'NONE', #915 ) ;
#9309=DIRECTION ( 'NONE',  ( -0.8660254037844360431, -0.5000000000000046629, 0.000000000000000000 ) ) ;
#9311=VERTEX_POINT ( 'NONE', #812 ) ;
#9314=EDGE_LOOP ( 'NONE', ( #6036, #15987, #6790, #5691 ) ) ;
#9318=VECTOR ( 'NONE', #18133, 1000.000000000000227 ) ;
#9319=ADVANCED_FACE ( 'NONE', ( #16919 ), #5436, .T. ) ;
#9327=CARTESIAN_POINT ( 'NONE',  ( 197.6726886235968834, -1.230109101077226486, -14.00000000000005507 ) ) ;
#9335=CARTESIAN_POINT ( 'NONE',  ( 197.5592321514251353, 4.823524888127141530, -22.03054070023847544 ) ) ;
#9343=CARTESIAN_POINT ( 'NONE',  ( 195.2585560139913810, 8.150276080056761074, -20.52105855319921446 ) ) ;
#9346=ORIENTED_EDGE ( 'NONE', *, *, #15861, .F. ) ;
#9349=CARTESIAN_POINT ( 'NONE',  ( 197.0236180130380319, 5.045337182940025755, -7.515250618841284869 ) ) ;
#9354=CARTESIAN_POINT ( 'NONE',  ( 200.8534188064670900, 11.38047161937165974, -2.669358488461094137 ) ) ;
#9356=CARTESIAN_POINT ( 'NONE',  ( 208.0983737146324870, 5.661548828456886895, -14.00000000000005507 ) ) ;
#9358=ORIENTED_EDGE ( 'NONE', *, *, #13560, .F. ) ;
#9363=ADVANCED_FACE ( 'NONE', ( #14391 ), #15564, .T. ) ;
#9364=DIRECTION ( 'NONE',  ( -0.5000000000000049960, 0.8660254037844357100, -0.000000000000000000 ) ) ;
#9370=VERTEX_POINT ( 'NONE', #1023 ) ;
#9372=CARTESIAN_POINT ( 'NONE',  ( 207.4970939194043922, 10.91519141264829429, -2.035916199211812216 ) ) ;
#9374=EDGE_CURVE ( 'NONE', #2644, #19458, #17448, .T. ) ;
#9376=CARTESIAN_POINT ( 'NONE',  ( 214.6606502076888034, 14.87405588687143698, -20.76014333877609275 ) ) ;
#9383=DIRECTION ( 'NONE',  ( -1.060575238724903217E-16, -6.123233995736827666E-17, 1.000000000000000000 ) ) ;
#9385=CARTESIAN_POINT ( 'NONE',  ( 215.0759710110270646, 15.29085814165182455, -19.44895743303496261 ) ) ;
#9389=ORIENTED_EDGE ( 'NONE', *, *, #2493, .F. ) ;
#9396=VERTEX_POINT ( 'NONE', #2927 ) ;
#9398=CARTESIAN_POINT ( 'NONE',  ( 198.6336827526812669, -1.448098972604089374, -15.39542905462715261 ) ) ;
#9401=CARTESIAN_POINT ( 'NONE',  ( 207.1242269781990331, 15.00092440535764560, -26.58724934764018855 ) ) ;
#9408=DIRECTION ( 'NONE',  ( -0.5000000000000049960, 0.8660254037844358210, -0.000000000000000000 ) ) ;
#9409=VECTOR ( 'NONE', #10894, 1000.000000000000114 ) ;
#9419=CARTESIAN_POINT ( 'NONE',  ( 206.8794782033451156, 3.312613250519402808, -26.96550585544242296 ) ) ;
#9423=EDGE_LOOP ( 'NONE', ( #7601, #12493, #3924, #17650, #11103, #3028 ) ) ;
#9424=VECTOR ( 'NONE', #10938, 1000.000000000000114 ) ;
#9429=B_SPLINE_CURVE_WITH_KNOTS ( 'NONE', 3,
 ( #14095, #3154, #7706, #12602 ),
 .UNSPECIFIED., .F., .F.,
 ( 4, 4 ),
 ( 7.698220069962578513E-05, 0.0007496329927527359965 ),
 .UNSPECIFIED. ) ;
#9431=ORIENTED_EDGE ( 'NONE', *, *, #6141, .T. ) ;
#9432=LINE ( 'NONE', #1502, #5005 ) ;
#9435=CYLINDRICAL_SURFACE ( 'NONE', #6102, 12.47473710546057646 ) ;
#9438=CARTESIAN_POINT ( 'NONE',  ( 199.2243387870319395, 21.03182819120163671, -14.00000000000005507 ) ) ;
#9440=CARTESIAN_POINT ( 'NONE',  ( 190.9298951392057120, 16.26579628913994213, -5.993340328401665751 ) ) ;
#9444=CARTESIAN_POINT ( 'NONE',  ( 218.4477085251713504, 9.991534140873421066, -9.972943347742013742 ) ) ;
#9447=LINE ( 'NONE', #35, #5019 ) ;
#9449=ORIENTED_EDGE ( 'NONE', *, *, #6861, .F. ) ;
#9450=ORIENTED_EDGE ( 'NONE', *, *, #4975, .F. ) ;
#9452=AXIS2_PLACEMENT_3D ( 'NONE', #17149, #15681, #12065 ) ;
#9454=AXIS2_PLACEMENT_3D ( 'NONE', #4532, #12804, #4733 ) ;
#9456=ORIENTED_EDGE ( 'NONE', *, *, #15898, .F. ) ;
#9457=EDGE_CURVE ( 'NONE', #15788, #2452, #6792, .T. ) ;
#9462=ORIENTED_EDGE ( 'NONE', *, *, #12642, .T. ) ;
#9463=CARTESIAN_POINT ( 'NONE',  ( 200.1605181682011221, -0.5665801344454006738, -7.448751785191272567 ) ) ;
#9466=AXIS2_PLACEMENT_3D ( 'NONE', #18483, #3955, #10404 ) ;
#9467=CARTESIAN_POINT ( 'NONE',  ( 203.9637611243273057, 8.521181414665040421, -26.28791492288515386 ) ) ;
#9468=CARTESIAN_POINT ( 'NONE',  ( 199.3642739955437833, 5.865666282727633352, -4.003039906353938804 ) ) ;
#9473=DIRECTION ( 'NONE',  ( -0.8660254037844355990, -0.5000000000000055511, 0.000000000000000000 ) ) ;
#9475=FACE_OUTER_BOUND ( 'NONE', #7100, .T. ) ;
#9481=ORIENTED_EDGE ( 'NONE', *, *, #9109, .T. ) ;
#9485=EDGE_CURVE ( 'NONE', #1053, #6174, #14704, .T. ) ;
#9488=CARTESIAN_POINT ( 'NONE',  ( 215.0768188481721381, 15.46835754483921832, -19.61062504997882172 ) ) ;
#9490=DIRECTION ( 'NONE',  ( -0.5000000000000027756, 0.8660254037844372643, -0.000000000000000000 ) ) ;
#9493=AXIS2_PLACEMENT_3D ( 'NONE', #4267, #7541, #14033 ) ;
#9497=AXIS2_PLACEMENT_3D ( 'NONE', #3466, #1672, #20840 ) ;
#9500=CARTESIAN_POINT ( 'NONE',  ( 197.7441788599589074, -1.188834193869147571, -15.43274561385865873 ) ) ;
#9508=CARTESIAN_POINT ( 'NONE',  ( 195.2241281744312857, 3.829391336032939908, -15.41371838794996840 ) ) ;
#9510=CARTESIAN_POINT ( 'NONE',  ( 208.8107687779841228, 4.427644383670616079, -14.00000000000005507 ) ) ;
#9513=LINE ( 'NONE', #14422, #9035 ) ;
#9515=AXIS2_PLACEMENT_3D ( 'NONE', #63, #4824, #1447 ) ;
#9516=PLANE ( 'NONE',  #11813 ) ;
#9525=FACE_OUTER_BOUND ( 'NONE', #893, .T. ) ;
#9526=ORIENTED_EDGE ( 'NONE', *, *, #18549, .F. ) ;
#9529=ORIENTED_EDGE ( 'NONE', *, *, #307, .F. ) ;
#9535=VECTOR ( 'NONE', #20382, 1000.000000000000114 ) ;
#9539=EDGE_CURVE ( 'NONE', #19576, #12179, #16078, .T. ) ;
#9546=FACE_OUTER_BOUND ( 'NONE', #14624, .T. ) ;
#9548=VECTOR ( 'NONE', #18378, 1000.000000000000114 ) ;
#9554=LINE ( 'NONE', #14257, #20344 ) ;
#9557=CARTESIAN_POINT ( 'NONE',  ( 212.8960219706529813, 6.786266414165766925, -3.025685634606239294 ) ) ;
#9561=VERTEX_POINT ( 'NONE', #6701 ) ;
#9562=ORIENTED_EDGE ( 'NONE', *, *, #10951, .F. ) ;
#9572=ORIENTED_EDGE ( 'NONE', *, *, #19257, .F. ) ;
#9574=CARTESIAN_POINT ( 'NONE',  ( 210.3388300726135753, 6.082691074106562290, -26.28791492288521425 ) ) ;
#9576=ORIENTED_EDGE ( 'NONE', *, *, #9648, .F. ) ;
#9579=ORIENTED_EDGE ( 'NONE', *, *, #4504, .F. ) ;
#9581=EDGE_LOOP ( 'NONE', ( #8624, #11413, #13538, #2195 ) ) ;
#9583=DIRECTION ( 'NONE',  ( 0.8660254037844352659, 0.5000000000000056621, 0.000000000000000000 ) ) ;
#9584=DIRECTION ( 'NONE',  ( 0.5000000000000051070, -0.8660254037844359321, 0.000000000000000000 ) ) ;
#9586=EDGE_CURVE ( 'NONE', #12995, #17291, #1545, .T. ) ;
#9588=VECTOR ( 'NONE', #10483, 1000.000000000000114 ) ;
#9591=CARTESIAN_POINT ( 'NONE',  ( 211.7320635740234422, 6.114254720546163924, -25.34310559273333396 ) ) ;
#9595=DIRECTION ( 'NONE',  ( -0.8660254037844354880, -0.5000000000000055511, 0.000000000000000000 ) ) ;
#9602=ORIENTED_EDGE ( 'NONE', *, *, #10043, .T. ) ;
#9603=CONICAL_SURFACE ( 'NONE', #4206, 4.389613146203297234, 1.047197551196619614 ) ;
#9604=CARTESIAN_POINT ( 'NONE',  ( 218.9149645394843731, 10.51890375032455438, -16.79062062844375092 ) ) ;
#9613=CARTESIAN_POINT ( 'NONE',  ( 214.1110484215691656, 14.37972046727219144, -5.993340328401894013 ) ) ;
#9615=EDGE_CURVE ( 'NONE', #18407, #16739, #19436, .T. ) ;
#9623=CARTESIAN_POINT ( 'NONE',  ( 198.0735972701637024, -1.389238810292188875, -14.00000000000005507 ) ) ;
#9626=EDGE_LOOP ( 'NONE', ( #16308, #20367, #12729, #6419 ) ) ;
#9628=DIRECTION ( 'NONE',  ( -0.4758887346169485832, -0.2747544890354092773, -0.8354878114129317135 ) ) ;
#9643=ORIENTED_EDGE ( 'NONE', *, *, #13388, .T. ) ;
#9644=EDGE_CURVE ( 'NONE', #8299, #17056, #2426, .T. ) ;
#9648=EDGE_CURVE ( 'NONE', #5150, #3223, #20072, .T. ) ;
#9650=DIRECTION ( 'NONE',  ( 0.8660254037844355990, 0.5000000000000054401, 0.000000000000000000 ) ) ;
#9657=AXIS2_PLACEMENT_3D ( 'NONE', #4456, #6027, #13791 ) ;
#9658=B_SPLINE_CURVE_WITH_KNOTS ( 'NONE', 3,
 ( #16550, #2032, #1930, #8376 ),
 .UNSPECIFIED., .F., .F.,
 ( 4, 4 ),
 ( 4.692417266935620115E-07, 0.0008544549797101211232 ),
 .UNSPECIFIED. ) ;
#9661=CARTESIAN_POINT ( 'NONE',  ( 209.3990796341988982, 4.767305814873403769, -25.92587471718750436 ) ) ;
#9667=AXIS2_PLACEMENT_3D ( 'NONE', #1029, #7791, #7484 ) ;
#9668=EDGE_CURVE ( 'NONE', #18332, #6104, #16306, .T. ) ;
#9673=CARTESIAN_POINT ( 'NONE',  ( 215.9829844511909300, 15.46048323788008361, -18.25196083293883120 ) ) ;
#9674=EDGE_CURVE ( 'NONE', #4463, #5382, #10395, .T. ) ;
#9680=DIRECTION ( 'NONE',  ( 0.8944271909999204073, 0.000000000000000000, 0.4472135954999487684 ) ) ;
#9681=PLANE ( 'NONE',  #4748 ) ;
#9682=AXIS2_PLACEMENT_3D ( 'NONE', #4412, #12585, #20731 ) ;
#9683=ORIENTED_EDGE ( 'NONE', *, *, #5654, .T. ) ;
#9686=VERTEX_POINT ( 'NONE', #13620 ) ;
#9692=ORIENTED_EDGE ( 'NONE', *, *, #3584, .T. ) ;
#9693=VECTOR ( 'NONE', #18231, 1000.000000000000114 ) ;
#9694=CIRCLE ( 'NONE', #12091, 12.47473710546057823 ) ;
#9695=DIRECTION ( 'NONE',  ( 0.8426815769442687065, 0.4865224352899185645, 0.2306158707424266763 ) ) ;
#9696=CARTESIAN_POINT ( 'NONE',  ( 209.3617675235332740, 26.90744277190043476, -9.718744748713266546 ) ) ;
#9698=CARTESIAN_POINT ( 'NONE',  ( 203.5446072452137685, 23.54890371929340631, -14.00000000000005507 ) ) ;
#9702=EDGE_LOOP ( 'NONE', ( #1670, #17803, #13283, #11406, #8788 ) ) ;
#9708=VERTEX_POINT ( 'NONE', #19852 ) ;
#9716=ORIENTED_EDGE ( 'NONE', *, *, #11585, .T. ) ;
#9718=VERTEX_POINT ( 'NONE', #18590 ) ;
#9719=DIRECTION ( 'NONE',  ( -0.5000000000000049960, 0.8660254037844358210, -0.000000000000000000 ) ) ;
#9723=CARTESIAN_POINT ( 'NONE',  ( 205.8264633344831225, 9.596613037118636669, -14.00000000000005507 ) ) ;
#9729=AXIS2_PLACEMENT_3D ( 'NONE', #782, #15327, #13716 ) ;
#9736=ORIENTED_EDGE ( 'NONE', *, *, #17593, .F. ) ;
#9737=CARTESIAN_POINT ( 'NONE',  ( 207.9729903995531402, 4.459159050239305699, -1.722272971484193782 ) ) ;
#9740=CARTESIAN_POINT ( 'NONE',  ( 205.0662616026534693, 10.91332106064940888, -14.00000000000005507 ) ) ;
#9750=CARTESIAN_POINT ( 'NONE',  ( 194.3181527907504176, 7.607334025971792535, -6.724618537539360119 ) ) ;
#9752=CARTESIAN_POINT ( 'NONE',  ( 206.8805578665094345, 3.570835818144959539, -2.061577111287765440 ) ) ;
#9756=VERTEX_POINT ( 'NONE', #10088 ) ;
#9759=SHAPE_REPRESENTATION ( 'Drill Bit Indexing Pin', ( #18233 ), #3328 ) ;
#9762=ORIENTED_EDGE ( 'NONE', *, *, #19246, .F. ) ;
#9769=CARTESIAN_POINT ( 'NONE',  ( 215.8017975273770332, 15.88692418043490306, -12.80378922971585887 ) ) ;
#9775=EDGE_CURVE ( 'NONE', #6868, #12264, #19956, .T. ) ;
#9778=VERTEX_POINT ( 'NONE', #17423 ) ;
#9781=AXIS2_PLACEMENT_3D ( 'NONE', #18742, #4107, #20114 ) ;
#9784=EDGE_CURVE ( 'NONE', #13943, #8036, #12660, .T. ) ;
#9785=ORIENTED_EDGE ( 'NONE', *, *, #9794, .T. ) ;
#9789=CARTESIAN_POINT ( 'NONE',  ( 216.7435376666127240, 9.522836875816564017, -21.90921222372436006 ) ) ;
#9794=EDGE_CURVE ( 'NONE', #15101, #15382, #9134, .T. ) ;
#9797=AXIS2_PLACEMENT_3D ( 'NONE', #2922, #9364, #1541 ) ;
#9804=ADVANCED_FACE ( 'NONE', ( #15640 ), #16321, .T. ) ;
#9816=CARTESIAN_POINT ( 'NONE',  ( 213.5401130648333492, 14.58114004716331280, -6.286464976499002155 ) ) ;
#9817=ORIENTED_EDGE ( 'NONE', *, *, #1968, .T. ) ;
#9823=VECTOR ( 'NONE', #18719, 1000.000000000000114 ) ;
#9824=CONICAL_SURFACE ( 'NONE', #377, 13.07248899748297433, 0.6693469023067423196 ) ;
#9825=CARTESIAN_POINT ( 'NONE',  ( 197.9399629305378880, -1.336196318472940181, -14.00519586093461832 ) ) ;
#9830=VECTOR ( 'NONE', #6169, 1000.000000000000000 ) ;
#9835=CARTESIAN_POINT ( 'NONE',  ( 215.5644888513662067, 15.74991395245902304, -11.24974199967302013 ) ) ;
#9836=CARTESIAN_POINT ( 'NONE',  ( 199.5722073119862046, -0.9062415656482646353, -8.625373497621064089 ) ) ;
#9840=AXIS2_PLACEMENT_3D ( 'NONE', #2690, #7651, #14037 ) ;
#9841=CONICAL_SURFACE ( 'NONE', #728, 10.85470691220533190, 0.8171114040043576665 ) ;
#9843=CARTESIAN_POINT ( 'NONE',  ( 213.9139752855751055, 14.44296291959195955, -21.91826003371448905 ) ) ;
#9845=ADVANCED_FACE ( 'NONE', ( #1204 ), #15538, .F. ) ;
#9847=CARTESIAN_POINT ( 'NONE',  ( 208.8107687779841228, 4.427644383670616079, -14.00000000000005507 ) ) ;
#9849=CARTESIAN_POINT ( 'NONE',  ( 205.0662616026534693, 10.91332106064940888, -14.00000000000005507 ) ) ;
#9854=ORIENTED_EDGE ( 'NONE', *, *, #9615, .T. ) ;
#9856=DIRECTION ( 'NONE',  ( -0.5000000000000054401, 0.8660254037844354880, -0.000000000000000000 ) ) ;
#9860=CARTESIAN_POINT ( 'NONE',  ( 206.8720745992954164, 3.565938001535339907, -25.93669565428267276 ) ) ;
#9862=ORIENTED_EDGE ( 'NONE', *, *, #20095, .F. ) ;
#9863=ORIENTED_EDGE ( 'NONE', *, *, #15060, .T. ) ;
#9864=VERTEX_POINT ( 'NONE', #2594 ) ;
#9868=VERTEX_POINT ( 'NONE', #995 ) ;
#9869=B_SPLINE_CURVE_WITH_KNOTS ( 'NONE', 3,
 ( #1249, #7696, #14197, #4529 ),
 .UNSPECIFIED., .F., .F.,
 ( 4, 4 ),
 ( 9.410049375302480474E-05, 0.0007667512858034030571 ),
 .UNSPECIFIED. ) ;
#9870=CARTESIAN_POINT ( 'NONE',  ( 196.9311089575304266, 4.991927054840251010, -20.59651891138145174 ) ) ;
#9873=FACE_OUTER_BOUND ( 'NONE', #5360, .T. ) ;
#9874=DIRECTION ( 'NONE',  ( 0.5000000000000049960, -0.8660254037844358210, 0.000000000000000000 ) ) ;
#9876=ADVANCED_FACE ( 'NONE', ( #14263 ), #14043, .T. ) ;
#9884=VECTOR ( 'NONE', #12962, 1000.000000000000114 ) ;
#9886=AXIS2_PLACEMENT_3D ( 'NONE', #16898, #15230, #18494 ) ;
#9890=CARTESIAN_POINT ( 'NONE',  ( 209.6243204174557206, 3.018531609524862880, -14.00000000000005507 ) ) ;
#9891=EDGE_CURVE ( 'NONE', #3202, #10176, #1312, .T. ) ;
#9898=CONICAL_SURFACE ( 'NONE', #3490, 10.85470691220533190, 0.8171114040043576665 ) ;
#9902=DIRECTION ( 'NONE',  ( 0.5000000000000049960, -0.8660254037844358210, 0.000000000000000000 ) ) ;
#9915=CARTESIAN_POINT ( 'NONE',  ( 198.5622009498131604, -1.489369010732141785, -13.97827067520021593 ) ) ;
#9918=AXIS2_PLACEMENT_3D ( 'NONE', #15880, #14199, #6100 ) ;
#9927=DIRECTION ( 'NONE',  ( -0.8601696498176549799, -0.4966191788709765631, 0.1160929141252379365 ) ) ;
#9935=ORIENTED_EDGE ( 'NONE', *, *, #19252, .F. ) ;
#9940=EDGE_LOOP ( 'NONE', ( #13228, #12978, #8460, #10527, #4829, #19783 ) ) ;
#9945=DIRECTION ( 'NONE',  ( -0.8660254037844355990, -0.5000000000000055511, 0.000000000000000000 ) ) ;
#9949=CARTESIAN_POINT ( 'NONE',  ( 199.2144802262915846, 21.04890371929339921, -14.00000000000005507 ) ) ;
#9952=ORIENTED_EDGE ( 'NONE', *, *, #19632, .T. ) ;
#9953=DIRECTION ( 'NONE',  ( 0.7499999999999953371, 0.4330127018922228510, -0.5000000000000038858 ) ) ;
#9959=VERTEX_POINT ( 'NONE', #13790 ) ;
#9963=VERTEX_POINT ( 'NONE', #5601 ) ;
#9964=CARTESIAN_POINT ( 'NONE',  ( 199.2144802262915846, 21.04890371929339921, -14.00000000000005507 ) ) ;
#9965=CLOSED_SHELL ( 'NONE', ( #2365, #3631, #13510, #880, #6018, #4465, #1491, #10128, #7948, #12257, #5267, #3449, #19496, #2436, #14879, #20049, #16348, #3826, #10519, #8852, #5369, #4982, #4805, #7016, #8871, #20543, #3813, #9363, #9272, #18112, #7562, #18886, #2314, #12193, #5894, #9876, #4214, #17579, #754, #13660, #12085, #11019, #15237, #10889, #16490, #3536, #15631, #19643, #5762, #4252, #8525, #1506, #4382, #2886, #13659, #4709, #7057, #6288, #4354, #4490, #8988, #19204, #12410, #15727, #13325, #109, #16381, #19832, #17069, #11106, #12929, #10945, #7526, #17068, #6901, #18868, #3666, #10279, #18820, #14135, #19856, #13817, #19509, #5340, #10691, #605, #887, #1790, #4610, #985, #1636, #15988, #16168, #9845, #20703, #19031, #5455, #10919, #6758, #17920, #18681, #10618, #5224, #16432, #14982, #4978, #7853, #17301, #6146, #11720, #19258, #9065, #1867, #12366, #16756, #16047, #13054, #8474, #17530, #5963, #5479, #882, #11887, #1348, #19136, #10036, #7957, #19448, #18424, #234, #19473, #11225, #7719, #6773, #4123, #15010, #1959, #6744, #13508, #19527, #2354, #20423, #13150, #9319, #12842, #6342, #8601, #15229, #11852, #12798, #5917, #11293, #4108, #20267, #6405, #4989, #9804, #16051, #16058, #19342, #19109, #1825, #5120, #360, #15326, #12409, #11283, #12857, #13574, #19393, #5856, #12296, #16880, #13041, #3391, #16640, #15644, #2308, #17171, #11711, #11603, #10981, #10292, #14035, #17290, #2549, #593 ) ) ;
#9969=ORIENTED_EDGE ( 'NONE', *, *, #11860, .T. ) ;
#9972=CARTESIAN_POINT ( 'NONE',  ( 213.7874248973967610, 18.84792351767029572, -16.70797078425240656 ) ) ;
#9982=ORIENTED_EDGE ( 'NONE', *, *, #13837, .F. ) ;
#9983=CONICAL_SURFACE ( 'NONE', #3928, 10.85470691220533190, 0.8171114040043576665 ) ;
#9986=VECTOR ( 'NONE', #5919, 1000.000000000000227 ) ;
#9989=DIRECTION ( 'NONE',  ( 0.1503837331804444566, 0.08682408883347132733, 0.9848077530122061329 ) ) ;
#9990=ORIENTED_EDGE ( 'NONE', *, *, #2788, .T. ) ;
#9996=VECTOR ( 'NONE', #10121, 999.9999999999998863 ) ;
#10001=DIRECTION ( 'NONE',  ( 0.8660254037844352659, 0.5000000000000056621, 0.000000000000000000 ) ) ;
#10004=CARTESIAN_POINT ( 'NONE',  ( 205.8564897284660731, 2.721990579170014080, -25.44774858730788125 ) ) ;
#10006=ORIENTED_EDGE ( 'NONE', *, *, #20871, .T. ) ;
#10013=EDGE_LOOP ( 'NONE', ( #20207, #19435, #635, #1863 ) ) ;
#10014=VERTEX_POINT ( 'NONE', #16968 ) ;
#10016=CARTESIAN_POINT ( 'NONE',  ( 197.3517780161357678, 19.97347209683980296, -26.28791492288515386 ) ) ;
#10024=FACE_OUTER_BOUND ( 'NONE', #4895, .T. ) ;
#10026=FACE_OUTER_BOUND ( 'NONE', #17629, .T. ) ;
#10032=AXIS2_PLACEMENT_3D ( 'NONE', #5383, #16957, #11985 ) ;
#10033=VECTOR ( 'NONE', #3074, 1000.000000000000114 ) ;
#10036=ADVANCED_FACE ( 'NONE', ( #15190 ), #15086, .F. ) ;
#10040=ORIENTED_EDGE ( 'NONE', *, *, #14071, .F. ) ;
#10041=FACE_OUTER_BOUND ( 'NONE', #11583, .T. ) ;
#10043=EDGE_CURVE ( 'NONE', #12385, #18641, #2342, .T. ) ;
#10046=EDGE_CURVE ( 'NONE', #6001, #1760, #14225, .T. ) ;
#10053=DIRECTION ( 'NONE',  ( -0.5000000000000054401, 0.8660254037844354880, -0.000000000000000000 ) ) ;
#10057=PLANE ( 'NONE',  #17361 ) ;
#10058=VERTEX_POINT ( 'NONE', #4557 ) ;
#10060=CARTESIAN_POINT ( 'NONE',  ( 206.1736271717860234, 10.32809743383080558, -25.81526893633800412 ) ) ;
#10061=CARTESIAN_POINT ( 'NONE',  ( 218.0611881365336444, 9.768376490446161853, -19.34736286182901210 ) ) ;
#10072=ORIENTED_EDGE ( 'NONE', *, *, #10460, .T. ) ;
#10073=PLANE ( 'NONE',  #4950 ) ;
#10078=CARTESIAN_POINT ( 'NONE',  ( 201.7914626300884890, 0.3750460896586316206, -22.62267072728657524 ) ) ;
#10088=CARTESIAN_POINT ( 'NONE',  ( 207.3262688097345574, 1.076026043308923930, -14.00000000000005507 ) ) ;
#10090=ORIENTED_EDGE ( 'NONE', *, *, #18211, .F. ) ;
#10091=VECTOR ( 'NONE', #13607, 1000.000000000000000 ) ;
#10093=CARTESIAN_POINT ( 'NONE',  ( 193.5622009498131035, 7.170885027112213983, -13.97827067520021416 ) ) ;
#10095=LINE ( 'NONE', #7033, #7322 ) ;
#10106=FACE_OUTER_BOUND ( 'NONE', #7945, .T. ) ;
#10111=CARTESIAN_POINT ( 'NONE',  ( 205.3647371392095806, 3.210897180031505371, -25.94618751764486575 ) ) ;
#10119=CARTESIAN_POINT ( 'NONE',  ( 195.2863413965735333, 4.042320060767385037, -12.62152863576138806 ) ) ;
#10121=DIRECTION ( 'NONE',  ( 0.4758887346169385357, 0.2747544890354034486, -0.8354878114129393740 ) ) ;
#10127=CONICAL_SURFACE ( 'NONE', #15266, 13.07248899748297433, 0.6693469023067423196 ) ;
#10128=ADVANCED_FACE ( 'NONE', ( #9100 ), #12720, .T. ) ;
#10130=CARTESIAN_POINT ( 'NONE',  ( 209.6971420603676677, 12.36239970324706050, -2.990331769139234375 ) ) ;
#10136=EDGE_CURVE ( 'NONE', #12995, #20836, #19183, .T. ) ;
#10137=ORIENTED_EDGE ( 'NONE', *, *, #307, .T. ) ;
#10146=CONICAL_SURFACE ( 'NONE', #697, 10.85470691220533190, 0.8171114040043576665 ) ;
#10147=ORIENTED_EDGE ( 'NONE', *, *, #19759, .T. ) ;
#10151=VERTEX_POINT ( 'NONE', #7927 ) ;
#10152=AXIS2_PLACEMENT_3D ( 'NONE', #3403, #9856, #8059 ) ;
#10158=CARTESIAN_POINT ( 'NONE',  ( 207.6891655446386551, 10.67204465957205350, -26.28791492288521781 ) ) ;
#10162=DIRECTION ( 'NONE',  ( -0.8660254037844357100, -0.5000000000000051070, 0.000000000000000000 ) ) ;
#10163=DIRECTION ( 'NONE',  ( 0.3886714912512298503, 0.2243995901002338311, 0.8936326403234118310 ) ) ;
#10167=CIRCLE ( 'NONE', #6446, 11.98469917212512215 ) ;
#10168=CIRCLE ( 'NONE', #5094, 12.47473710546057823 ) ;
#10174=ORIENTED_EDGE ( 'NONE', *, *, #3972, .F. ) ;
#10176=VERTEX_POINT ( 'NONE', #12515 ) ;
#10180=ORIENTED_EDGE ( 'NONE', *, *, #118, .T. ) ;
#10182=EDGE_CURVE ( 'NONE', #17941, #14915, #18976, .T. ) ;
#10187=VECTOR ( 'NONE', #19858, 1000.000000000000227 ) ;
#10191=DIRECTION ( 'NONE',  ( -0.5000000000000054401, 0.8660254037844354880, -0.000000000000000000 ) ) ;
#10193=VERTEX_POINT ( 'NONE', #16322 ) ;
#10199=ORIENTED_EDGE ( 'NONE', *, *, #18715, .T. ) ;
#10202=PLANE ( 'NONE',  #16320 ) ;
#10204=DIRECTION ( 'NONE',  ( 0.8296432542242785368, 0.4789947561577507784, 0.2868032327110803803 ) ) ;
#10206=AXIS2_PLACEMENT_3D ( 'NONE', #13242, #14646, #2000 ) ;
#10207=DIRECTION ( 'NONE',  ( 0.5000000000000055511, -0.8660254037844353769, 2.220446049250313574E-16 ) ) ;
#10215=DIRECTION ( 'NONE',  ( 0.5000000000000051070, -0.8660254037844359321, 0.000000000000000000 ) ) ;
#10218=AXIS2_PLACEMENT_3D ( 'NONE', #4482, #4372, #20579 ) ;
#10219=DIRECTION ( 'NONE',  ( 0.5000000000000054401, -0.8660254037844354880, -1.665334536937734318E-16 ) ) ;
#10220=CARTESIAN_POINT ( 'NONE',  ( 210.3654177961080052, 6.098041503423209164, -1.717498466822859227 ) ) ;
#10221=DIRECTION ( 'NONE',  ( -0.8660254037844355990, -0.5000000000000055511, 0.000000000000000000 ) ) ;
#10228=EDGE_CURVE ( 'NONE', #19879, #5830, #16497, .T. ) ;
#10232=DIRECTION ( 'NONE',  ( -0.8660254037844355990, -0.5000000000000055511, 0.000000000000000000 ) ) ;
#10235=CARTESIAN_POINT ( 'NONE',  ( 208.5625094892126583, 11.70731928285941770, -25.48492467622476099 ) ) ;
#10236=VECTOR ( 'NONE', #16120, 1000.000000000000114 ) ;
#10242=DIRECTION ( 'NONE',  ( -0.3886714912512189701, -0.2243995901002275584, 0.8936326403234180482 ) ) ;
#10244=DIRECTION ( 'NONE',  ( 0.5000000000000049960, -0.8660254037844358210, 0.000000000000000000 ) ) ;
#10245=FACE_OUTER_BOUND ( 'NONE', #8573, .T. ) ;
#10251=ORIENTED_EDGE ( 'NONE', *, *, #11700, .T. ) ;
#10252=EDGE_CURVE ( 'NONE', #20929, #13537, #16118, .T. ) ;
#10253=ORIENTED_EDGE ( 'NONE', *, *, #9586, .T. ) ;
#10259=CARTESIAN_POINT ( 'NONE',  ( 213.7342555843919740, 14.51621837890814248, -21.80597602412992231 ) ) ;
#10260=ORIENTED_EDGE ( 'NONE', *, *, #14833, .T. ) ;
#10261=VECTOR ( 'NONE', #9116, 1000.000000000000000 ) ;
#10268=EDGE_CURVE ( 'NONE', #2368, #10684, #3777, .T. ) ;
#10270=CARTESIAN_POINT ( 'NONE',  ( 208.9513496856693564, 16.05581419235814522, -3.762296834228893605 ) ) ;
#10271=CARTESIAN_POINT ( 'NONE',  ( 205.0662616026534693, 10.91332106064940888, -14.00000000000005507 ) ) ;
#10275=VERTEX_POINT ( 'NONE', #13136 ) ;
#10278=DIRECTION ( 'NONE',  ( -0.8660254037844357100, -0.5000000000000053291, 0.000000000000000000 ) ) ;
#10279=ADVANCED_FACE ( 'NONE', ( #8236 ), #1, .F. ) ;
#10282=EDGE_CURVE ( 'NONE', #8359, #6033, #5143, .T. ) ;
#10288=CARTESIAN_POINT ( 'NONE',  ( 198.4659246047362444, -1.544954184478863901, -13.98474561060102772 ) ) ;
#10292=ADVANCED_FACE ( 'NONE', ( #10026 ), #19703, .T. ) ;
#10293=CARTESIAN_POINT ( 'NONE',  ( 195.6198561393837281, 4.234874887307574554, -16.70797078425209037 ) ) ;
#10296=FACE_OUTER_BOUND ( 'NONE', #3690, .T. ) ;
#10298=DIRECTION ( 'NONE',  ( 0.8660254037844355990, 0.5000000000000054401, 3.017578575841809918E-14 ) ) ;
#10300=EDGE_CURVE ( 'NONE', #6800, #15885, #19476, .T. ) ;
#10301=ORIENTED_EDGE ( 'NONE', *, *, #4581, .F. ) ;
#10302=EDGE_LOOP ( 'NONE', ( #11587, #242, #14835, #15855 ) ) ;
#10303=ORIENTED_EDGE ( 'NONE', *, *, #8772, .F. ) ;
#10307=EDGE_CURVE ( 'NONE', #310, #11827, #3581, .T. ) ;
#10310=VECTOR ( 'NONE', #1977, 1000.000000000000227 ) ;
#10314=EDGE_CURVE ( 'NONE', #8036, #17291, #3482, .T. ) ;
#10322=CARTESIAN_POINT ( 'NONE',  ( 214.8600158830803650, 14.81213703278996618, -20.84195174293595443 ) ) ;
#10325=CARTESIAN_POINT ( 'NONE',  ( 205.8264633344831225, 9.596613037118636669, -14.00000000000005507 ) ) ;
#10328=ORIENTED_EDGE ( 'NONE', *, *, #10136, .T. ) ;
#10329=ORIENTED_EDGE ( 'NONE', *, *, #4219, .T. ) ;
#10332=FACE_OUTER_BOUND ( 'NONE', #17605, .T. ) ;
#10334=DIRECTION ( 'NONE',  ( 0.6958540455341891695, 0.000000000000000000, -0.7181832268395738073 ) ) ;
#10335=VERTEX_POINT ( 'NONE', #15474 ) ;
#10336=ORIENTED_EDGE ( 'NONE', *, *, #15536, .F. ) ;
#10347=FACE_OUTER_BOUND ( 'NONE', #19799, .T. ) ;
#10351=CARTESIAN_POINT ( 'NONE',  ( 218.6234151596997322, 10.86579850426016769, -9.718744748713266546 ) ) ;
#10353=ORIENTED_EDGE ( 'NONE', *, *, #6403, .F. ) ;
#10357=ORIENTED_EDGE ( 'NONE', *, *, #16067, .T. ) ;
#10358=AXIS2_PLACEMENT_3D ( 'NONE', #14529, #19278, #4746 ) ;
#10364=VERTEX_POINT ( 'NONE', #10130 ) ;
#10369=CONICAL_SURFACE ( 'NONE', #1262, 10.85470691220533190, 0.8171114040043576665 ) ;
#10372=DIRECTION ( 'NONE',  ( -0.5000000000000051070, 0.8660254037844359321, -0.000000000000000000 ) ) ;
#10374=VERTEX_POINT ( 'NONE', #620 ) ;
#10376=EDGE_CURVE ( 'NONE', #10497, #6334, #20726, .T. ) ;
#10379=ORIENTED_EDGE ( 'NONE', *, *, #7216, .F. ) ;
#10381=ORIENTED_EDGE ( 'NONE', *, *, #18902, .F. ) ;
#10383=DIRECTION ( 'NONE',  ( 0.5000000000000052180, -0.8660254037844355990, 0.000000000000000000 ) ) ;
#10384=AXIS2_PLACEMENT_3D ( 'NONE', #5255, #296, #19382 ) ;
#10386=VECTOR ( 'NONE', #16073, 1000.000000000000114 ) ;
#10388=ORIENTED_EDGE ( 'NONE', *, *, #11253, .F. ) ;
#10391=CARTESIAN_POINT ( 'NONE',  ( 211.6467004136641208, 6.580176515810935989, -25.78004855466132739 ) ) ;
#10395=B_SPLINE_CURVE_WITH_KNOTS ( 'NONE', 3,
 ( #5423, #12024, #15222, #16892 ),
 .UNSPECIFIED., .F., .F.,
 ( 4, 4 ),
 ( 7.218489860149274802E-05, 0.0007448356906551951507 ),
 .UNSPECIFIED. ) ;
#10397=CARTESIAN_POINT ( 'NONE',  ( 219.1657043289025921, 10.92127545031173774, -12.56699194733521097 ) ) ;
#10399=CARTESIAN_POINT ( 'NONE',  ( 211.2398691629905159, 12.72204434944011986, -24.79563718815145279 ) ) ;
#10404=DIRECTION ( 'NONE',  ( -0.8660254037844357100, -0.5000000000000051070, 0.000000000000000000 ) ) ;
#10406=DIRECTION ( 'NONE',  ( 0.8660254037844352659, 0.5000000000000056621, 0.000000000000000000 ) ) ;
#10409=FACE_BOUND ( 'NONE', #20530, .T. ) ;
#10412=ORIENTED_EDGE ( 'NONE', *, *, #2131, .T. ) ;
#10414=DIRECTION ( 'NONE',  ( -0.8660254037844355990, -0.5000000000000054401, 8.343535232742331521E-16 ) ) ;
#10418=AXIS2_PLACEMENT_3D ( 'NONE', #16774, #2255, #18471 ) ;
#10421=DIRECTION ( 'NONE',  ( 0.8404609622712050365, 0.000000000000000000, 0.5418720982834971389 ) ) ;
#10430=EDGE_CURVE ( 'NONE', #5830, #2244, #8669, .T. ) ;
#10431=FACE_OUTER_BOUND ( 'NONE', #811, .T. ) ;
#10433=CARTESIAN_POINT ( 'NONE',  ( 200.2378745322256464, -0.5219184168523266498, -7.515250618841284869 ) ) ;
#10434=EDGE_CURVE ( 'NONE', #20411, #9561, #19794, .T. ) ;
#10436=ORIENTED_EDGE ( 'NONE', *, *, #15159, .T. ) ;
#10438=DIRECTION ( 'NONE',  ( 0.5000000000000052180, -0.8660254037844355990, 1.665334536937734318E-16 ) ) ;
#10440=VERTEX_POINT ( 'NONE', #13763 ) ;
#10443=CARTESIAN_POINT ( 'NONE',  ( 209.4659469037960093, 16.35291703476779546, -2.579136038830255107 ) ) ;
#10444=B_SPLINE_CURVE_WITH_KNOTS ( 'NONE', 3,
 ( #3250, #5042, #14831, #5246 ),
 .UNSPECIFIED., .F., .F.,
 ( 4, 4 ),
 ( 8.982943871858821536E-05, 0.0009438151766972277881 ),
 .UNSPECIFIED. ) ;
#10446=PLANE ( 'NONE',  #11030 ) ;
#10450=EDGE_CURVE ( 'NONE', #8387, #2861, #18360, .T. ) ;
#10457=ORIENTED_EDGE ( 'NONE', *, *, #6789, .F. ) ;
#10460=EDGE_CURVE ( 'NONE', #3882, #20176, #8773, .T. ) ;
#10464=ORIENTED_EDGE ( 'NONE', *, *, #17147, .T. ) ;
#10466=LINE ( 'NONE', #3909, #7978 ) ;
#10468=ORIENTED_EDGE ( 'NONE', *, *, #6942, .F. ) ;
#10469=ORIENTED_EDGE ( 'NONE', *, *, #1517, .T. ) ;
#10470=CARTESIAN_POINT ( 'NONE',  ( 216.3355731942785951, 15.66405044361498788, -16.89203719259520753 ) ) ;
#10471=VECTOR ( 'NONE', #2515, 1000.000000000000000 ) ;
#10476=EDGE_LOOP ( 'NONE', ( #17122, #19446, #19658, #12761 ) ) ;
#10479=DIRECTION ( 'NONE',  ( -0.8660254037843260200, -0.5000000000001951772, 0.000000000000000000 ) ) ;
#10482=AXIS2_PLACEMENT_3D ( 'NONE', #1956, #5015, #17964 ) ;
#10483=DIRECTION ( 'NONE',  ( -0.05035489893517522408, -0.02907241445524020446, -0.9983081582712679536 ) ) ;
#10497=VERTEX_POINT ( 'NONE', #2840 ) ;
#10502=AXIS2_PLACEMENT_3D ( 'NONE', #3907, #18439, #16848 ) ;
#10503=ORIENTED_EDGE ( 'NONE', *, *, #5108, .T. ) ;
#10505=DIRECTION ( 'NONE',  ( 0.1503837331804316335, 0.08682408883346437456, -0.9848077530122086864 ) ) ;
#10514=CARTESIAN_POINT ( 'NONE',  ( 197.5418782473972499, 4.813505606965178707, -5.993340328401664863 ) ) ;
#10519=ADVANCED_FACE ( 'NONE', ( #10347 ), #6205, .T. ) ;
#10520=ORIENTED_EDGE ( 'NONE', *, *, #11081, .T. ) ;
#10524=LINE ( 'NONE', #2490, #14295 ) ;
#10526=CARTESIAN_POINT ( 'NONE',  ( 199.0943133668587564, -1.182153763511707867, -18.09983247376283089 ) ) ;
#10527=ORIENTED_EDGE ( 'NONE', *, *, #12948, .F. ) ;
#10528=CIRCLE ( 'NONE', #14968, 11.98469917212512215 ) ;
#10529=CARTESIAN_POINT ( 'NONE',  ( 215.1214136286681082, 19.61810227076572843, -12.41782726985285557 ) ) ;
#10532=ORIENTED_EDGE ( 'NONE', *, *, #16178, .F. ) ;
#10534=EDGE_CURVE ( 'NONE', #1000, #17941, #1149, .T. ) ;
#10537=ORIENTED_EDGE ( 'NONE', *, *, #13316, .F. ) ;
#10538=CYLINDRICAL_SURFACE ( 'NONE', #14276, 12.47473710546057646 ) ;
#10541=CYLINDRICAL_SURFACE ( 'NONE', #1016, 12.47473710546057646 ) ;
#10544=DIRECTION ( 'NONE',  ( 0.5171545105027588463, 0.2985792958514013051, 0.8021231927550364071 ) ) ;
#10545=VERTEX_POINT ( 'NONE', #10663 ) ;
#10547=AXIS2_PLACEMENT_3D ( 'NONE', #5710, #19929, #648 ) ;
#10549=VECTOR ( 'NONE', #8077, 1000.000000000000000 ) ;
#10551=EDGE_CURVE ( 'NONE', #3195, #18441, #271, .T. ) ;
#10555=ORIENTED_EDGE ( 'NONE', *, *, #18145, .T. ) ;
#10563=CARTESIAN_POINT ( 'NONE',  ( 204.9818247258934321, 9.640009970873842704, -2.036337243043272238 ) ) ;
#10570=FACE_OUTER_BOUND ( 'NONE', #17617, .T. ) ;
#10580=CARTESIAN_POINT ( 'NONE',  ( 218.9914638623158396, 11.07829152179047760, -11.13829696442610029 ) ) ;
#10582=DIRECTION ( 'NONE',  ( 0.8679903670753312817, 0.4965810333313504521, 0.000000000000000000 ) ) ;
#10583=EDGE_CURVE ( 'NONE', #18856, #9864, #9869, .T. ) ;
#10585=ORIENTED_EDGE ( 'NONE', *, *, #10314, .F. ) ;
#10588=DIRECTION ( 'NONE',  ( -0.8660254037844355990, -0.5000000000000055511, 0.000000000000000000 ) ) ;
#10595=FACE_OUTER_BOUND ( 'NONE', #7536, .T. ) ;
#10597=AXIS2_PLACEMENT_3D ( 'NONE', #19557, #5035, #11511 ) ;
#10598=CARTESIAN_POINT ( 'NONE',  ( 199.1738290307970374, -1.136245373532171588, -9.972943347741736630 ) ) ;
#10600=DIRECTION ( 'NONE',  ( -0.05035489893516262305, -0.02907241445523293250, 0.9983081582712687307 ) ) ;
#10605=DIRECTION ( 'NONE',  ( -0.8660254037844357100, -0.5000000000000051070, 0.000000000000000000 ) ) ;
#10609=CIRCLE ( 'NONE', #1158, 12.47473710546057823 ) ;
#10618=ADVANCED_FACE ( 'NONE', ( #1767 ), #6486, .T. ) ;
#10634=CARTESIAN_POINT ( 'NONE',  ( 205.5965122587965084, 9.994899983462953941, -14.00000000000005507 ) ) ;
#10636=CARTESIAN_POINT ( 'NONE',  ( 198.0735972701637024, -1.389238810292188875, -14.00000000000005507 ) ) ;
#10646=ORIENTED_EDGE ( 'NONE', *, *, #1906, .F. ) ;
#10652=CARTESIAN_POINT ( 'NONE',  ( 200.4167038695724443, 7.004336215593725434, -24.38552490958304020 ) ) ;
#10658=ORIENTED_EDGE ( 'NONE', *, *, #11302, .F. ) ;
#10663=CARTESIAN_POINT ( 'NONE',  ( 210.1178786253386193, 12.07426281049857408, -2.551678190571530891 ) ) ;
#10669=ORIENTED_EDGE ( 'NONE', *, *, #7428, .F. ) ;
#10672=CARTESIAN_POINT ( 'NONE',  ( 208.6933310212059496, 11.60583922538805268, -2.363289276295987840 ) ) ;
#10676=EDGE_CURVE ( 'NONE', #16137, #13251, #13213, .T. ) ;
#10677=FACE_OUTER_BOUND ( 'NONE', #10476, .T. ) ;
#10678=CARTESIAN_POINT ( 'NONE',  ( 205.8264633344831225, 9.596613037118636669, -14.00000000000005507 ) ) ;
#10682=ORIENTED_EDGE ( 'NONE', *, *, #20645, .F. ) ;
#10684=VERTEX_POINT ( 'NONE', #17987 ) ;
#10687=EDGE_CURVE ( 'NONE', #13380, #7589, #13011, .T. ) ;
#10688=DIRECTION ( 'NONE',  ( 0.5000000000000054401, -0.8660254037844354880, 2.220446049250312834E-16 ) ) ;
#10690=FACE_OUTER_BOUND ( 'NONE', #6889, .T. ) ;
#10691=ADVANCED_FACE ( 'NONE', ( #3453 ), #5136, .F. ) ;
#10692=ORIENTED_EDGE ( 'NONE', *, *, #4187, .T. ) ;
#10700=LINE ( 'NONE', #10804, #10970 ) ;
#10703=ORIENTED_EDGE ( 'NONE', *, *, #16178, .T. ) ;
#10707=ORIENTED_EDGE ( 'NONE', *, *, #10182, .F. ) ;
#10710=CARTESIAN_POINT ( 'NONE',  ( 208.8107687779841228, 4.427644383670616079, -14.00000000000005507 ) ) ;
#10719=CARTESIAN_POINT ( 'NONE',  ( 201.0721825858487364, 0.7325896531374328502, -4.915515517929136990 ) ) ;
#10723=EDGE_CURVE ( 'NONE', #12475, #15862, #18224, .T. ) ;
#10726=FACE_OUTER_BOUND ( 'NONE', #13680, .T. ) ;
#10734=ORIENTED_EDGE ( 'NONE', *, *, #15653, .F. ) ;
#10736=CARTESIAN_POINT ( 'NONE',  ( 200.8894739819445192, 11.40128808463920329, -25.34310559273323804 ) ) ;
#10737=EDGE_LOOP ( 'NONE', ( #17425, #11777, #7449, #6247 ) ) ;
#10738=DIRECTION ( 'NONE',  ( -0.5000000000000051070, 0.8660254037844359321, -0.000000000000000000 ) ) ;
#10741=DIRECTION ( 'NONE',  ( 0.1005394128318207458, 0.05804645706261939847, 0.9932383577419421350 ) ) ;
#10742=ORIENTED_EDGE ( 'NONE', *, *, #4409, .T. ) ;
#10747=ORIENTED_EDGE ( 'NONE', *, *, #17793, .F. ) ;
#10749=CARTESIAN_POINT ( 'NONE',  ( 199.8291677591948314, 21.40379373188257972, -1.545471579934816875 ) ) ;
#10757=ORIENTED_EDGE ( 'NONE', *, *, #19628, .F. ) ;
#10758=VERTEX_POINT ( 'NONE', #20204 ) ;
#10761=LINE ( 'NONE', #8964, #3423 ) ;
#10766=CARTESIAN_POINT ( 'NONE',  ( 209.3909370991932519, 3.422763374394458769, -14.00000000000005507 ) ) ;
#10767=ORIENTED_EDGE ( 'NONE', *, *, #7183, .T. ) ;
#10774=DIRECTION ( 'NONE',  ( -0.5000000000000049960, 0.8660254037844358210, -0.000000000000000000 ) ) ;
#10780=CARTESIAN_POINT ( 'NONE',  ( 196.0270608673617687, 8.593972564023673044, -4.392917125964746816 ) ) ;
#10781=LINE ( 'NONE', #4330, #13245 ) ;
#10782=( NAMED_UNIT ( * ) PLANE_ANGLE_UNIT ( ) SI_UNIT ( $, .RADIAN. ) );
#10788=FACE_OUTER_BOUND ( 'NONE', #9013, .T. ) ;
#10789=ORIENTED_EDGE ( 'NONE', *, *, #18858, .T. ) ;
#10793=EDGE_CURVE ( 'NONE', #4941, #16061, #13983, .T. ) ;
#10796=DIRECTION ( 'NONE',  ( -0.4330127018922105275, -0.2499999999999986955, 0.8660254037844433705 ) ) ;
#10797=PLANE ( 'NONE',  #7565 ) ;
#10798=CARTESIAN_POINT ( 'NONE',  ( 214.7634125556922129, 15.28741233751021156, -19.29168348739315775 ) ) ;
#10800=DIRECTION ( 'NONE',  ( -0.8660254037844357100, -0.5000000000000049960, 0.000000000000000000 ) ) ;
#10801=CARTESIAN_POINT ( 'NONE',  ( 197.6726970570908293, -1.230104231997219300, -14.01558723443171850 ) ) ;
#10804=CARTESIAN_POINT ( 'NONE',  ( 205.6766695652311512, 24.77985047368454019, -4.003039906354141308 ) ) ;
#10809=EDGE_CURVE ( 'NONE', #6449, #14979, #18935, .T. ) ;
#10813=DIRECTION ( 'NONE',  ( -0.8660254037844354880, -0.5000000000000055511, 0.000000000000000000 ) ) ;
#10818=VERTEX_POINT ( 'NONE', #9168 ) ;
#10821=CARTESIAN_POINT ( 'NONE',  ( 204.3420759002525529, 1.847643347786420698, -26.10173121575770594 ) ) ;
#10824=EDGE_CURVE ( 'NONE', #7471, #7703, #6087, .T. ) ;
#10825=CIRCLE ( 'NONE', #5069, 11.94520687646042667 ) ;
#10826=EDGE_CURVE ( 'NONE', #15665, #7763, #14340, .T. ) ;
#10827=CARTESIAN_POINT ( 'NONE',  ( 219.2080768649571496, 11.20335309717537520, -15.43274561385901400 ) ) ;
#10828=CARTESIAN_POINT ( 'NONE',  ( 215.9040783327276358, 15.94597603093701466, -15.40420431385954281 ) ) ;
#10835=CARTESIAN_POINT ( 'NONE',  ( 188.4825312237924777, 14.85281007377110640, -15.43274561385865695 ) ) ;
#10836=VECTOR ( 'NONE', #9953, 1000.000000000000114 ) ;
#10840=CIRCLE ( 'NONE', #12886, 11.98469917212512215 ) ;
#10841=CARTESIAN_POINT ( 'NONE',  ( 213.9878548032869503, 18.96364177778961491, -15.39542905462748656 ) ) ;
#10848=DIRECTION ( 'NONE',  ( -0.9795788631971408256, 0.000000000000000000, -0.2010603162670278610 ) ) ;
#10849=CIRCLE ( 'NONE', #11422, 11.98469917212512215 ) ;
#10852=CARTESIAN_POINT ( 'NONE',  ( 214.9988779556950078, 8.000350883196837515, -23.57241037536588735 ) ) ;
#10856=ORIENTED_EDGE ( 'NONE', *, *, #10676, .T. ) ;
#10857=CARTESIAN_POINT ( 'NONE',  ( 208.9119903699346708, 11.37804290162847209, -2.044871543907030631 ) ) ;
#10863=B_SPLINE_CURVE_WITH_KNOTS ( 'NONE', 3,
 ( #17436, #7455, #13950, #20492 ),
 .UNSPECIFIED., .F., .F.,
 ( 4, 4 ),
 ( 6.919709117646055681E-07, 0.0006733427629651237561 ),
 .UNSPECIFIED. ) ;
#10872=VECTOR ( 'NONE', #4375, 1000.000000000000114 ) ;
#10875=DIRECTION ( 'NONE',  ( -0.5000000000000054401, 0.8660254037844354880, -0.000000000000000000 ) ) ;
#10879=DIRECTION ( 'NONE',  ( 0.5000000000000051070, -0.8660254037844359321, 0.000000000000000000 ) ) ;
#10884=VECTOR ( 'NONE', #446, 1000.000000000000114 ) ;
#10885=CONICAL_SURFACE ( 'NONE', #3775, 13.07248899748297433, 0.6693469023067423196 ) ;
#10888=DIRECTION ( 'NONE',  ( -0.5000000000000049960, 0.8660254037844358210, -0.000000000000000000 ) ) ;
#10889=ADVANCED_FACE ( 'NONE', ( #7787 ), #14292, .F. ) ;
#10890=ORIENTED_EDGE ( 'NONE', *, *, #18317, .T. ) ;
#10892=CARTESIAN_POINT ( 'NONE',  ( 207.0274154277438754, 3.398024846849156511, -2.233628351993186101 ) ) ;
#10893=FACE_OUTER_BOUND ( 'NONE', #1423, .T. ) ;
#10894=DIRECTION ( 'NONE',  ( 0.5000000000000052180, -0.8660254037844355990, 1.665334536937734564E-16 ) ) ;
#10895=VERTEX_POINT ( 'NONE', #7477 ) ;
#10897=ORIENTED_EDGE ( 'NONE', *, *, #13306, .F. ) ;
#10905=CARTESIAN_POINT ( 'NONE',  ( 206.9147384664715901, 10.75597823931698294, -11.08174281168198227 ) ) ;
#10910=DIRECTION ( 'NONE',  ( 0.5171545105027589573, 0.2985792958514010831, 0.8021231927550364071 ) ) ;
#10911=EDGE_CURVE ( 'NONE', #8365, #17033, #15683, .T. ) ;
#10912=AXIS2_PLACEMENT_3D ( 'NONE', #13451, #19899, #13347 ) ;
#10916=CARTESIAN_POINT ( 'NONE',  ( 207.4656388362384973, 11.07404071609857077, -17.01204567730803063 ) ) ;
#10917=DIRECTION ( 'NONE',  ( 0.8660254037844355990, 0.5000000000000054401, 5.284238980736809733E-15 ) ) ;
#10919=ADVANCED_FACE ( 'NONE', ( #7366 ), #7527, .F. ) ;
#10920=VERTEX_POINT ( 'NONE', #4203 ) ;
#10922=CARTESIAN_POINT ( 'NONE',  ( 202.0139385235187035, 1.276312697262135920, -4.003039906353937916 ) ) ;
#10925=ORIENTED_EDGE ( 'NONE', *, *, #10430, .F. ) ;
#10927=AXIS2_PLACEMENT_3D ( 'NONE', #17667, #5020, #19439 ) ;
#10929=B_SPLINE_CURVE_WITH_KNOTS ( 'NONE', 3,
 ( #4923, #4721, #3235, #17767 ),
 .UNSPECIFIED., .F., .F.,
 ( 4, 4 ),
 ( 3.242053695154241001E-07, 0.0008543099433544477624 ),
 .UNSPECIFIED. ) ;
#10932=CARTESIAN_POINT ( 'NONE',  ( 219.0871984830704662, 10.36074384021052985, -12.62839849932177394 ) ) ;
#10935=ORIENTED_EDGE ( 'NONE', *, *, #7040, .T. ) ;
#10938=DIRECTION ( 'NONE',  ( 0.5000000000000054401, -0.8660254037844354880, -2.220446049250312834E-16 ) ) ;
#10940=CARTESIAN_POINT ( 'NONE',  ( 199.2144802262915846, 21.04890371929339921, -14.00000000000005507 ) ) ;
#10941=CARTESIAN_POINT ( 'NONE',  ( 208.8577037357181894, 4.346350652224124644, -14.00000000000005507 ) ) ;
#10944=LINE ( 'NONE', #9124, #19687 ) ;
#10945=ADVANCED_FACE ( 'NONE', ( #11609 ), #11295, .F. ) ;
#10947=CARTESIAN_POINT ( 'NONE',  ( 206.2937561296588456, 1.095629421411969950, -14.00000000000005507 ) ) ;
#10949=EDGE_LOOP ( 'NONE', ( #17950, #5351, #4306, #3355 ) ) ;
#10951=EDGE_CURVE ( 'NONE', #11581, #6296, #103, .T. ) ;
#10953=EDGE_CURVE ( 'NONE', #4965, #17368, #1788, .T. ) ;
#10955=CARTESIAN_POINT ( 'NONE',  ( 199.2144802262915846, 21.04890371929339921, -14.00000000000005507 ) ) ;
#10963=ORIENTED_EDGE ( 'NONE', *, *, #20937, .T. ) ;
#10966=CARTESIAN_POINT ( 'NONE',  ( 205.5965122587965084, 9.994899983462953941, -14.00000000000005507 ) ) ;
#10967=EDGE_CURVE ( 'NONE', #6104, #15417, #11947, .T. ) ;
#10969=VECTOR ( 'NONE', #7422, 1000.000000000000114 ) ;
#10970=VECTOR ( 'NONE', #4249, 1000.000000000000227 ) ;
#10972=ORIENTED_EDGE ( 'NONE', *, *, #10967, .F. ) ;
#10973=CARTESIAN_POINT ( 'NONE',  ( 208.8107687779841228, 4.427644383670616079, -14.00000000000005507 ) ) ;
#10978=CARTESIAN_POINT ( 'NONE',  ( 214.9514471701782270, 8.488172945287894677, -4.138477629886256004 ) ) ;
#10981=ADVANCED_FACE ( 'NONE', ( #1548 ), #9841, .T. ) ;
#10984=EDGE_CURVE ( 'NONE', #14638, #14727, #14809, .T. ) ;
#10987=CARTESIAN_POINT ( 'NONE',  ( 204.6045052031513478, 24.16083609062223303, -3.188775577416895324 ) ) ;
#10988=AXIS2_PLACEMENT_3D ( 'NONE', #70, #9989, #5130 ) ;
#10989=DIRECTION ( 'NONE',  ( 0.8660254037844355990, 0.5000000000000054401, 0.000000000000000000 ) ) ;
#10992=ORIENTED_EDGE ( 'NONE', *, *, #18100, .T. ) ;
#10993=DIRECTION ( 'NONE',  ( -0.9170191824714420958, 0.000000000000000000, -0.3988431007042845255 ) ) ;
#10999=CIRCLE ( 'NONE', #18783, 11.98469917212512215 ) ;
#11003=ORIENTED_EDGE ( 'NONE', *, *, #4847, .F. ) ;
#11005=CARTESIAN_POINT ( 'NONE',  ( 218.8798129321970976, 10.24100973658777924, -16.73990883341947367 ) ) ;
#11008=EDGE_LOOP ( 'NONE', ( #13575, #10469, #9529, #12250 ) ) ;
#11015=ORIENTED_EDGE ( 'NONE', *, *, #2917, .F. ) ;
#11019=ADVANCED_FACE ( 'NONE', ( #15336 ), #16797, .F. ) ;
#11020=VECTOR ( 'NONE', #2134, 1000.000000000000000 ) ;
#11030=AXIS2_PLACEMENT_3D ( 'NONE', #3888, #2411, #8867 ) ;
#11032=EDGE_CURVE ( 'NONE', #3882, #5656, #3540, .T. ) ;
#11041=CARTESIAN_POINT ( 'NONE',  ( 211.5616548979095626, 6.788689316162965781, -2.044871543907030631 ) ) ;
#11042=EDGE_CURVE ( 'NONE', #2725, #9686, #3135, .T. ) ;
#11048=ORIENTED_EDGE ( 'NONE', *, *, #10583, .F. ) ;
#11049=DIRECTION ( 'NONE',  ( 0.5000000000000057732, -0.8660254037844352659, 4.857225732735059864E-17 ) ) ;
#11062=ORIENTED_EDGE ( 'NONE', *, *, #13309, .F. ) ;
#11068=EDGE_CURVE ( 'NONE', #6425, #2244, #17998, .T. ) ;
#11069=DIRECTION ( 'NONE',  ( 0.5000000000000051070, -0.8660254037844359321, 0.000000000000000000 ) ) ;
#11074=DIRECTION ( 'NONE',  ( -0.9679941405060923376, 0.000000000000000000, -0.2509727952306220478 ) ) ;
#11078=CARTESIAN_POINT ( 'NONE',  ( 216.3417993343409194, 15.66764510725598214, -11.13829696442610029 ) ) ;
#11081=EDGE_CURVE ( 'NONE', #3522, #2297, #375, .T. ) ;
#11083=ORIENTED_EDGE ( 'NONE', *, *, #13309, .T. ) ;
#11086=DIRECTION ( 'NONE',  ( 0.5000000000000049960, -0.8660254037844358210, 0.000000000000000000 ) ) ;
#11092=CARTESIAN_POINT ( 'NONE',  ( 212.1124805811015790, 13.40286946702044979, -23.87887634647646351 ) ) ;
#11098=CARTESIAN_POINT ( 'NONE',  ( 208.0983737146324870, 5.661548828456886895, -14.00000000000005507 ) ) ;
#11099=LINE ( 'NONE', #20428, #6080 ) ;
#11103=ORIENTED_EDGE ( 'NONE', *, *, #10723, .F. ) ;
#11104=PLANE ( 'NONE',  #19323 ) ;
#11106=ADVANCED_FACE ( 'NONE', ( #13408 ), #10202, .F. ) ;
#11108=( LENGTH_UNIT ( ) NAMED_UNIT ( * ) SI_UNIT ( .MILLI., .METRE. ) );
#11109=ORIENTED_EDGE ( 'NONE', *, *, #16314, .F. ) ;
#11116=ORIENTED_EDGE ( 'NONE', *, *, #14172, .F. ) ;
#11120=STYLED_ITEM('',(#20988),#17843);
#11133=ORIENTED_EDGE ( 'NONE', *, *, #2373, .T. ) ;
#11135=EDGE_LOOP ( 'NONE', ( #4407, #2066, #17167, #17497 ) ) ;
#11137=DIRECTION ( 'NONE',  ( -0.8660254037844358210, -0.5000000000000049960, 0.000000000000000000 ) ) ;
#11138=ORIENTED_EDGE ( 'NONE', *, *, #12783, .F. ) ;
#11140=CARTESIAN_POINT ( 'NONE',  ( 209.8428577672754898, 12.26951880167198894, -25.15316579317395096 ) ) ;
#11141=EDGE_LOOP ( 'NONE', ( #11256, #3904, #2947, #17104 ) ) ;
#11143=CARTESIAN_POINT ( 'NONE',  ( 202.6226596002730389, 0.8549378841442712984, -23.57241037536569195 ) ) ;
#11145=DIRECTION ( 'NONE',  ( -0.5000000000000049960, 0.8660254037844357100, -0.000000000000000000 ) ) ;
#11148=DIRECTION ( 'NONE',  ( 0.5000000000000049960, -0.8660254037844357100, 0.000000000000000000 ) ) ;
#11151=DIRECTION ( 'NONE',  ( -0.8660254037844355990, -0.5000000000000051070, 0.000000000000000000 ) ) ;
#11152=CARTESIAN_POINT ( 'NONE',  ( 202.6868825351897669, 7.960997897939990686, -25.79243801023027061 ) ) ;
#11154=CARTESIAN_POINT ( 'NONE',  ( 205.5965122587965084, 9.994899983462953941, -14.00000000000005507 ) ) ;
#11162=ORIENTED_EDGE ( 'NONE', *, *, #1306, .T. ) ;
#11166=DIRECTION ( 'NONE',  ( -0.5000000000000049960, 0.8660254037844358210, 0.000000000000000000 ) ) ;
#11167=VERTEX_POINT ( 'NONE', #15124 ) ;
#11168=DIRECTION ( 'NONE',  ( -0.8660254037844357100, -0.5000000000000051070, 0.000000000000000000 ) ) ;
#11172=VERTEX_POINT ( 'NONE', #7031 ) ;
#11175=DIRECTION ( 'NONE',  ( 0.8660254037844355990, 0.5000000000000054401, 0.000000000000000000 ) ) ;
#11176=ORIENTED_EDGE ( 'NONE', *, *, #7965, .T. ) ;
#11180=CARTESIAN_POINT ( 'NONE',  ( 205.5965122587965084, 9.994899983462953941, -14.00000000000005507 ) ) ;
#11184=EDGE_CURVE ( 'NONE', #19244, #5690, #1317, .T. ) ;
#11190=LINE ( 'NONE', #11297, #13778 ) ;
#11198=CARTESIAN_POINT ( 'NONE',  ( 211.9579643972498673, 13.49067618385247158, -23.74217242726248145 ) ) ;
#11200=CONICAL_SURFACE ( 'NONE', #6430, 13.07248899748297433, 0.6693469023067423196 ) ;
#11202=DIRECTION ( 'NONE',  ( 0.05035489893517486326, 0.02907241445524025303, 0.9983081582712680646 ) ) ;
#11204=PLANE ( 'NONE',  #7220 ) ;
#11205=AXIS2_PLACEMENT_3D ( 'NONE', #12146, #10215, #8420 ) ;
#11207=LINE ( 'NONE', #8215, #3708 ) ;
#11209=CARTESIAN_POINT ( 'NONE',  ( 205.5965122587965084, 9.994899983462952164, -14.00000000000005507 ) ) ;
#11210=VERTEX_POINT ( 'NONE', #9349 ) ;
#11216=VECTOR ( 'NONE', #13303, 1000.000000000000227 ) ;
#11220=LINE ( 'NONE', #14735, #8497 ) ;
#11223=DIRECTION ( 'NONE',  ( -0.8660254037844355990, -0.5000000000000055511, 0.000000000000000000 ) ) ;
#11225=ADVANCED_FACE ( 'NONE', ( #9244 ), #19350, .T. ) ;
#11230=AXIS2_PLACEMENT_3D ( 'NONE', #6824, #581, #13409 ) ;
#11233=CIRCLE ( 'NONE', #4791, 11.98469917212512215 ) ;
#11243=CARTESIAN_POINT ( 'NONE',  ( 197.6756539743620351, 9.545788238134468529, -23.47937149798923073 ) ) ;
#11248=VERTEX_POINT ( 'NONE', #18595 ) ;
#11252=CIRCLE ( 'NONE', #2109, 6.960520131757800932 ) ;
#11253=EDGE_CURVE ( 'NONE', #15055, #2247, #10524, .T. ) ;
#11256=ORIENTED_EDGE ( 'NONE', *, *, #18704, .T. ) ;
#11258=LINE ( 'NONE', #7951, #6049 ) ;
#11260=CARTESIAN_POINT ( 'NONE',  ( 199.2144802262915846, 21.04890371929339921, -14.00000000000005507 ) ) ;
#11263=CARTESIAN_POINT ( 'NONE',  ( 198.6701878702990030, 10.11998265067189529, -3.762296834228767484 ) ) ;
#11272=CARTESIAN_POINT ( 'NONE',  ( 205.5889925535339557, 2.567551013215509936, -1.381056684022587078 ) ) ;
#11274=ORIENTED_EDGE ( 'NONE', *, *, #15439, .T. ) ;
#11277=LINE ( 'NONE', #15954, #18352 ) ;
#11278=ORIENTED_EDGE ( 'NONE', *, *, #7177, .T. ) ;
#11282=DIRECTION ( 'NONE',  ( -0.8660254037844355990, -0.5000000000000054401, -1.599177586275613688E-14 ) ) ;
#11283=ADVANCED_FACE ( 'NONE', ( #12951 ), #10885, .T. ) ;
#11292=DIRECTION ( 'NONE',  ( 0.5000000000000057732, -0.8660254037844352659, -4.857225732735059248E-17 ) ) ;
#11293=ADVANCED_FACE ( 'NONE', ( #10677 ), #6145, .T. ) ;
#11295=PLANE ( 'NONE',  #10927 ) ;
#11296=DIRECTION ( 'NONE',  ( 0.5000000000000051070, -0.8660254037844359321, 0.000000000000000000 ) ) ;
#11297=CARTESIAN_POINT ( 'NONE',  ( 198.5728404875461024, 20.67845284340592471, -26.45271578590682893 ) ) ;
#11298=CARTESIAN_POINT ( 'NONE',  ( 205.0662616026534693, 10.91332106064940888, -14.00000000000005507 ) ) ;
#11302=EDGE_CURVE ( 'NONE', #12664, #14889, #17175, .T. ) ;
#11305=DIRECTION ( 'NONE',  ( -0.8296432542242785368, -0.4789947561577507784, -0.2868032327110803803 ) ) ;
#11306=VERTEX_POINT ( 'NONE', #4230 ) ;
#11309=DIRECTION ( 'NONE',  ( 1.000000000000000000, 0.000000000000000000, 0.000000000000000000 ) ) ;
#11310=PLANE ( 'NONE',  #12185 ) ;
#11312=B_SPLINE_CURVE_WITH_KNOTS ( 'NONE', 3,
 ( #2237, #20141, #11885, #18348 ),
 .UNSPECIFIED., .F., .F.,
 ( 4, 4 ),
 ( 3.625823136733547116E-05, 0.0008902439693512922492 ),
 .UNSPECIFIED. ) ;
#11314=VERTEX_POINT ( 'NONE', #1163 ) ;
#11315=VERTEX_POINT ( 'NONE', #19171 ) ;
#11316=CARTESIAN_POINT ( 'NONE',  ( 218.5653220041813540, 10.31703753844722016, -9.858802615641375056 ) ) ;
#11317=CARTESIAN_POINT ( 'NONE',  ( 208.4761278624580711, 5.007259451653140125, -14.00000000000005507 ) ) ;
#11323=CARTESIAN_POINT ( 'NONE',  ( 215.8450800869675277, 15.91191337786571403, -13.97827067520052147 ) ) ;
#11325=CARTESIAN_POINT ( 'NONE',  ( 198.0882619218635057, -1.762997836098331828, -18.44761907388178912 ) ) ;
#11328=CARTESIAN_POINT ( 'NONE',  ( 196.1030895030431225, 19.25254144767176356, -25.94618751764486575 ) ) ;
#11329=EDGE_CURVE ( 'NONE', #15290, #7006, #15697, .T. ) ;
#11331=AXIS2_PLACEMENT_3D ( 'NONE', #777, #8394, #14897 ) ;
#11332=DIRECTION ( 'NONE',  ( 0.5000000000000057732, -0.8660254037844352659, 0.000000000000000000 ) ) ;
#11336=DIRECTION ( 'NONE',  ( 0.7235536692358585098, 0.4177439057064706307, -0.5495089780708131144 ) ) ;
#11339=ORIENTED_EDGE ( 'NONE', *, *, #14494, .F. ) ;
#11345=DIRECTION ( 'NONE',  ( -0.8660254037844354880, -0.5000000000000055511, 0.000000000000000000 ) ) ;
#11355=CYLINDRICAL_SURFACE ( 'NONE', #1550, 12.47473710546057646 ) ;
#11359=DIRECTION ( 'NONE',  ( -0.5171545105027588463, -0.2985792958514009166, -0.8021231927550366292 ) ) ;
#11364=ORIENTED_EDGE ( 'NONE', *, *, #15264, .T. ) ;
#11365=VECTOR ( 'NONE', #8158, 1000.000000000000000 ) ;
#11375=EDGE_LOOP ( 'NONE', ( #9990, #5466, #6914, #18804 ) ) ;
#11377=ORIENTED_EDGE ( 'NONE', *, *, #5380, .T. ) ;
#11381=EDGE_CURVE ( 'NONE', #184, #18641, #12499, .T. ) ;
#11382=CARTESIAN_POINT ( 'NONE',  ( 200.1750369523376492, -0.5581977105158604235, -20.57673792763505460 ) ) ;
#11391=AXIS2_PLACEMENT_3D ( 'NONE', #2103, #2306, #10232 ) ;
#11395=VERTEX_POINT ( 'NONE', #4438 ) ;
#11396=CARTESIAN_POINT ( 'NONE',  ( 200.6547414633283211, -0.02364095815690154048, -21.78787861992495323 ) ) ;
#11403=AXIS2_PLACEMENT_3D ( 'NONE', #2177, #19758, #8629 ) ;
#11406=ORIENTED_EDGE ( 'NONE', *, *, #10723, .T. ) ;
#11407=B_SPLINE_CURVE_WITH_KNOTS ( 'NONE', 3,
 ( #13414, #3968, #19860, #5326 ),
 .UNSPECIFIED., .F., .F.,
 ( 4, 4 ),
 ( 3.702528811464445919E-05, 0.0007096760801717362337 ),
 .UNSPECIFIED. ) ;
#11413=ORIENTED_EDGE ( 'NONE', *, *, #14357, .T. ) ;
#11416=CARTESIAN_POINT ( 'NONE',  ( 196.3164214246273218, 4.637037042251114904, -19.36714384557513924 ) ) ;
#11422=AXIS2_PLACEMENT_3D ( 'NONE', #2029, #14984, #4029 ) ;
#11423=CARTESIAN_POINT ( 'NONE',  ( 214.2742449478047604, 15.00499128741754262, -7.425127016398544555 ) ) ;
#11428=ORIENTED_EDGE ( 'NONE', *, *, #5679, .T. ) ;
#11430=CARTESIAN_POINT ( 'NONE',  ( 215.6692934924029146, 15.81042294017388805, -11.13964600021398432 ) ) ;
#11431=B_SPLINE_CURVE_WITH_KNOTS ( 'NONE', 3,
 ( #7933, #3656, #6338, #5339 ),
 .UNSPECIFIED., .F., .F.,
 ( 4, 4 ),
 ( 9.556227015513408202E-07, 0.0006736064147546274401 ),
 .UNSPECIFIED. ) ;
#11433=VECTOR ( 'NONE', #1733, 1000.000000000000114 ) ;
#11434=DIRECTION ( 'NONE',  ( -0.8660254037844373753, -0.5000000000000022204, 0.000000000000000000 ) ) ;
#11438=AXIS2_PLACEMENT_3D ( 'NONE', #15705, #7299, #10588 ) ;
#11446=CARTESIAN_POINT ( 'NONE',  ( 210.3654177961080052, 6.098041503423209164, -1.717498466822859227 ) ) ;
#11454=EDGE_CURVE ( 'NONE', #20019, #15072, #12301, .T. ) ;
#11456=DIRECTION ( 'NONE',  ( -0.8660254037844355990, -0.5000000000000055511, 0.000000000000000000 ) ) ;
#11458=DIRECTION ( 'NONE',  ( 0.8660254037844355990, 0.5000000000000054401, 0.000000000000000000 ) ) ;
#11465=ORIENTED_EDGE ( 'NONE', *, *, #7456, .F. ) ;
#11466=FACE_OUTER_BOUND ( 'NONE', #928, .T. ) ;
#11469=CARTESIAN_POINT ( 'NONE',  ( 206.6134256523022259, 3.931827829199530999, -26.28791492288515386 ) ) ;
#11476=B_SPLINE_CURVE_WITH_KNOTS ( 'NONE', 3,
 ( #9613, #1991, #291, #9816 ),
 .UNSPECIFIED., .F., .F.,
 ( 4, 4 ),
 ( 4.589663077585729394E-07, 0.0006731097583523744637 ),
 .UNSPECIFIED. ) ;
#11480=VECTOR ( 'NONE', #11751, 1000.000000000000114 ) ;
#11481=ORIENTED_EDGE ( 'NONE', *, *, #467, .F. ) ;
#11482=LINE ( 'NONE', #20906, #5210 ) ;
#11486=DIRECTION ( 'NONE',  ( 0.8660254037844355990, 0.5000000000000054401, 0.000000000000000000 ) ) ;
#11487=EDGE_LOOP ( 'NONE', ( #1888, #5714, #1338, #15158 ) ) ;
#11489=CARTESIAN_POINT ( 'NONE',  ( 214.8451803045405484, 14.80357170752643370, -7.132002368301448847 ) ) ;
#11491=ORIENTED_EDGE ( 'NONE', *, *, #15516, .F. ) ;
#11493=EDGE_CURVE ( 'NONE', #330, #2960, #11233, .T. ) ;
#11501=CARTESIAN_POINT ( 'NONE',  ( 200.8776667170992027, -0.1525342266901607846, -21.66653917424381603 ) ) ;
#11507=VECTOR ( 'NONE', #19453, 1000.000000000000114 ) ;
#11508=ORIENTED_EDGE ( 'NONE', *, *, #343, .F. ) ;
#11511=DIRECTION ( 'NONE',  ( 0.8660254037844355990, 0.5000000000000054401, 0.000000000000000000 ) ) ;
#11513=FACE_OUTER_BOUND ( 'NONE', #3561, .T. ) ;
#11518=ORIENTED_EDGE ( 'NONE', *, *, #10376, .T. ) ;
#11520=CARTESIAN_POINT ( 'NONE',  ( 208.8107687779841228, 4.427644383670616079, -14.00000000000005507 ) ) ;
#11524=LINE ( 'NONE', #17693, #20336 ) ;
#11525=DIRECTION ( 'NONE',  ( 0.5000000000000054401, -0.8660254037844354880, 0.000000000000000000 ) ) ;
#11528=ORIENTED_EDGE ( 'NONE', *, *, #1647, .F. ) ;
#11529=AXIS2_PLACEMENT_3D ( 'NONE', #20587, #2593, #17318 ) ;
#11533=B_SPLINE_CURVE_WITH_KNOTS ( 'NONE', 3,
 ( #4374, #19008, #987, #16813 ),
 .UNSPECIFIED., .F., .F.,
 ( 4, 4 ),
 ( 5.642010595650565963E-05, 0.0009104058439395384603 ),
 .UNSPECIFIED. ) ;
#11534=LINE ( 'NONE', #13449, #19590 ) ;
#11541=CARTESIAN_POINT ( 'NONE',  ( 208.8107687779841228, 4.427644383670616079, -14.00000000000005507 ) ) ;
#11546=CIRCLE ( 'NONE', #1406, 0.004059536337672174817 ) ;
#11549=CARTESIAN_POINT ( 'NONE',  ( 198.8360742877594589, -1.073648941537930668, -18.15054426878710103 ) ) ;
#11557=CONICAL_SURFACE ( 'NONE', #9170, 13.07248899748297433, 0.6693469023067423196 ) ;
#11566=DIRECTION ( 'NONE',  ( -0.8660254037844357100, -0.5000000000000051070, 0.000000000000000000 ) ) ;
#11574=CARTESIAN_POINT ( 'NONE',  ( 200.4103230900084895, 6.823642366611345267, -3.481206571632855074 ) ) ;
#11576=B_SPLINE_CURVE_WITH_KNOTS ( 'NONE', 3,
 ( #11912, #2262, #8716, #7122 ),
 .UNSPECIFIED., .F., .F.,
 ( 4, 4 ),
 ( 2.508483997137242450E-05, 0.0008790705779558581102 ),
 .UNSPECIFIED. ) ;
#11581=VERTEX_POINT ( 'NONE', #12361 ) ;
#11583=EDGE_LOOP ( 'NONE', ( #3492, #1045, #6002, #9969 ) ) ;
#11585=EDGE_CURVE ( 'NONE', #11248, #7589, #18024, .T. ) ;
#11587=ORIENTED_EDGE ( 'NONE', *, *, #17326, .T. ) ;
#11588=DIRECTION ( 'NONE',  ( -0.5000000000000049960, 0.8660254037844357100, -0.000000000000000000 ) ) ;
#11593=ORIENTED_EDGE ( 'NONE', *, *, #18317, .F. ) ;
#11595=VECTOR ( 'NONE', #7273, 1000.000000000000114 ) ;
#11603=ADVANCED_FACE ( 'NONE', ( #20604 ), #8873, .T. ) ;
#11604=DIRECTION ( 'NONE',  ( -0.8660254037844362651, -0.5000000000000043299, 0.000000000000000000 ) ) ;
#11605=AXIS2_PLACEMENT_3D ( 'NONE', #9849, #3197, #9650 ) ;
#11606=AXIS2_PLACEMENT_3D ( 'NONE', #17558, #17451, #2930 ) ;
#11607=ORIENTED_EDGE ( 'NONE', *, *, #16252, .F. ) ;
#11609=FACE_OUTER_BOUND ( 'NONE', #14281, .T. ) ;
#11610=CARTESIAN_POINT ( 'NONE',  ( 198.6293134455681013, -1.450621593242038099, -12.64773574313024440 ) ) ;
#11611=DIRECTION ( 'NONE',  ( -0.5000000000000049960, 0.8660254037844358210, -0.000000000000000000 ) ) ;
#11615=LINE ( 'NONE', #19078, #6680 ) ;
#11616=DIRECTION ( 'NONE',  ( -0.8645602258681711616, -0.4991540791356389728, 0.05814482891047952767 ) ) ;
#11623=ORIENTED_EDGE ( 'NONE', *, *, #20728, .T. ) ;
#11624=DIRECTION ( 'NONE',  ( 0.9987303135603804449, 0.000000000000000000, -0.05037619254751497799 ) ) ;
#11632=EDGE_LOOP ( 'NONE', ( #11838, #11518, #5825, #7857 ) ) ;
#11633=ORIENTED_EDGE ( 'NONE', *, *, #6679, .T. ) ;
#11636=CARTESIAN_POINT ( 'NONE',  ( 205.0662616026534693, 10.91332106064940888, -14.00000000000005507 ) ) ;
#11646=ORIENTED_EDGE ( 'NONE', *, *, #9668, .T. ) ;
#11647=CARTESIAN_POINT ( 'NONE',  ( 199.7687975563032410, 10.75426524862079702, -3.125199447383416818 ) ) ;
#11653=LINE ( 'NONE', #15063, #20755 ) ;
#11654=CARTESIAN_POINT ( 'NONE',  ( 205.1848235957376403, 9.226162161231169279, -26.45271578590682893 ) ) ;
#11656=VERTEX_POINT ( 'NONE', #10852 ) ;
#11658=EDGE_LOOP ( 'NONE', ( #16065, #1849, #19415, #11769 ) ) ;
#11661=CARTESIAN_POINT ( 'NONE',  ( 208.8577037357181894, 4.346350652224121092, -14.00000000000005507 ) ) ;
#11662=B_SPLINE_CURVE_WITH_KNOTS ( 'NONE', 3,
 ( #18394, #13632, #3863, #16803 ),
 .UNSPECIFIED., .F., .F.,
 ( 4, 4 ),
 ( 1.122767056911022901E-06, 0.0008551085050338230699 ),
 .UNSPECIFIED. ) ;
#11663=EDGE_CURVE ( 'NONE', #4355, #10895, #15552, .T. ) ;
#11664=ORIENTED_EDGE ( 'NONE', *, *, #20760, .F. ) ;
#11668=ORIENTED_EDGE ( 'NONE', *, *, #14383, .F. ) ;
#11670=DIRECTION ( 'NONE',  ( 0.5547001962252220419, 0.000000000000000000, -0.8320502943378484950 ) ) ;
#11671=CARTESIAN_POINT ( 'NONE',  ( 188.4110494209243711, 14.81154003564305199, -14.01558723443171850 ) ) ;
#11674=LINE ( 'NONE', #18038, #19992 ) ;
#11677=EDGE_CURVE ( 'NONE', #5830, #14733, #19202, .T. ) ;
#11685=ORIENTED_EDGE ( 'NONE', *, *, #9163, .T. ) ;
#11696=ORIENTED_EDGE ( 'NONE', *, *, #14627, .T. ) ;
#11699=CONICAL_SURFACE ( 'NONE', #13746, 10.85470691220533190, 0.8171114040043576665 ) ;
#11700=EDGE_CURVE ( 'NONE', #2960, #14504, #12381, .T. ) ;
#11704=CARTESIAN_POINT ( 'NONE',  ( 195.8395605881523522, 4.361721309946301695, -9.913166705713630122 ) ) ;
#11708=EDGE_CURVE ( 'NONE', #15696, #20836, #19044, .T. ) ;
#11710=VECTOR ( 'NONE', #5072, 1000.000000000000227 ) ;
#11711=ADVANCED_FACE ( 'NONE', ( #1635 ), #5126, .T. ) ;
#11712=DIRECTION ( 'NONE',  ( 0.5000000000000049960, -0.8660254037844358210, 0.000000000000000000 ) ) ;
#11714=AXIS2_PLACEMENT_3D ( 'NONE', #7079, #16426, #20018 ) ;
#11716=LINE ( 'NONE', #18279, #20848 ) ;
#11720=ADVANCED_FACE ( 'NONE', ( #12878 ), #1536, .F. ) ;
#11734=ORIENTED_EDGE ( 'NONE', *, *, #7428, .T. ) ;
#11740=ORIENTED_EDGE ( 'NONE', *, *, #1095, .F. ) ;
#11743=DIRECTION ( 'NONE',  ( -0.3886714912512298503, -0.2243995901002338311, -0.8936326403234118310 ) ) ;
#11747=CIRCLE ( 'NONE', #6304, 12.47473710546057823 ) ;
#11751=DIRECTION ( 'NONE',  ( -0.2483788854153071435, -0.1434016163555487389, -0.9579895123154875680 ) ) ;
#11754=LINE ( 'NONE', #3679, #3146 ) ;
#11760=VERTEX_POINT ( 'NONE', #4811 ) ;
#11769=ORIENTED_EDGE ( 'NONE', *, *, #2121, .F. ) ;
#11775=CARTESIAN_POINT ( 'NONE',  ( 208.1960812450810465, 4.072754371081482638, -2.187257959407754804 ) ) ;
#11777=ORIENTED_EDGE ( 'NONE', *, *, #19257, .T. ) ;
#11784=ORIENTED_EDGE ( 'NONE', *, *, #19219, .F. ) ;
#11786=CARTESIAN_POINT ( 'NONE',  ( 199.0852767235472527, -1.187371071960172664, -9.928836400542227381 ) ) ;
#11792=ORIENTED_EDGE ( 'NONE', *, *, #14511, .F. ) ;
#11799=CARTESIAN_POINT ( 'NONE',  ( 210.7763206480203166, 12.98546375133203767, -24.38552490958320718 ) ) ;
#11802=CARTESIAN_POINT ( 'NONE',  ( 219.1264567230215050, 10.64100881942120580, -12.59769448420680504 ) ) ;
#11804=EDGE_CURVE ( 'NONE', #2174, #4567, #4909, .T. ) ;
#11808=CARTESIAN_POINT ( 'NONE',  ( 195.9478142713745399, 8.548219520498097523, -21.59012016402711254 ) ) ;
#11813=AXIS2_PLACEMENT_3D ( 'NONE', #17491, #16018, #2966 ) ;
#11818=LINE ( 'NONE', #16585, #12740 ) ;
#11820=PLANE ( 'NONE',  #16404 ) ;
#11821=VERTEX_POINT ( 'NONE', #6693 ) ;
#11826=CIRCLE ( 'NONE', #9781, 1.003313105759049417 ) ;
#11827=VERTEX_POINT ( 'NONE', #5110 ) ;
#11828=EDGE_CURVE ( 'NONE', #6449, #310, #16167, .T. ) ;
#11834=DIRECTION ( 'NONE',  ( -0.8660254037844355990, -0.5000000000000055511, 0.000000000000000000 ) ) ;
#11836=ORIENTED_EDGE ( 'NONE', *, *, #1889, .F. ) ;
#11838=ORIENTED_EDGE ( 'NONE', *, *, #17793, .T. ) ;
#11846=DIRECTION ( 'NONE',  ( -0.8660254037844355990, -0.5000000000000054401, -2.934143223514386573E-14 ) ) ;
#11847=AXIS2_PLACEMENT_3D ( 'NONE', #8244, #11336, #19481 ) ;
#11849=LINE ( 'NONE', #16617, #194 ) ;
#11850=DIRECTION ( 'NONE',  ( 0.7951984747223580507, 0.4591080534401394408, -0.3960797660391671138 ) ) ;
#11852=ADVANCED_FACE ( 'NONE', ( #20808 ), #15668, .T. ) ;
#11853=AXIS2_PLACEMENT_3D ( 'NONE', #10325, #20094, #20196 ) ;
#11854=CARTESIAN_POINT ( 'NONE',  ( 218.7874248973968179, 10.18766947982593862, -16.70797078425240301 ) ) ;
#11855=CIRCLE ( 'NONE', #20318, 11.94520687646042667 ) ;
#11860=EDGE_CURVE ( 'NONE', #10920, #4917, #413, .T. ) ;
#11865=CIRCLE ( 'NONE', #2731, 11.98469917212512215 ) ;
#11870=ORIENTED_EDGE ( 'NONE', *, *, #9784, .T. ) ;
#11872=DIRECTION ( 'NONE',  ( -0.8660254037844354880, -0.5000000000000055511, 0.000000000000000000 ) ) ;
#11875=CARTESIAN_POINT ( 'NONE',  ( 215.6983787324637376, 15.82721531135244675, -16.75125533358882279 ) ) ;
#11879=ORIENTED_EDGE ( 'NONE', *, *, #17168, .F. ) ;
#11883=AXIS2_PLACEMENT_3D ( 'NONE', #15836, #15742, #5951 ) ;
#11885=CARTESIAN_POINT ( 'NONE',  ( 214.9440738535968762, 8.483915958974842297, -23.86786078788951571 ) ) ;
#11887=ADVANCED_FACE ( 'NONE', ( #667 ), #18164, .F. ) ;
#11892=ORIENTED_EDGE ( 'NONE', *, *, #4504, .T. ) ;
#11895=EDGE_CURVE ( 'NONE', #7807, #15357, #6000, .T. ) ;
#11901=ORIENTED_EDGE ( 'NONE', *, *, #1850, .T. ) ;
#11902=AXIS2_PLACEMENT_3D ( 'NONE', #12157, #7362, #18618 ) ;
#11904=DIRECTION ( 'NONE',  ( -0.7499999999999953371, -0.4330127018922227400, 0.5000000000000039968 ) ) ;
#11905=ORIENTED_EDGE ( 'NONE', *, *, #18844, .T. ) ;
#11909=CARTESIAN_POINT ( 'NONE',  ( 198.4821375217713353, 5.887413813925527428, -22.72623880687287468 ) ) ;
#11912=CARTESIAN_POINT ( 'NONE',  ( 208.2224579217690632, 4.087982952467670295, -25.92587471718749725 ) ) ;
#11917=VERTEX_POINT ( 'NONE', #16782 ) ;
#11918=AXIS2_PLACEMENT_3D ( 'NONE', #3629, #19634, #18063 ) ;
#11925=ORIENTED_EDGE ( 'NONE', *, *, #4152, .F. ) ;
#11928=CYLINDRICAL_SURFACE ( 'NONE', #1592, 12.47473710546057646 ) ;
#11935=LINE ( 'NONE', #5649, #3878 ) ;
#11939=VERTEX_POINT ( 'NONE', #18264 ) ;
#11943=VECTOR ( 'NONE', #19714, 1000.000000000000114 ) ;
#11947=CIRCLE ( 'NONE', #19013, 3.845804376225747667 ) ;
#11950=ORIENTED_EDGE ( 'NONE', *, *, #10282, .T. ) ;
#11953=DIRECTION ( 'NONE',  ( 0.6634139481689433904, 0.3830222215594970003, 0.6427876096865293709 ) ) ;
#11958=ORIENTED_EDGE ( 'NONE', *, *, #13146, .F. ) ;
#11961=EDGE_CURVE ( 'NONE', #20547, #5368, #11576, .T. ) ;
#11965=DIRECTION ( 'NONE',  ( 0.5000000000000054401, -0.8660254037844354880, 0.000000000000000000 ) ) ;
#11973=ORIENTED_EDGE ( 'NONE', *, *, #14435, .T. ) ;
#11974=ORIENTED_EDGE ( 'NONE', *, *, #1765, .T. ) ;
#11982=EDGE_CURVE ( 'NONE', #14131, #16845, #19948, .T. ) ;
#11985=DIRECTION ( 'NONE',  ( 0.9949159024423659403, 0.000000000000000000, 0.1007092203688055299 ) ) ;
#11988=VECTOR ( 'NONE', #20572, 1000.000000000000227 ) ;
#11993=DIRECTION ( 'NONE',  ( -0.2483788854152947367, -0.1434016163555419388, 0.9579895123154918979 ) ) ;
#11996=CARTESIAN_POINT ( 'NONE',  ( 216.3916581709072489, 15.88978658501442887, -14.00519583319098871 ) ) ;
#11997=LINE ( 'NONE', #10270, #7567 ) ;
#11998=DIRECTION ( 'NONE',  ( 0.8660254037844355990, 0.5000000000000054401, 0.000000000000000000 ) ) ;
#12001=EDGE_CURVE ( 'NONE', #9686, #2725, #11252, .T. ) ;
#12008=CARTESIAN_POINT ( 'NONE',  ( 206.2111997916997552, 10.34978999605213268, -14.00000000000005507 ) ) ;
#12012=DIRECTION ( 'NONE',  ( -0.1997192025788092351, -0.1153079353712145594, 0.9730448705798270259 ) ) ;
#12013=CARTESIAN_POINT ( 'NONE',  ( 189.5662401447910383, 15.47848971103284477, -19.61257667712936126 ) ) ;
#12017=VECTOR ( 'NONE', #10741, 1000.000000000000114 ) ;
#12018=DIRECTION ( 'NONE',  ( -0.8660254037844354880, -0.5000000000000055511, 0.000000000000000000 ) ) ;
#12021=CYLINDRICAL_SURFACE ( 'NONE', #7113, 12.47473710546057646 ) ;
#12022=EDGE_CURVE ( 'NONE', #4848, #437, #10944, .T. ) ;
#12024=CARTESIAN_POINT ( 'NONE',  ( 196.2703485803101842, 4.433426968998789519, -19.44895743303468905 ) ) ;
#12028=ORIENTED_EDGE ( 'NONE', *, *, #19792, .T. ) ;
#12032=FACE_OUTER_BOUND ( 'NONE', #3238, .T. ) ;
#12041=ORIENTED_EDGE ( 'NONE', *, *, #11663, .T. ) ;
#12044=CARTESIAN_POINT ( 'NONE',  ( 215.7779675912125867, 15.87316596037559968, -12.64773574313060678 ) ) ;
#12047=AXIS2_PLACEMENT_3D ( 'NONE', #4781, #17516, #14454 ) ;
#12049=ORIENTED_EDGE ( 'NONE', *, *, #7381, .F. ) ;
#12052=VECTOR ( 'NONE', #15599, 1000.000000000000227 ) ;
#12056=ORIENTED_EDGE ( 'NONE', *, *, #10911, .F. ) ;
#12065=DIRECTION ( 'NONE',  ( -0.8660254037844363761, -0.5000000000000037748, 0.000000000000000000 ) ) ;
#12068=DIRECTION ( 'NONE',  ( 0.6048098792058420603, 0.000000000000000000, -0.7963698952214447457 ) ) ;
#12069=ORIENTED_EDGE ( 'NONE', *, *, #4038, .T. ) ;
#12071=DIRECTION ( 'NONE',  ( 0.7500000000000013323, 0.4330127018922261817, 0.4999999999999918954 ) ) ;
#12080=CARTESIAN_POINT ( 'NONE',  ( 208.0983737146324870, 5.661548828456886895, -14.00000000000005507 ) ) ;
#12084=CARTESIAN_POINT ( 'NONE',  ( 200.2585560139914378, -0.5099779577875940273, -20.52105855319921801 ) ) ;
#12085=ADVANCED_FACE ( 'NONE', ( #5628, #4269 ), #15830, .F. ) ;
#12086=LINE ( 'NONE', #20342, #17404 ) ;
#12091=AXIS2_PLACEMENT_3D ( 'NONE', #1589, #15813, #12423 ) ;
#12097=EDGE_CURVE ( 'NONE', #9868, #330, #1480, .T. ) ;
#12101=CYLINDRICAL_SURFACE ( 'NONE', #13903, 12.47473710546057646 ) ;
#12107=B_SPLINE_CURVE_WITH_KNOTS ( 'NONE', 3,
 ( #5364, #4744, #4851, #16204 ),
 .UNSPECIFIED., .F., .F.,
 ( 4, 4 ),
 ( 7.900540974747862941E-05, 0.0007516562018010966269 ),
 .UNSPECIFIED. ) ;
#12108=LINE ( 'NONE', #15728, #13685 ) ;
#12113=FACE_OUTER_BOUND ( 'NONE', #6920, .T. ) ;
#12115=EDGE_LOOP ( 'NONE', ( #15433, #5040, #17822, #1168 ) ) ;
#12121=PRODUCT ( 'Drill Bit Indexing Pin', 'Drill Bit Indexing Pin', '', ( #16770 ) ) ;
#12123=CIRCLE ( 'NONE', #9729, 12.47473710546057823 ) ;
#12126=DIRECTION ( 'NONE',  ( -0.5000000000000049960, 0.8660254037844358210, 0.000000000000000000 ) ) ;
#12128=EDGE_LOOP ( 'NONE', ( #5203, #13751, #15534, #10890 ) ) ;
#12139=DIRECTION ( 'NONE',  ( 0.8296432542242747621, 0.4789947561577490021, -0.2868032327110942581 ) ) ;
#12140=EDGE_CURVE ( 'NONE', #184, #16451, #5488, .T. ) ;
#12141=ORIENTED_EDGE ( 'NONE', *, *, #1252, .T. ) ;
#12143=CARTESIAN_POINT ( 'NONE',  ( 217.4610193877672941, 9.421868901786666584, -7.448751785191543462 ) ) ;
#12146=CARTESIAN_POINT ( 'NONE',  ( 205.5965122587965084, 9.994899983462953941, -14.00000000000005507 ) ) ;
#12147=CARTESIAN_POINT ( 'NONE',  ( 195.8472345282168874, 4.366151861308305016, -18.11117897393217646 ) ) ;
#12150=B_SPLINE_CURVE_WITH_KNOTS ( 'NONE', 3,
 ( #17469, #13986, #9385, #12395 ),
 .UNSPECIFIED., .F., .F.,
 ( 4, 4 ),
 ( 5.481513501348629134E-07, 0.0006731989433939361729 ),
 .UNSPECIFIED. ) ;
#12157=CARTESIAN_POINT ( 'NONE',  ( 205.0662616026534693, 10.91332106064940888, -14.00000000000005507 ) ) ;
#12159=ORIENTED_EDGE ( 'NONE', *, *, #11068, .T. ) ;
#12162=CARTESIAN_POINT ( 'NONE',  ( 205.5965122587965084, 9.994899983462953941, -14.00000000000005507 ) ) ;
#12166=ORIENTED_EDGE ( 'NONE', *, *, #10300, .T. ) ;
#12168=B_SPLINE_CURVE_WITH_KNOTS ( 'NONE', 3,
 ( #5190, #6778, #16149, #13272 ),
 .UNSPECIFIED., .F., .F.,
 ( 4, 4 ),
 ( 0.0001032701082515755423, 0.0009572558462284362375 ),
 .UNSPECIFIED. ) ;
#12173=LINE ( 'NONE', #8976, #16606 ) ;
#12176=ORIENTED_EDGE ( 'NONE', *, *, #12022, .T. ) ;
#12179=VERTEX_POINT ( 'NONE', #10827 ) ;
#12185=AXIS2_PLACEMENT_3D ( 'NONE', #8424, #3150, #5142 ) ;
#12189=EDGE_LOOP ( 'NONE', ( #11162, #17505, #15759, #19715 ) ) ;
#12191=LINE ( 'NONE', #2550, #4994 ) ;
#12193=ADVANCED_FACE ( 'NONE', ( #15735 ), #14254, .T. ) ;
#12201=ORIENTED_EDGE ( 'NONE', *, *, #10376, .F. ) ;
#12203=VECTOR ( 'NONE', #15330, 1000.000000000000114 ) ;
#12206=ORIENTED_EDGE ( 'NONE', *, *, #2629, .F. ) ;
#12209=VERTEX_POINT ( 'NONE', #8159 ) ;
#12211=CARTESIAN_POINT ( 'NONE',  ( 196.9187795697884269, 4.984808679508447860, -7.425127016398286983 ) ) ;
#12214=VECTOR ( 'NONE', #31, 1000.000000000000000 ) ;
#12215=EDGE_CURVE ( 'NONE', #2199, #5956, #8796, .T. ) ;
#12218=ORIENTED_EDGE ( 'NONE', *, *, #3575, .T. ) ;
#12221=DIRECTION ( 'NONE',  ( 0.5000000000000051070, -0.8660254037844359321, 0.000000000000000000 ) ) ;
#12223=CARTESIAN_POINT ( 'NONE',  ( 205.5965122587965084, 9.994899983462953941, -14.00000000000005507 ) ) ;
#12227=FACE_OUTER_BOUND ( 'NONE', #7921, .T. ) ;
#12234=AXIS2_PLACEMENT_3D ( 'NONE', #2827, #20818, #4516 ) ;
#12239=EDGE_LOOP ( 'NONE', ( #6691, #8679, #19164, #7609 ) ) ;
#12242=ORIENTED_EDGE ( 'NONE', *, *, #3134, .T. ) ;
#12245=ORIENTED_EDGE ( 'NONE', *, *, #12140, .T. ) ;
#12250=ORIENTED_EDGE ( 'NONE', *, *, #2493, .T. ) ;
#12252=AXIS2_PLACEMENT_3D ( 'NONE', #2068, #3965, #10414 ) ;
#12257=ADVANCED_FACE ( 'NONE', ( #3100 ), #6497, .T. ) ;
#12259=CARTESIAN_POINT ( 'NONE',  ( 215.2800591377192916, 15.23167179936302240, -8.480087152951449880 ) ) ;
#12264=VERTEX_POINT ( 'NONE', #15937 ) ;
#12272=ORIENTED_EDGE ( 'NONE', *, *, #7420, .F. ) ;
#12274=DIRECTION ( 'NONE',  ( 0.8660254037844377084, 0.5000000000000015543, 0.000000000000000000 ) ) ;
#12276=PLANE ( 'NONE',  #18841 ) ;
#12278=CARTESIAN_POINT ( 'NONE',  ( 206.2111997916997552, 10.34978999605213623, -2.187257959407755248 ) ) ;
#12280=EDGE_CURVE ( 'NONE', #14638, #18324, #8053, .T. ) ;
#12284=DIRECTION ( 'NONE',  ( -0.5000000000000054401, 0.8660254037844354880, -0.000000000000000000 ) ) ;
#12285=VECTOR ( 'NONE', #18349, 1000.000000000000000 ) ;
#12293=ORIENTED_EDGE ( 'NONE', *, *, #11804, .T. ) ;
#12294=CYLINDRICAL_SURFACE ( 'NONE', #20001, 12.47473710546057646 ) ;
#12296=ADVANCED_FACE ( 'NONE', ( #17934 ), #13289, .T. ) ;
#12297=LINE ( 'NONE', #15792, #20582 ) ;
#12301=LINE ( 'NONE', #14633, #2779 ) ;
#12304=CARTESIAN_POINT ( 'NONE',  ( 195.3173534746875930, 3.529175630622251258, -16.89203719259486647 ) ) ;
#12309=ORIENTED_EDGE ( 'NONE', *, *, #17154, .F. ) ;
#12314=LINE ( 'NONE', #7301, #4371 ) ;
#12316=DIRECTION ( 'NONE',  ( 0.4330127018922209636, 0.2500000000000048850, 0.8660254037844363761 ) ) ;
#12319=ORIENTED_EDGE ( 'NONE', *, *, #9648, .T. ) ;
#12320=CARTESIAN_POINT ( 'NONE',  ( 212.0325450024346026, 6.287737754125841683, -1.381056684022670344 ) ) ;
#12321=DIRECTION ( 'NONE',  ( -0.5000000000000051070, 0.8660254037844359321, -0.000000000000000000 ) ) ;
#12328=DIRECTION ( 'NONE',  ( 0.5000000000000054401, -0.8660254037844354880, 0.000000000000000000 ) ) ;
#12329=CONICAL_SURFACE ( 'NONE', #6882, 13.07248899748297433, 0.6693469023067423196 ) ;
#12331=VERTEX_POINT ( 'NONE', #1710 ) ;
#12333=CARTESIAN_POINT ( 'NONE',  ( 217.9607779367323985, 9.710404634561534465, -8.669480444820854004 ) ) ;
#12334=DIRECTION ( 'NONE',  ( -0.5000000000000054401, 0.8660254037844354880, -0.000000000000000000 ) ) ;
#12335=CARTESIAN_POINT ( 'NONE',  ( 204.3878836909736094, 13.42109587188279285, -25.81526893633800412 ) ) ;
#12337=EDGE_CURVE ( 'NONE', #8757, #3195, #4820, .T. ) ;
#12343=EDGE_LOOP ( 'NONE', ( #6506, #19374, #11481, #6401, #11133, #10357 ) ) ;
#12346=EDGE_CURVE ( 'NONE', #3585, #12762, #1817, .T. ) ;
#12347=CARTESIAN_POINT ( 'NONE',  ( 195.9720064151970007, 8.562186861246273040, -6.376588578941770002 ) ) ;
#12350=ORIENTED_EDGE ( 'NONE', *, *, #12388, .F. ) ;
#12351=EDGE_LOOP ( 'NONE', ( #11003, #12766, #3718, #798, #10253, #6943 ) ) ;
#12358=AXIS2_PLACEMENT_3D ( 'NONE', #8414, #380, #20085 ) ;
#12361=CARTESIAN_POINT ( 'NONE',  ( 218.5272241891094325, 10.03744253085286964, -18.09983247376310089 ) ) ;
#12363=CARTESIAN_POINT ( 'NONE',  ( 215.0732969577928202, 15.28931427629719231, -8.544894389633146403 ) ) ;
#12365=DIRECTION ( 'NONE',  ( -0.5000000000000054401, 0.8660254037844354880, -0.000000000000000000 ) ) ;
#12366=ADVANCED_FACE ( 'NONE', ( #16439 ), #10057, .F. ) ;
#12370=VERTEX_POINT ( 'NONE', #13370 ) ;
#12371=VERTEX_POINT ( 'NONE', #14873 ) ;
#12375=CIRCLE ( 'NONE', #6926, 11.98469917212512215 ) ;
#12380=CARTESIAN_POINT ( 'NONE',  ( 195.4216187824635824, 18.83910615367633667, -14.00000000000005507 ) ) ;
#12381=B_SPLINE_CURVE_WITH_KNOTS ( 'NONE', 3,
 ( #9150, #18921, #9252, #15757 ),
 .UNSPECIFIED., .F., .F.,
 ( 4, 4 ),
 ( 4.507033345943735000E-05, 0.0007177211255159268027 ),
 .UNSPECIFIED. ) ;
#12382=CARTESIAN_POINT ( 'NONE',  ( 193.6293134455680445, 7.209632444602317669, -12.64773574313024085 ) ) ;
#12385=VERTEX_POINT ( 'NONE', #13267 ) ;
#12388=EDGE_CURVE ( 'NONE', #16780, #18827, #18680, .T. ) ;
#12393=VECTOR ( 'NONE', #11049, 1000.000000000000114 ) ;
#12394=EDGE_CURVE ( 'NONE', #340, #18388, #644, .T. ) ;
#12395=CARTESIAN_POINT ( 'NONE',  ( 214.8766030929655813, 15.35276292467472103, -19.36714384557541990 ) ) ;
#12397=ORIENTED_EDGE ( 'NONE', *, *, #2373, .F. ) ;
#12400=CARTESIAN_POINT ( 'NONE',  ( 208.4761278624580711, 5.007259451653140125, -14.00000000000005507 ) ) ;
#12403=CARTESIAN_POINT ( 'NONE',  ( 209.3577481411912231, 3.480248335904271961, -14.00000000000005507 ) ) ;
#12404=PLANE ( 'NONE',  #8129 ) ;
#12406=CIRCLE ( 'NONE', #4609, 2.961423854602166283 ) ;
#12409=ADVANCED_FACE ( 'NONE', ( #3817 ), #20062, .T. ) ;
#12410=ADVANCED_FACE ( 'NONE', ( #16654 ), #5186, .F. ) ;
#12418=EDGE_CURVE ( 'NONE', #16451, #13417, #6888, .T. ) ;
#12422=TOROIDAL_SURFACE ( 'NONE', #5952, 1.003313105759043200, 1.000000000000000000 ) ;
#12423=DIRECTION ( 'NONE',  ( -0.8660254037844355990, -0.5000000000000054401, -1.682612938603036717E-14 ) ) ;
#12426=CONICAL_SURFACE ( 'NONE', #3266, 13.07248899748297433, 0.6693469023067423196 ) ;
#12427=VERTEX_POINT ( 'NONE', #7099 ) ;
#12436=CARTESIAN_POINT ( 'NONE',  ( 210.0179110316588265, 27.28626740294374287, -14.01558723443205068 ) ) ;
#12445=CARTESIAN_POINT ( 'NONE',  ( 199.4075733045063146, 6.421714412205289157, -4.379064819896086647 ) ) ;
#12447=ORIENTED_EDGE ( 'NONE', *, *, #19854, .F. ) ;
#12448=LINE ( 'NONE', #2898, #3056 ) ;
#12451=DIRECTION ( 'NONE',  ( 0.6634139481689351747, 0.3830222215594923374, -0.6427876096865405842 ) ) ;
#12454=VERTEX_POINT ( 'NONE', #2137 ) ;
#12459=CARTESIAN_POINT ( 'NONE',  ( 205.5965122587965084, 9.994899983462953941, -14.00000000000005507 ) ) ;
#12461=ORIENTED_EDGE ( 'NONE', *, *, #18053, .T. ) ;
#12464=AXIS2_PLACEMENT_3D ( 'NONE', #20378, #5531, #5631 ) ;
#12465=ORIENTED_EDGE ( 'NONE', *, *, #1330, .T. ) ;
#12470=CARTESIAN_POINT ( 'NONE',  ( 214.9383172013976093, 8.738206206044257129, -4.003039906354144861 ) ) ;
#12472=VERTEX_POINT ( 'NONE', #13161 ) ;
#12475=VERTEX_POINT ( 'NONE', #14771 ) ;
#12486=CARTESIAN_POINT ( 'NONE',  ( 205.5965122587965084, 9.994899983462953941, -14.00000000000005507 ) ) ;
#12493=ORIENTED_EDGE ( 'NONE', *, *, #561, .T. ) ;
#12498=ORIENTED_EDGE ( 'NONE', *, *, #9794, .F. ) ;
#12499=LINE ( 'NONE', #18959, #4471 ) ;
#12500=CARTESIAN_POINT ( 'NONE',  ( 199.2243387870319395, 21.03182819120163671, -14.00000000000005507 ) ) ;
#12507=DIRECTION ( 'NONE',  ( -0.5000000000000054401, 0.8660254037844354880, -0.000000000000000000 ) ) ;
#12508=ORIENTED_EDGE ( 'NONE', *, *, #11329, .F. ) ;
#12510=LINE ( 'NONE', #17490, #14040 ) ;
#12514=ORIENTED_EDGE ( 'NONE', *, *, #12140, .F. ) ;
#12515=CARTESIAN_POINT ( 'NONE',  ( 195.0945143319839872, 3.400519391596340757, -15.43274561385865695 ) ) ;
#12518=EDGE_CURVE ( 'NONE', #18037, #15665, #13615, .T. ) ;
#12529=DIRECTION ( 'NONE',  ( 0.3886714912512297393, 0.2243995901002339699, 0.8936326403234117199 ) ) ;
#12533=CARTESIAN_POINT ( 'NONE',  ( 202.0355941508142337, 1.288815579510670828, -24.01557619556968248 ) ) ;
#12537=LINE ( 'NONE', #4265, #9424 ) ;
#12538=DIRECTION ( 'NONE',  ( -0.5000000000000049960, 0.8660254037844358210, -0.000000000000000000 ) ) ;
#12539=LINE ( 'NONE', #17305, #15632 ) ;
#12545=FACE_OUTER_BOUND ( 'NONE', #13513, .T. ) ;
#12547=VERTEX_POINT ( 'NONE', #5706 ) ;
#12550=EDGE_CURVE ( 'NONE', #10440, #7006, #8209, .T. ) ;
#12551=DIRECTION ( 'NONE',  ( -0.8660254037844355990, -0.5000000000000055511, 0.000000000000000000 ) ) ;
#12557=ORIENTED_EDGE ( 'NONE', *, *, #9539, .F. ) ;
#12565=DIRECTION ( 'NONE',  ( 0.7366891686653773696, 0.000000000000000000, -0.6762315200958287642 ) ) ;
#12567=FACE_OUTER_BOUND ( 'NONE', #17137, .T. ) ;
#12570=( NAMED_UNIT ( * ) PLANE_ANGLE_UNIT ( ) SI_UNIT ( $, .RADIAN. ) );
#12572=ORIENTED_EDGE ( 'NONE', *, *, #3830, .F. ) ;
#12585=DIRECTION ( 'NONE',  ( 0.5000000000000054401, -0.8660254037844354880, 0.000000000000000000 ) ) ;
#12593=CARTESIAN_POINT ( 'NONE',  ( 213.9717500725588479, 7.407338323375970646, -24.35247136794745515 ) ) ;
#12595=CARTESIAN_POINT ( 'NONE',  ( 199.2231352798572743, 21.03391272677540513, -14.00000000000005507 ) ) ;
#12596=AXIS2_PLACEMENT_3D ( 'NONE', #18041, #14878, #14464 ) ;
#12599=CARTESIAN_POINT ( 'NONE',  ( 190.1809276776941715, 15.83337972362198265, -20.84195174293567376 ) ) ;
#12602=CARTESIAN_POINT ( 'NONE',  ( 195.3173534746875930, 3.529175630622251258, -16.89203719259486647 ) ) ;
#12609=CARTESIAN_POINT ( 'NONE',  ( 216.7494463307476451, 9.526248244645403318, -6.098918798390618790 ) ) ;
#12610=CARTESIAN_POINT ( 'NONE',  ( 195.1593178475889374, 3.614956399211269655, -15.42323214253203112 ) ) ;
#12615=ORIENTED_EDGE ( 'NONE', *, *, #17670, .T. ) ;
#12627=DIRECTION ( 'NONE',  ( -1.000000000000000000, 0.000000000000000000, 0.000000000000000000 ) ) ;
#12629=ORIENTED_EDGE ( 'NONE', *, *, #19483, .F. ) ;
#12630=VECTOR ( 'NONE', #6160, 1000.000000000000114 ) ;
#12634=VERTEX_POINT ( 'NONE', #7206 ) ;
#12642=EDGE_CURVE ( 'NONE', #11172, #18411, #4657, .T. ) ;
#12646=CARTESIAN_POINT ( 'NONE',  ( 210.7370931664818272, 12.96281575430614552, -3.762296834228894493 ) ) ;
#12658=LINE ( 'NONE', #15639, #4433 ) ;
#12660=LINE ( 'NONE', #19019, #4472 ) ;
#12664=VERTEX_POINT ( 'NONE', #17495 ) ;
#12667=EDGE_CURVE ( 'NONE', #9307, #20827, #4961, .T. ) ;
#12670=CARTESIAN_POINT ( 'NONE',  ( 217.9776690748798558, 9.720156737717866591, -19.29168348739315775 ) ) ;
#12678=( NAMED_UNIT ( * ) SI_UNIT ( $, .STERADIAN. ) SOLID_ANGLE_UNIT ( ) );
#12680=DIRECTION ( 'NONE',  ( -0.8660254037844355990, -0.5000000000000055511, 0.000000000000000000 ) ) ;
#12690=LINE ( 'NONE', #4620, #1410 ) ;
#12695=ORIENTED_EDGE ( 'NONE', *, *, #5232, .T. ) ;
#12696=DIRECTION ( 'NONE',  ( 0.5000000000000051070, -0.8660254037844359321, 0.000000000000000000 ) ) ;
#12697=DIRECTION ( 'NONE',  ( -0.5000000000000049960, 0.8660254037844357100, -0.000000000000000000 ) ) ;
#12699=LINE ( 'NONE', #9698, #803 ) ;
#12700=AXIS2_PLACEMENT_3D ( 'NONE', #10966, #11069, #14275 ) ;
#12705=DIRECTION ( 'NONE',  ( -0.8660254037844357100, -0.5000000000000051070, 0.000000000000000000 ) ) ;
#12707=VERTEX_POINT ( 'NONE', #12831 ) ;
#12712=LINE ( 'NONE', #18307, #17976 ) ;
#12714=ORIENTED_EDGE ( 'NONE', *, *, #4468, .F. ) ;
#12720=CYLINDRICAL_SURFACE ( 'NONE', #5127, 7.960520131757808038 ) ;
#12723=ORIENTED_EDGE ( 'NONE', *, *, #10534, .F. ) ;
#12727=VERTEX_POINT ( 'NONE', #12937 ) ;
#12729=ORIENTED_EDGE ( 'NONE', *, *, #14736, .T. ) ;
#12730=AXIS2_PLACEMENT_3D ( 'NONE', #12080, #8576, #11872 ) ;
#12740=VECTOR ( 'NONE', #18077, 999.9999999999998863 ) ;
#12741=CARTESIAN_POINT ( 'NONE',  ( 203.6701878702990598, 1.459728612827534855, -3.762296834228767928 ) ) ;
#12742=CARTESIAN_POINT ( 'NONE',  ( 216.7607129495440859, 9.790366881806683352, -5.993340328401894013 ) ) ;
#12744=EDGE_CURVE ( 'NONE', #791, #12727, #18014, .T. ) ;
#12745=AXIS2_PLACEMENT_3D ( 'NONE', #9510, #16511, #11223 ) ;
#12751=DIRECTION ( 'NONE',  ( -0.2961981327260293506, -0.1710100716628398243, -0.9396926207859056523 ) ) ;
#12752=DIRECTION ( 'NONE',  ( 0.8645602258681711616, 0.4991540791356389728, -0.05814482891047952767 ) ) ;
#12761=ORIENTED_EDGE ( 'NONE', *, *, #7207, .T. ) ;
#12762=VERTEX_POINT ( 'NONE', #5475 ) ;
#12763=VECTOR ( 'NONE', #16083, 1000.000000000000227 ) ;
#12766=ORIENTED_EDGE ( 'NONE', *, *, #2704, .F. ) ;
#12768=CARTESIAN_POINT ( 'NONE',  ( 202.9975627544909003, 8.494395787541842324, -26.16494226148076052 ) ) ;
#12776=DIRECTION ( 'NONE',  ( -0.8660254037844354880, -0.5000000000000055511, 0.000000000000000000 ) ) ;
#12779=VECTOR ( 'NONE', #1061, 1000.000000000000114 ) ;
#12781=VECTOR ( 'NONE', #8136, 1000.000000000000227 ) ;
#12783=EDGE_CURVE ( 'NONE', #14727, #2960, #11754, .T. ) ;
#12784=CARTESIAN_POINT ( 'NONE',  ( 203.8052576239561802, 8.960718637850693113, -2.195132782454258358 ) ) ;
#12785=EDGE_CURVE ( 'NONE', #13537, #12472, #11653, .T. ) ;
#12791=DIRECTION ( 'NONE',  ( -0.5000000000000054401, 0.8660254037844354880, -0.000000000000000000 ) ) ;
#12792=EDGE_CURVE ( 'NONE', #5372, #15392, #13088, .T. ) ;
#12795=ORIENTED_EDGE ( 'NONE', *, *, #1968, .F. ) ;
#12797=PLANE ( 'NONE',  #5720 ) ;
#12798=ADVANCED_FACE ( 'NONE', ( #17913 ), #9898, .T. ) ;
#12800=DIRECTION ( 'NONE',  ( 0.5000000000000026645, -0.8660254037844370423, 0.000000000000000000 ) ) ;
#12802=DIRECTION ( 'NONE',  ( -0.5000000000000054401, 0.8660254037844354880, -0.000000000000000000 ) ) ;
#12804=DIRECTION ( 'NONE',  ( 0.8645602258681718277, 0.4991540791356398055, 0.05814482891046528212 ) ) ;
#12809=EDGE_LOOP ( 'NONE', ( #12695, #9716, #321, #8834 ) ) ;
#12813=VECTOR ( 'NONE', #10910, 1000.000000000000000 ) ;
#12815=EDGE_CURVE ( 'NONE', #13335, #2368, #19898, .T. ) ;
#12816=ORIENTED_EDGE ( 'NONE', *, *, #17135, .F. ) ;
#12817=ORIENTED_EDGE ( 'NONE', *, *, #8061, .F. ) ;
#12818=ORIENTED_EDGE ( 'NONE', *, *, #18145, .F. ) ;
#12821=CARTESIAN_POINT ( 'NONE',  ( 215.9755601355957424, 15.98724606906508683, -13.98704593443257771 ) ) ;
#12824=ORIENTED_EDGE ( 'NONE', *, *, #6035, .T. ) ;
#12825=FACE_OUTER_BOUND ( 'NONE', #9295, .T. ) ;
#12826=CIRCLE ( 'NONE', #3659, 11.94520687646042667 ) ;
#12827=CARTESIAN_POINT ( 'NONE',  ( 200.1945581936670635, 6.876080349810432146, -24.60216584133502238 ) ) ;
#12831=CARTESIAN_POINT ( 'NONE',  ( 209.7177441667290339, 12.37429433490069997, -24.99940654434242759 ) ) ;
#12833=DIRECTION ( 'NONE',  ( -0.1005394128318207181, -0.05804645706261944010, -0.9932383577419421350 ) ) ;
#12834=LINE ( 'NONE', #11243, #46 ) ;
#12841=DIRECTION ( 'NONE',  ( -0.5000000000000051070, 0.8660254037844359321, -0.000000000000000000 ) ) ;
#12842=ADVANCED_FACE ( 'NONE', ( #1899 ), #13658, .T. ) ;
#12843=CARTESIAN_POINT ( 'NONE',  ( 205.5718816476997688, 14.10467741091863658, -2.341985411377013548 ) ) ;
#12847=ORIENTED_EDGE ( 'NONE', *, *, #5122, .T. ) ;
#12857=ADVANCED_FACE ( 'NONE', ( #3372 ), #17713, .T. ) ;
#12874=CARTESIAN_POINT ( 'NONE',  ( 196.8389703229736938, 4.584704208019711125, -20.76014333877581564 ) ) ;
#12876=CARTESIAN_POINT ( 'NONE',  ( 198.4557123656591386, 5.695147338747302612, -22.83852658738919317 ) ) ;
#12878=FACE_OUTER_BOUND ( 'NONE', #18852, .T. ) ;
#12879=CARTESIAN_POINT ( 'NONE',  ( 193.0882619218634488, 6.897256201746025717, -18.44761907388178557 ) ) ;
#12882=ORIENTED_EDGE ( 'NONE', *, *, #19159, .T. ) ;
#12884=CARTESIAN_POINT ( 'NONE',  ( 203.8353993890810898, 8.978120994059423765, -2.341985411376945159 ) ) ;
#12886=AXIS2_PLACEMENT_3D ( 'NONE', #13719, #786, #10406 ) ;
#12890=EDGE_CURVE ( 'NONE', #425, #9243, #3714, .T. ) ;
#12893=CARTESIAN_POINT ( 'NONE',  ( 216.6298941398503359, 15.83397672076898566, -14.01558723443205068 ) ) ;
#12894=DIRECTION ( 'NONE',  ( -0.8660254037844362651, -0.5000000000000043299, 0.000000000000000000 ) ) ;
#12895=VECTOR ( 'NONE', #5188, 1000.000000000000227 ) ;
#12897=CARTESIAN_POINT ( 'NONE',  ( 209.0908153953612612, 5.362149464242316199, -1.545471579934816875 ) ) ;
#12911=DIRECTION ( 'NONE',  ( -0.5000000000000051070, 0.8660254037844359321, -0.000000000000000000 ) ) ;
#12913=EDGE_LOOP ( 'NONE', ( #6495, #17071, #19830, #746 ) ) ;
#12916=CARTESIAN_POINT ( 'NONE',  ( 198.0085843809688413, -1.293793446905138422, -15.42246552719588948 ) ) ;
#12920=VERTEX_POINT ( 'NONE', #4321 ) ;
#12927=ORIENTED_EDGE ( 'NONE', *, *, #1889, .T. ) ;
#12928=CARTESIAN_POINT ( 'NONE',  ( 195.1138010445122575, 8.066701759461459176, -22.49869731917958049 ) ) ;
#12929=ADVANCED_FACE ( 'NONE', ( #16836 ), #5682, .F. ) ;
#12932=DIRECTION ( 'NONE',  ( -0.8601696498176548689, -0.4966191788709768407, 0.1160929141252376451 ) ) ;
#12937=CARTESIAN_POINT ( 'NONE',  ( 213.9513496856694132, 7.395560154513789897, -3.762296834228892717 ) ) ;
#12944=ORIENTED_EDGE ( 'NONE', *, *, #13888, .F. ) ;
#12945=ORIENTED_EDGE ( 'NONE', *, *, #10824, .F. ) ;
#12948=EDGE_CURVE ( 'NONE', #12454, #15941, #1151, .T. ) ;
#12949=VECTOR ( 'NONE', #9874, 1000.000000000000227 ) ;
#12950=VECTOR ( 'NONE', #19690, 1000.000000000000114 ) ;
#12951=FACE_OUTER_BOUND ( 'NONE', #6657, .T. ) ;
#12952=ORIENTED_EDGE ( 'NONE', *, *, #629, .F. ) ;
#12955=B_SPLINE_CURVE_WITH_KNOTS ( 'NONE', 3,
 ( #17456, #14299, #9376, #19052 ),
 .UNSPECIFIED., .F., .F.,
 ( 4, 4 ),
 ( 0.0001275232718639688831, 0.0008001740639077388690 ),
 .UNSPECIFIED. ) ;
#12958=CARTESIAN_POINT ( 'NONE',  ( 215.7669897261582435, 15.51280130567490367, -9.783550055872625606 ) ) ;
#12961=CARTESIAN_POINT ( 'NONE',  ( 215.5386005439712562, 15.73496733121568170, -17.74130751083515634 ) ) ;
#12962=DIRECTION ( 'NONE',  ( 0.5000000000000052180, -0.8660254037844355990, -5.551115123125782086E-17 ) ) ;
#12964=CARTESIAN_POINT ( 'NONE',  ( 209.4137679361615767, 3.391338277461352302, -14.00000000000005507 ) ) ;
#12965=VECTOR ( 'NONE', #9902, 1000.000000000000227 ) ;
#12966=CARTESIAN_POINT ( 'NONE',  ( 205.5254235590770406, 9.953856903543574219, -12.15027190984248229 ) ) ;
#12967=DIRECTION ( 'NONE',  ( 0.5000000000000049960, -0.8660254037844358210, 0.000000000000000000 ) ) ;
#12978=ORIENTED_EDGE ( 'NONE', *, *, #20424, .F. ) ;
#12984=CARTESIAN_POINT ( 'NONE',  ( 195.4998201364199417, 4.165572068683992768, -11.22353489230383339 ) ) ;
#12987=EDGE_CURVE ( 'NONE', #8117, #10684, #4004, .T. ) ;
#12990=CIRCLE ( 'NONE', #13671, 11.98469917212512215 ) ;
#12991=DIRECTION ( 'NONE',  ( -0.5000000000000057732, 0.8660254037844352659, 0.000000000000000000 ) ) ;
#12995=VERTEX_POINT ( 'NONE', #15271 ) ;
#12996=DIRECTION ( 'NONE',  ( -0.5000000000000051070, 0.8660254037844359321, -0.000000000000000000 ) ) ;
#12998=CARTESIAN_POINT ( 'NONE',  ( 205.8264633344831225, 9.596613037118636669, -14.00000000000005507 ) ) ;
#13002=CIRCLE ( 'NONE', #20432, 11.94520687646042667 ) ;
#13005=EDGE_LOOP ( 'NONE', ( #2703, #10457, #17, #19373, #19266, #13484 ) ) ;
#13009=ORIENTED_EDGE ( 'NONE', *, *, #15881, .F. ) ;
#13011=LINE ( 'NONE', #9696, #12965 ) ;
#13021=CARTESIAN_POINT ( 'NONE',  ( 198.5374064076044078, -1.503684146350823703, -15.40190399002796440 ) ) ;
#13028=CARTESIAN_POINT ( 'NONE',  ( 208.4761278624580711, 5.007259451653140125, -14.00000000000005507 ) ) ;
#13029=EDGE_LOOP ( 'NONE', ( #6614, #11083, #17217, #15197 ) ) ;
#13030=ORIENTED_EDGE ( 'NONE', *, *, #13963, .F. ) ;
#13032=B_SPLINE_CURVE_WITH_KNOTS ( 'NONE', 3,
 ( #15005, #2257, #6906, #5306 ),
 .UNSPECIFIED., .F., .F.,
 ( 4, 4 ),
 ( 3.577803810849139650E-07, 0.0006730085724363164519 ),
 .UNSPECIFIED. ) ;
#13034=AXIS2_PLACEMENT_3D ( 'NONE', #4602, #4506, #1010 ) ;
#13035=CARTESIAN_POINT ( 'NONE',  ( 207.4098631234038521, 11.04183859327925354, -25.80036831778744144 ) ) ;
#13041=ADVANCED_FACE ( 'NONE', ( #16093 ), #3163, .T. ) ;
#13042=DIRECTION ( 'NONE',  ( -0.5000000000000051070, 0.8660254037844359321, -0.000000000000000000 ) ) ;
#13043=CARTESIAN_POINT ( 'NONE',  ( 205.0193973458067092, 9.661702533094931766, -25.81526893633797570 ) ) ;
#13044=EDGE_LOOP ( 'NONE', ( #10040, #6039, #8674, #8292 ) ) ;
#13049=EDGE_CURVE ( 'NONE', #16451, #184, #5519, .T. ) ;
#13051=VECTOR ( 'NONE', #13742, 1000.000000000000114 ) ;
#13054=ADVANCED_FACE ( 'NONE', ( #19058 ), #11204, .F. ) ;
#13060=DIRECTION ( 'NONE',  ( -0.5000000000000049960, 0.8660254037844357100, -0.000000000000000000 ) ) ;
#13063=DIRECTION ( 'NONE',  ( -0.5000000000000049960, 0.8660254037844357100, -0.000000000000000000 ) ) ;
#13069=CARTESIAN_POINT ( 'NONE',  ( 200.3972727712213668, 6.993117665730062882, -3.627429155984474907 ) ) ;
#13075=ORIENTED_EDGE ( 'NONE', *, *, #9615, .F. ) ;
#13079=CONICAL_SURFACE ( 'NONE', #9667, 10.85470691220533190, 0.8171114040043576665 ) ;
#13086=DIRECTION ( 'NONE',  ( 0.5000000000000054401, -0.8660254037844354880, 0.000000000000000000 ) ) ;
#13088=B_SPLINE_CURVE_WITH_KNOTS ( 'NONE', 3,
 ( #3484, #16733, #8238, #622 ),
 .UNSPECIFIED., .F., .F.,
 ( 4, 4 ),
 ( 8.130009260133085402E-07, 0.0008547987389031481238 ),
 .UNSPECIFIED. ) ;
#13093=CIRCLE ( 'NONE', #7319, 11.98469917212512215 ) ;
#13096=CIRCLE ( 'NONE', #10358, 12.47473710546057823 ) ;
#13100=CARTESIAN_POINT ( 'NONE',  ( 205.0662616026534693, 10.91332106064940888, -14.00000000000005507 ) ) ;
#13107=ORIENTED_EDGE ( 'NONE', *, *, #6581, .F. ) ;
#13115=CARTESIAN_POINT ( 'NONE',  ( 208.9187556984696812, 16.03699604507445287, -24.25943249057096907 ) ) ;
#13116=VERTEX_POINT ( 'NONE', #15783 ) ;
#13120=ORIENTED_EDGE ( 'NONE', *, *, #17701, .T. ) ;
#13122=AXIS2_PLACEMENT_3D ( 'NONE', #5158, #15370, #821 ) ;
#13126=CARTESIAN_POINT ( 'NONE',  ( 195.2863413965735333, 4.042320060767385037, -12.62152863576138806 ) ) ;
#13128=EDGE_CURVE ( 'NONE', #7006, #6033, #19406, .T. ) ;
#13129=AXIS2_PLACEMENT_3D ( 'NONE', #18924, #6286, #17441 ) ;
#13132=CARTESIAN_POINT ( 'NONE',  ( 215.4868200432858600, 15.17402258341379451, -8.415281845792092597 ) ) ;
#13136=CARTESIAN_POINT ( 'NONE',  ( 197.7335577521869823, 5.455221082446096936, -21.59012016402710188 ) ) ;
#13139=VECTOR ( 'NONE', #10796, 1000.000000000000227 ) ;
#13143=VERTEX_POINT ( 'NONE', #3243 ) ;
#13146=EDGE_CURVE ( 'NONE', #9708, #13417, #12699, .T. ) ;
#13147=VERTEX_POINT ( 'NONE', #20831 ) ;
#13148=DIRECTION ( 'NONE',  ( -0.8660254037844354880, -0.5000000000000055511, 0.000000000000000000 ) ) ;
#13149=CARTESIAN_POINT ( 'NONE',  ( 189.0671929290500088, 15.19036466668641872, -9.718744748712971671 ) ) ;
#13150=ADVANCED_FACE ( 'NONE', ( #4631 ), #4853, .T. ) ;
#13151=ORIENTED_EDGE ( 'NONE', *, *, #2027, .F. ) ;
#13153=ORIENTED_EDGE ( 'NONE', *, *, #13762, .T. ) ;
#13154=EDGE_CURVE ( 'NONE', #10151, #4077, #14617, .T. ) ;
#13158=CARTESIAN_POINT ( 'NONE',  ( 205.2117758015800462, 9.241723024529527208, -1.545471579934808215 ) ) ;
#13159=EDGE_CURVE ( 'NONE', #18887, #8757, #6980, .T. ) ;
#13161=CARTESIAN_POINT ( 'NONE',  ( 206.1888006519934891, 10.33685784671313002, -25.96516918080908454 ) ) ;
#13162=B_SPLINE_CURVE_WITH_KNOTS ( 'NONE', 3,
 ( #7679, #9262, #10978, #12470 ),
 .UNSPECIFIED., .F., .F.,
 ( 4, 4 ),
 ( 4.097547176954192966E-05, 0.0008949612097532494903 ),
 .UNSPECIFIED. ) ;
#13163=ORIENTED_EDGE ( 'NONE', *, *, #977, .F. ) ;
#13171=ORIENTED_EDGE ( 'NONE', *, *, #16022, .T. ) ;
#13183=EDGE_LOOP ( 'NONE', ( #6955, #9643, #7170, #17233 ) ) ;
#13192=EDGE_CURVE ( 'NONE', #19576, #13251, #6202, .T. ) ;
#13203=DIRECTION ( 'NONE',  ( 0.7739085681710397013, 0.4468163201617135760, 0.4487991802004502873 ) ) ;
#13204=DIRECTION ( 'NONE',  ( -0.8660254037844355990, -0.5000000000000055511, 0.000000000000000000 ) ) ;
#13205=CARTESIAN_POINT ( 'NONE',  ( 216.7433590455158878, 9.780347600644502037, -22.03054070023868860 ) ) ;
#13208=CARTESIAN_POINT ( 'NONE',  ( 215.5759555690916045, 8.333526798634666832, -24.58554911381534325 ) ) ;
#13210=ORIENTED_EDGE ( 'NONE', *, *, #5523, .F. ) ;
#13212=ORIENTED_EDGE ( 'NONE', *, *, #4998, .F. ) ;
#13213=LINE ( 'NONE', #17886, #17703 ) ;
#13217=CARTESIAN_POINT ( 'NONE',  ( 709.3577481411962253, -862.5451554485315455, -14.00000000000005507 ) ) ;
#13221=ORIENTED_EDGE ( 'NONE', *, *, #9485, .F. ) ;
#13225=LINE ( 'NONE', #17783, #2743 ) ;
#13228=ORIENTED_EDGE ( 'NONE', *, *, #20111, .F. ) ;
#13234=ORIENTED_EDGE ( 'NONE', *, *, #210, .T. ) ;
#13239=CARTESIAN_POINT ( 'NONE',  ( 216.1228831263525194, 15.89529313325283688, -12.59311507502024163 ) ) ;
#13240=AXIS2_PLACEMENT_3D ( 'NONE', #5444, #14924, #389 ) ;
#13241=AXIS2_PLACEMENT_3D ( 'NONE', #10941, #2787, #9228 ) ;
#13242=CARTESIAN_POINT ( 'NONE',  ( 208.0983737146324870, 5.661548828456886895, -14.00000000000005507 ) ) ;
#13245=VECTOR ( 'NONE', #20329, 1000.000000000000227 ) ;
#13246=B_SPLINE_CURVE_WITH_KNOTS ( 'NONE', 3,
 ( #11005, #9604, #16100, #5899 ),
 .UNSPECIFIED., .F., .F.,
 ( 4, 4 ),
 ( 5.484421174515580465E-05, 0.0009088299497278719708 ),
 .UNSPECIFIED. ) ;
#13248=VECTOR ( 'NONE', #10438, 1000.000000000000227 ) ;
#13250=EDGE_CURVE ( 'NONE', #5859, #3323, #12990, .T. ) ;
#13251=VERTEX_POINT ( 'NONE', #13926 ) ;
#13258=DIRECTION ( 'NONE',  ( 0.5000000000000052180, -0.8660254037844355990, -0.000000000000000000 ) ) ;
#13264=CARTESIAN_POINT ( 'NONE',  ( 214.9166615741016244, 8.725703323795450217, -24.01557619556987078 ) ) ;
#13267=CARTESIAN_POINT ( 'NONE',  ( 201.2663852398743529, 7.494899983462938842, -14.00000000000005507 ) ) ;
#13268=EDGE_CURVE ( 'NONE', #18827, #20929, #17415, .T. ) ;
#13269=ORIENTED_EDGE ( 'NONE', *, *, #18939, .F. ) ;
#13272=CARTESIAN_POINT ( 'NONE',  ( 197.7473131227538659, -1.187024626400782656, -12.53629070788332989 ) ) ;
#13283=ORIENTED_EDGE ( 'NONE', *, *, #20908, .T. ) ;
#13284=ORIENTED_EDGE ( 'NONE', *, *, #589, .T. ) ;
#13285=DIRECTION ( 'NONE',  ( 0.5547001962252345875, 0.000000000000000000, 0.8320502943378400573 ) ) ;
#13286=ORIENTED_EDGE ( 'NONE', *, *, #8874, .F. ) ;
#13289=CONICAL_SURFACE ( 'NONE', #11605, 10.85470691220533190, 0.8171114040043576665 ) ;
#13293=ORIENTED_EDGE ( 'NONE', *, *, #19246, .T. ) ;
#13300=VERTEX_POINT ( 'NONE', #10322 ) ;
#13302=FACE_OUTER_BOUND ( 'NONE', #4397, .T. ) ;
#13303=DIRECTION ( 'NONE',  ( 0.5000000000000049960, -0.8660254037844358210, 0.000000000000000000 ) ) ;
#13306=EDGE_CURVE ( 'NONE', #2200, #5521, #11533, .T. ) ;
#13307=EDGE_LOOP ( 'NONE', ( #19621, #7930, #736, #13356 ) ) ;
#13309=EDGE_CURVE ( 'NONE', #5971, #7973, #7884, .T. ) ;
#13311=CARTESIAN_POINT ( 'NONE',  ( 208.8107687779841228, 4.427644383670616079, -14.00000000000005507 ) ) ;
#13315=DIRECTION ( 'NONE',  ( 0.5000000000000051070, -0.8660254037844359321, 0.000000000000000000 ) ) ;
#13316=EDGE_CURVE ( 'NONE', #19592, #19576, #20394, .T. ) ;
#13321=VERTEX_POINT ( 'NONE', #14146 ) ;
#13325=ADVANCED_FACE ( 'NONE', ( #7432 ), #19980, .F. ) ;
#13332=CARTESIAN_POINT ( 'NONE',  ( 215.6983787324637376, 15.82721531135244675, -16.75125533358882279 ) ) ;
#13333=CARTESIAN_POINT ( 'NONE',  ( 205.8534188064671469, 2.720217581527302642, -2.669358488461094581 ) ) ;
#13335=VERTEX_POINT ( 'NONE', #1197 ) ;
#13338=LINE ( 'NONE', #17042, #17146 ) ;
#13347=DIRECTION ( 'NONE',  ( -0.8660254037844355990, -0.5000000000000054401, -7.092004947830981940E-15 ) ) ;
#13351=CARTESIAN_POINT ( 'NONE',  ( 205.0042238655992719, 9.652942120212628652, -25.96516918080906677 ) ) ;
#13352=CARTESIAN_POINT ( 'NONE',  ( 208.4761278624580711, 5.007259451653140125, -14.00000000000005507 ) ) ;
#13353=ORIENTED_EDGE ( 'NONE', *, *, #6938, .T. ) ;
#13354=ORIENTED_EDGE ( 'NONE', *, *, #3317, .T. ) ;
#13356=ORIENTED_EDGE ( 'NONE', *, *, #4813, .F. ) ;
#13358=CARTESIAN_POINT ( 'NONE',  ( 210.5941221282246545, 5.457263920492195552, -2.233628351993232730 ) ) ;
#13370=CARTESIAN_POINT ( 'NONE',  ( 213.4541640218532166, 5.845417697364395870, -14.00000000000005507 ) ) ;
#13371=DIRECTION ( 'NONE',  ( -0.5000000000000049960, 0.8660254037844357100, -0.000000000000000000 ) ) ;
#13379=VERTEX_POINT ( 'NONE', #1100 ) ;
#13380=VERTEX_POINT ( 'NONE', #19113 ) ;
#13381=B_SPLINE_CURVE_WITH_KNOTS ( 'NONE', 3,
 ( #20790, #11152, #16052, #1513 ),
 .UNSPECIFIED., .F., .F.,
 ( 4, 4 ),
 ( 2.916652381017237348E-07, 0.0006729424572952378593 ),
 .UNSPECIFIED. ) ;
#13382=ORIENTED_EDGE ( 'NONE', *, *, #2171, .T. ) ;
#13385=CARTESIAN_POINT ( 'NONE',  ( 216.2725394319739110, 15.91768827161142674, -14.00000000000005507 ) ) ;
#13386=ORIENTED_EDGE ( 'NONE', *, *, #14603, .T. ) ;
#13388=EDGE_CURVE ( 'NONE', #13569, #2452, #4788, .T. ) ;
#13390=CYLINDRICAL_SURFACE ( 'NONE', #17220, 12.47473710546057646 ) ;
#13392=CARTESIAN_POINT ( 'NONE',  ( 196.2730226335446844, 4.434970834353566538, -8.544894389632862186 ) ) ;
#13398=LINE ( 'NONE', #5115, #1967 ) ;
#13399=ORIENTED_EDGE ( 'NONE', *, *, #16651, .T. ) ;
#13401=DIRECTION ( 'NONE',  ( 0.8601696498176548689, 0.4966191788709768407, -0.1160929141252376451 ) ) ;
#13403=CARTESIAN_POINT ( 'NONE',  ( 205.8264633344831225, 9.596613037118636669, -14.00000000000005507 ) ) ;
#13405=EDGE_CURVE ( 'NONE', #13379, #17056, #1411, .T. ) ;
#13408=FACE_OUTER_BOUND ( 'NONE', #16768, .T. ) ;
#13409=DIRECTION ( 'NONE',  ( -0.8660254037844355990, -0.5000000000000055511, 0.000000000000000000 ) ) ;
#13413=EDGE_CURVE ( 'NONE', #17484, #2297, #3832, .T. ) ;
#13414=CARTESIAN_POINT ( 'NONE',  ( 206.1888006519934891, 10.33685784671313002, -25.96516918080908454 ) ) ;
#13417=VERTEX_POINT ( 'NONE', #6461 ) ;
#13420=VECTOR ( 'NONE', #3833, 1000.000000000000000 ) ;
#13423=ORIENTED_EDGE ( 'NONE', *, *, #12001, .T. ) ;
#13427=CARTESIAN_POINT ( 'NONE',  ( 212.8611117457045907, 7.023710210201398851, -25.12838443884023576 ) ) ;
#13428=AXIS2_PLACEMENT_3D ( 'NONE', #7050, #19559, #10221 ) ;
#13433=ORIENTED_EDGE ( 'NONE', *, *, #13146, .T. ) ;
#13439=EDGE_LOOP ( 'NONE', ( #16636, #14211, #2226, #10353 ) ) ;
#13444=DIRECTION ( 'NONE',  ( 0.6634139481689433904, 0.3830222215594973889, 0.6427876096865291489 ) ) ;
#13448=VERTEX_POINT ( 'NONE', #17626 ) ;
#13449=CARTESIAN_POINT ( 'NONE',  ( 219.9079348888217567, 10.83459622500478048, -11.01983352639526714 ) ) ;
#13451=CARTESIAN_POINT ( 'NONE',  ( 208.4761278624580711, 5.007259451653140125, -14.00000000000005507 ) ) ;
#13453=CARTESIAN_POINT ( 'NONE',  ( 212.8527399996651752, 6.761277556564890823, -3.125199447383528284 ) ) ;
#13456=DIRECTION ( 'NONE',  ( -0.7951984747223579397, -0.4591080534401397184, 0.3960797660391670583 ) ) ;
#13458=ORIENTED_EDGE ( 'NONE', *, *, #2575, .F. ) ;
#13463=ORIENTED_EDGE ( 'NONE', *, *, #6551, .F. ) ;
#13464=CARTESIAN_POINT ( 'NONE',  ( 218.5272241891094325, 10.03744253085286964, -18.09983247376310089 ) ) ;
#13465=DIRECTION ( 'NONE',  ( -0.7499999999999953371, -0.4330127018922228510, 0.5000000000000038858 ) ) ;
#13478=DIRECTION ( 'NONE',  ( -0.8660254037844355990, -0.5000000000000055511, 0.000000000000000000 ) ) ;
#13480=ORIENTED_EDGE ( 'NONE', *, *, #19079, .T. ) ;
#13481=CARTESIAN_POINT ( 'NONE',  ( 203.1555906521724637, 1.162625770417896609, -2.579136038830115218 ) ) ;
#13483=CARTESIAN_POINT ( 'NONE',  ( 207.3371157680689407, 10.99983788809380236, -1.383673999417951439 ) ) ;
#13484=ORIENTED_EDGE ( 'NONE', *, *, #14119, .T. ) ;
#13487=EDGE_CURVE ( 'NONE', #14131, #17716, #1511, .T. ) ;
#13490=VECTOR ( 'NONE', #10688, 1000.000000000000114 ) ;
#13494=ORIENTED_EDGE ( 'NONE', *, *, #2278, .T. ) ;
#13496=ORIENTED_EDGE ( 'NONE', *, *, #12987, .F. ) ;
#13499=CARTESIAN_POINT ( 'NONE',  ( 198.4028805101389992, 5.310605495132000975, -23.06309126349794170 ) ) ;
#13502=EDGE_CURVE ( 'NONE', #3214, #1853, #4985, .T. ) ;
#13503=VECTOR ( 'NONE', #4368, 1000.000000000000227 ) ;
#13506=LINE ( 'NONE', #8719, #18217 ) ;
#13507=CARTESIAN_POINT ( 'NONE',  ( 199.2144802262915846, 21.04890371929339921, -14.00000000000005507 ) ) ;
#13508=ADVANCED_FACE ( 'NONE', ( #7959 ), #6529, .T. ) ;
#13509=FACE_OUTER_BOUND ( 'NONE', #4408, .T. ) ;
#13510=ADVANCED_FACE ( 'NONE', ( #17736 ), #1145, .T. ) ;
#13513=EDGE_LOOP ( 'NONE', ( #1987, #19193, #18329, #20637 ) ) ;
#13514=ORIENTED_EDGE ( 'NONE', *, *, #19711, .T. ) ;
#13519=ORIENTED_EDGE ( 'NONE', *, *, #20501, .T. ) ;
#13521=DIRECTION ( 'NONE',  ( -0.8660254037844355990, -0.5000000000000055511, 0.000000000000000000 ) ) ;
#13522=ORIENTED_EDGE ( 'NONE', *, *, #6956, .T. ) ;
#13526=CIRCLE ( 'NONE', #1680, 11.98469917212512215 ) ;
#13537=VERTEX_POINT ( 'NONE', #10060 ) ;
#13538=ORIENTED_EDGE ( 'NONE', *, *, #4468, .T. ) ;
#13539=CYLINDRICAL_SURFACE ( 'NONE', #4081, 12.47473710546057646 ) ;
#13542=ORIENTED_EDGE ( 'NONE', *, *, #15291, .F. ) ;
#13543=EDGE_LOOP ( 'NONE', ( #19994, #18755, #5582, #5420 ) ) ;
#13546=CARTESIAN_POINT ( 'NONE',  ( 215.3856909933734300, 6.960585314318631589, -14.00000000000005329 ) ) ;
#13548=CIRCLE ( 'NONE', #6748, 11.94520687646042667 ) ;
#13559=DIRECTION ( 'NONE',  ( -0.8660254037844354880, -0.5000000000000055511, 0.000000000000000000 ) ) ;
#13560=EDGE_CURVE ( 'NONE', #7157, #12427, #10609, .T. ) ;
#13564=ORIENTED_EDGE ( 'NONE', *, *, #3394, .F. ) ;
#13569=VERTEX_POINT ( 'NONE', #2031 ) ;
#13570=CARTESIAN_POINT ( 'NONE',  ( 207.8344881237125890, 4.636808575765666518, -26.45271578590683248 ) ) ;
#13571=PLANE ( 'NONE',  #14109 ) ;
#13574=ADVANCED_FACE ( 'NONE', ( #16549 ), #12329, .T. ) ;
#13575=ORIENTED_EDGE ( 'NONE', *, *, #4409, .F. ) ;
#13577=VECTOR ( 'NONE', #19310, 1000.000000000000000 ) ;
#13580=CONICAL_SURFACE ( 'NONE', #20674, 10.85470691220533190, 0.8171114040043576665 ) ;
#13582=PLANE ( 'NONE',  #13731 ) ;
#13583=EDGE_CURVE ( 'NONE', #18388, #12727, #11997, .T. ) ;
#13592=EDGE_LOOP ( 'NONE', ( #14001, #10329, #7782, #3693 ) ) ;
#13596=ORIENTED_EDGE ( 'NONE', *, *, #2296, .T. ) ;
#13597=CARTESIAN_POINT ( 'NONE',  ( 198.5498304622664989, 5.926496351342651181, -5.407152407593843968 ) ) ;
#13598=VECTOR ( 'NONE', #20691, 1000.000000000000114 ) ;
#13603=SHAPE_DEFINITION_REPRESENTATION ( #15708, #9759 ) ;
#13607=DIRECTION ( 'NONE',  ( -0.5943026915289656431, -0.3431208189343725179, -0.7273736415730450711 ) ) ;
#13611=CONICAL_SURFACE ( 'NONE', #8870, 13.07248899748297433, 0.6693469023067423196 ) ;
#13614=CYLINDRICAL_SURFACE ( 'NONE', #2448, 12.47473710546057646 ) ;
#13615=B_SPLINE_CURVE_WITH_KNOTS ( 'NONE', 3,
 ( #18773, #9001, #1177, #855 ),
 .UNSPECIFIED., .F., .F.,
 ( 4, 4 ),
 ( 3.603418170223495296E-07, 0.0008543460798012778587 ),
 .UNSPECIFIED. ) ;
#13620=CARTESIAN_POINT ( 'NONE',  ( 203.3297164780629487, 6.518256075426767313E-05, -14.00000000000005507 ) ) ;
#13625=ORIENTED_EDGE ( 'NONE', *, *, #17867, .F. ) ;
#13632=CARTESIAN_POINT ( 'NONE',  ( 198.2252501544971324, -1.168701404234412600, -16.84132998195068964 ) ) ;
#13639=CARTESIAN_POINT ( 'NONE',  ( 213.5401130648333492, 14.58114004716331280, -6.286464976499002155 ) ) ;
#13647=ORIENTED_EDGE ( 'NONE', *, *, #15861, .T. ) ;
#13649=CARTESIAN_POINT ( 'NONE',  ( 203.4540983502001836, 1.592568494036425530, -24.50020013040629863 ) ) ;
#13653=CARTESIAN_POINT ( 'NONE',  ( 217.3629815419766942, 9.365266725128718051, -20.52105855319946670 ) ) ;
#13654=ORIENTED_EDGE ( 'NONE', *, *, #6639, .F. ) ;
#13656=LINE ( 'NONE', #5464, #4654 ) ;
#13658=CONICAL_SURFACE ( 'NONE', #5502, 13.07248899748297433, 0.6693469023067423196 ) ;
#13659=ADVANCED_FACE ( 'NONE', ( #19820 ), #6994, .F. ) ;
#13660=ADVANCED_FACE ( 'NONE', ( #3926 ), #20144, .T. ) ;
#13662=DIRECTION ( 'NONE',  ( -0.5000000000000051070, 0.8660254037844359321, -0.000000000000000000 ) ) ;
#13670=ORIENTED_EDGE ( 'NONE', *, *, #2278, .F. ) ;
#13671=AXIS2_PLACEMENT_3D ( 'NONE', #17203, #5945, #1304 ) ;
#13673=ORIENTED_EDGE ( 'NONE', *, *, #1997, .F. ) ;
#13680=EDGE_LOOP ( 'NONE', ( #5061, #20685, #17380, #12293 ) ) ;
#13681=DIRECTION ( 'NONE',  ( 0.5000000000000053291, -0.8660254037844355990, -2.220446049250312588E-16 ) ) ;
#13685=VECTOR ( 'NONE', #9222, 1000.000000000000000 ) ;
#13686=DIRECTION ( 'NONE',  ( -0.8528685319524408337, -0.4924038765061092282, -0.1736481776669271115 ) ) ;
#13692=EDGE_CURVE ( 'NONE', #12370, #18332, #17745, .T. ) ;
#13693=VERTEX_POINT ( 'NONE', #2770 ) ;
#13697=ORIENTED_EDGE ( 'NONE', *, *, #10450, .T. ) ;
#13702=EDGE_CURVE ( 'NONE', #15950, #1927, #10700, .T. ) ;
#13708=DIRECTION ( 'NONE',  ( -0.8660254037844357100, -0.5000000000000051070, 0.000000000000000000 ) ) ;
#13710=CARTESIAN_POINT ( 'NONE',  ( 201.5617312735136579, 7.665418095488669259, -2.488895219275796933 ) ) ;
#13712=DIRECTION ( 'NONE',  ( 0.5000000000000051070, -0.8660254037844359321, 0.000000000000000000 ) ) ;
#13714=EDGE_CURVE ( 'NONE', #5663, #19244, #14126, .T. ) ;
#13716=DIRECTION ( 'NONE',  ( 0.8660254037844355990, 0.5000000000000054401, -1.599177586275613688E-14 ) ) ;
#13717=ORIENTED_EDGE ( 'NONE', *, *, #14844, .F. ) ;
#13718=LINE ( 'NONE', #2369, #691 ) ;
#13719=CARTESIAN_POINT ( 'NONE',  ( 205.5965122587965084, 9.994899983462953941, -14.00000000000005507 ) ) ;
#13721=PLANE ( 'NONE',  #19236 ) ;
#13723=ORIENTED_EDGE ( 'NONE', *, *, #14740, .T. ) ;
#13728=CARTESIAN_POINT ( 'NONE',  ( 219.1254566829535975, 10.64043144601880897, -15.41218500610179198 ) ) ;
#13730=DIRECTION ( 'NONE',  ( -0.8660254037844357100, -0.5000000000000049960, 0.000000000000000000 ) ) ;
#13731=AXIS2_PLACEMENT_3D ( 'NONE', #17930, #14871, #11670 ) ;
#13736=DIRECTION ( 'NONE',  ( 0.8660254037844355990, 0.5000000000000054401, 0.000000000000000000 ) ) ;
#13739=CARTESIAN_POINT ( 'NONE',  ( 205.9193846489986015, 10.18131044486001535, -16.32385667531026741 ) ) ;
#13741=CARTESIAN_POINT ( 'NONE',  ( 196.9187795697884269, 4.984808679508447860, -7.425127016398286983 ) ) ;
#13742=DIRECTION ( 'NONE',  ( 0.5000000000000055511, -0.8660254037844353769, 2.775557561562890735E-17 ) ) ;
#13743=VECTOR ( 'NONE', #16033, 1000.000000000000000 ) ;
#13745=ORIENTED_EDGE ( 'NONE', *, *, #11961, .F. ) ;
#13746=AXIS2_PLACEMENT_3D ( 'NONE', #905, #3866, #13736 ) ;
#13751=ORIENTED_EDGE ( 'NONE', *, *, #4342, .T. ) ;
#13757=CARTESIAN_POINT ( 'NONE',  ( 199.4075733045063146, 6.421714412205289157, -4.379064819896086647 ) ) ;
#13761=PLANE ( 'NONE',  #325 ) ;
#13762=EDGE_CURVE ( 'NONE', #9756, #6104, #1830, .T. ) ;
#13763=CARTESIAN_POINT ( 'NONE',  ( 209.4067366129695529, 3.387278741123676440, -14.00000000000005507 ) ) ;
#13769=ORIENTED_EDGE ( 'NONE', *, *, #14862, .F. ) ;
#13773=CARTESIAN_POINT ( 'NONE',  ( 198.5809828321035013, -0.9633190470588108845, -9.788772202513250420 ) ) ;
#13778=VECTOR ( 'NONE', #11611, 1000.000000000000227 ) ;
#13779=EDGE_CURVE ( 'NONE', #2710, #16780, #2852, .T. ) ;
#13781=CARTESIAN_POINT ( 'NONE',  ( 198.8157711536554189, -0.5701500946419610916, -8.415281845791808379 ) ) ;
#13783=ORIENTED_EDGE ( 'NONE', *, *, #3916, .T. ) ;
#13785=CARTESIAN_POINT ( 'NONE',  ( 193.6336827526812101, 7.212155065240265728, -15.39542905462715083 ) ) ;
#13786=CARTESIAN_POINT ( 'NONE',  ( 213.9922241104001444, 18.96616439842760471, -12.64773574313060678 ) ) ;
#13790=CARTESIAN_POINT ( 'NONE',  ( 214.7465214175448125, 15.27766023435388298, -8.669480444820855780 ) ) ;
#13791=DIRECTION ( 'NONE',  ( -0.7743856023693594937, 0.000000000000000000, 0.6327139470906613106 ) ) ;
#13795=ORIENTED_EDGE ( 'NONE', *, *, #20040, .T. ) ;
#13797=DIRECTION ( 'NONE',  ( -0.9679941405060890069, 0.000000000000000000, 0.2509727952306343712 ) ) ;
#13805=EDGE_CURVE ( 'NONE', #18096, #9213, #7736, .T. ) ;
#13807=EDGE_CURVE ( 'NONE', #7763, #10335, #2454, .T. ) ;
#13811=ORIENTED_EDGE ( 'NONE', *, *, #20234, .F. ) ;
#13817=ADVANCED_FACE ( 'NONE', ( #2872 ), #20661, .F. ) ;
#13820=CARTESIAN_POINT ( 'NONE',  ( 199.5603494194345444, -0.9130877231049959741, -19.34736286182874565 ) ) ;
#13828=EDGE_CURVE ( 'NONE', #9199, #14589, #16327, .T. ) ;
#13834=ORIENTED_EDGE ( 'NONE', *, *, #11700, .F. ) ;
#13837=EDGE_CURVE ( 'NONE', #18324, #7529, #4562, .T. ) ;
#13840=CARTESIAN_POINT ( 'NONE',  ( 208.4761278624580711, 5.007259451653140125, -14.00000000000005507 ) ) ;
#13848=DIRECTION ( 'NONE',  ( -0.4330127018922213522, -0.2500000000000047740, -0.8660254037844362651 ) ) ;
#13850=CARTESIAN_POINT ( 'NONE',  ( 206.7320635740233854, 14.77450875839051925, -25.34310559273333396 ) ) ;
#13851=AXIS2_PLACEMENT_3D ( 'NONE', #5724, #12221, #18687 ) ;
#13853=ORIENTED_EDGE ( 'NONE', *, *, #6378, .F. ) ;
#13864=FACE_OUTER_BOUND ( 'NONE', #14291, .T. ) ;
#13871=CARTESIAN_POINT ( 'NONE',  ( 209.2023654653594349, 5.168939075417601003, -1.722272971484202220 ) ) ;
#13876=EDGE_LOOP ( 'NONE', ( #13382, #10935, #4097, #2599 ) ) ;
#13877=CARTESIAN_POINT ( 'NONE',  ( 208.0154570403102241, 11.39147840422473479, -11.03569519926165654 ) ) ;
#13881=FACE_OUTER_BOUND ( 'NONE', #19186, .T. ) ;
#13888=EDGE_CURVE ( 'NONE', #17291, #20129, #14433, .T. ) ;
#13891=CARTESIAN_POINT ( 'NONE',  ( 214.0593366061550569, 19.00491181591769418, -13.97827067520052324 ) ) ;
#13903=AXIS2_PLACEMENT_3D ( 'NONE', #20253, #18361, #10605 ) ;
#13906=FACE_OUTER_BOUND ( 'NONE', #9314, .T. ) ;
#13914=DIRECTION ( 'NONE',  ( -0.8404609622712050365, 0.000000000000000000, -0.5418720982834971389 ) ) ;
#13919=FACE_OUTER_BOUND ( 'NONE', #13592, .T. ) ;
#13922=B_SPLINE_CURVE_WITH_KNOTS ( 'NONE', 3,
 ( #12984, #16367, #6279, #3217 ),
 .UNSPECIFIED., .F., .F.,
 ( 4, 4 ),
 ( 7.831744291011048613E-05, 0.0007509682349631222791 ),
 .UNSPECIFIED. ) ;
#13926=CARTESIAN_POINT ( 'NONE',  ( 216.3355731942785951, 15.66405044361498788, -16.89203719259520753 ) ) ;
#13928=CARTESIAN_POINT ( 'NONE',  ( 205.5374615299400602, 3.053005801749057113, -2.216907231065453399 ) ) ;
#13929=ORIENTED_EDGE ( 'NONE', *, *, #17019, .F. ) ;
#13930=CIRCLE ( 'NONE', #4774, 12.47473710546057823 ) ;
#13933=LINE ( 'NONE', #20697, #9830 ) ;
#13937=DIRECTION ( 'NONE',  ( -0.8660254037844358210, -0.5000000000000049960, 0.000000000000000000 ) ) ;
#13943=VERTEX_POINT ( 'NONE', #13043 ) ;
#13945=EDGE_CURVE ( 'NONE', #3166, #9370, #19089, .T. ) ;
#13950=CARTESIAN_POINT ( 'NONE',  ( 195.7860920451057325, 4.153841328041666614, -9.848357292554023701 ) ) ;
#13951=EDGE_CURVE ( 'NONE', #5368, #14969, #896, .T. ) ;
#13960=CARTESIAN_POINT ( 'NONE',  ( 215.6932043811731603, 15.82422789824195242, -11.22353489230414958 ) ) ;
#13961=VECTOR ( 'NONE', #8066, 1000.000000000000000 ) ;
#13963=EDGE_CURVE ( 'NONE', #10440, #8359, #16459, .T. ) ;
#13966=ORIENTED_EDGE ( 'NONE', *, *, #8206, .T. ) ;
#13971=ORIENTED_EDGE ( 'NONE', *, *, #15986, .T. ) ;
#13973=CARTESIAN_POINT ( 'NONE',  ( 709.3577481411962253, -862.5451554485315455, -14.00000000000005507 ) ) ;
#13983=CIRCLE ( 'NONE', #8543, 11.98469917212512215 ) ;
#13986=CARTESIAN_POINT ( 'NONE',  ( 215.2753377405919650, 15.22894589946059440, -19.53076827296978024 ) ) ;
#13988=ORIENTED_EDGE ( 'NONE', *, *, #20871, .F. ) ;
#13989=EDGE_LOOP ( 'NONE', ( #5097, #7776, #6929, #6730 ) ) ;
#13990=DIRECTION ( 'NONE',  ( 0.000000000000000000, 0.000000000000000000, -1.000000000000000000 ) ) ;
#13991=CARTESIAN_POINT ( 'NONE',  ( 205.2286857969292839, 9.782535276688834713, -12.71431551095683332 ) ) ;
#13996=DIRECTION ( 'NONE',  ( 0.8660254037844357100, 0.5000000000000052180, 0.000000000000000000 ) ) ;
#14000=ORIENTED_EDGE ( 'NONE', *, *, #1720, .T. ) ;
#14001=ORIENTED_EDGE ( 'NONE', *, *, #13306, .T. ) ;
#14010=CARTESIAN_POINT ( 'NONE',  ( 190.9472490432335690, 16.27581557030192982, -22.03054070023845767 ) ) ;
#14012=VECTOR ( 'NONE', #230, 1000.000000000000227 ) ;
#14013=ORIENTED_EDGE ( 'NONE', *, *, #19632, .F. ) ;
#14017=ORIENTED_EDGE ( 'NONE', *, *, #7090, .F. ) ;
#14027=CARTESIAN_POINT ( 'NONE',  ( 208.1960812450810465, 4.072754371081482638, -2.187257959407754804 ) ) ;
#14033=DIRECTION ( 'NONE',  ( -0.8660254037844357100, -0.5000000000000051070, 0.000000000000000000 ) ) ;
#14035=ADVANCED_FACE ( 'NONE', ( #6866 ), #14791, .T. ) ;
#14037=DIRECTION ( 'NONE',  ( 0.8660254037844352659, 0.5000000000000056621, 0.000000000000000000 ) ) ;
#14040=VECTOR ( 'NONE', #9408, 1000.000000000000227 ) ;
#14041=CARTESIAN_POINT ( 'NONE',  ( 212.7675431533135679, 7.484909225033065994, -2.551678190571531335 ) ) ;
#14043=CYLINDRICAL_SURFACE ( 'NONE', #18679, 12.47473710546057646 ) ;
#14050=CARTESIAN_POINT ( 'NONE',  ( 197.7441788599589074, -1.188834193869147571, -15.43274561385865873 ) ) ;
#14053=B_SPLINE_CURVE_WITH_KNOTS ( 'NONE', 3,
 ( #20451, #1174, #7623, #7725 ),
 .UNSPECIFIED., .F., .F.,
 ( 4, 4 ),
 ( 3.577803810398533474E-07, 0.0006730085724280226306 ),
 .UNSPECIFIED. ) ;
#14056=CIRCLE ( 'NONE', #12700, 11.98469917212512215 ) ;
#14062=CYLINDRICAL_SURFACE ( 'NONE', #2974, 12.47473710546057646 ) ;
#14064=LINE ( 'NONE', #2509, #4480 ) ;
#14069=ORIENTED_EDGE ( 'NONE', *, *, #15528, .F. ) ;
#14071=EDGE_CURVE ( 'NONE', #15363, #15277, #7980, .T. ) ;
#14075=CARTESIAN_POINT ( 'NONE',  ( 207.0325450024345457, 14.94799179197019789, -1.381056684022670344 ) ) ;
#14076=CARTESIAN_POINT ( 'NONE',  ( 207.3877668936371492, 11.02908132907535332, -2.195132782454303655 ) ) ;
#14077=CARTESIAN_POINT ( 'NONE',  ( 208.3673372177917429, 15.71863443681889549, -1.942038651984890674 ) ) ;
#14079=DIRECTION ( 'NONE',  ( 0.5000000000000051070, -0.8660254037844359321, 0.000000000000000000 ) ) ;
#14082=ORIENTED_EDGE ( 'NONE', *, *, #17147, .F. ) ;
#14085=AXIS2_PLACEMENT_3D ( 'NONE', #9847, #8368, #9945 ) ;
#14086=DIRECTION ( 'NONE',  ( -0.5943026915289658652, -0.3431208189343721848, -0.7273736415730450711 ) ) ;
#14088=DIRECTION ( 'NONE',  ( 0.8660254037844355990, 0.5000000000000054401, 0.000000000000000000 ) ) ;
#14089=AXIS2_PLACEMENT_3D ( 'NONE', #17831, #6457, #16343 ) ;
#14095=CARTESIAN_POINT ( 'NONE',  ( 195.4946457851292507, 4.162584655573419390, -16.75125533358848884 ) ) ;
#14097=LINE ( 'NONE', #13991, #15295 ) ;
#14104=AXIS2_PLACEMENT_3D ( 'NONE', #11298, #8092, #15984 ) ;
#14108=ORIENTED_EDGE ( 'NONE', *, *, #14345, .T. ) ;
#14109=AXIS2_PLACEMENT_3D ( 'NONE', #16639, #15075, #20127 ) ;
#14111=ORIENTED_EDGE ( 'NONE', *, *, #13502, .T. ) ;
#14113=EDGE_CURVE ( 'NONE', #2143, #18516, #8993, .T. ) ;
#14119=EDGE_CURVE ( 'NONE', #14158, #15392, #5478, .T. ) ;
#14126=LINE ( 'NONE', #9211, #9588 ) ;
#14131=VERTEX_POINT ( 'NONE', #3794 ) ;
#14132=ORIENTED_EDGE ( 'NONE', *, *, #13702, .T. ) ;
#14135=ADVANCED_FACE ( 'NONE', ( #10245 ), #16736, .F. ) ;
#14140=VECTOR ( 'NONE', #19349, 1000.000000000000227 ) ;
#14141=CARTESIAN_POINT ( 'NONE',  ( 202.2312820113153862, 1.144182166681870561, -23.86786078788932741 ) ) ;
#14146=CARTESIAN_POINT ( 'NONE',  ( 216.3417993343409194, 15.66764510725598214, -11.13829696442610029 ) ) ;
#14147=DIRECTION ( 'NONE',  ( -0.5000000000000051070, 0.8660254037844359321, -0.000000000000000000 ) ) ;
#14153=VECTOR ( 'NONE', #14640, 1000.000000000000114 ) ;
#14155=DIRECTION ( 'NONE',  ( -0.6958540455341998276, 0.000000000000000000, -0.7181832268395633712 ) ) ;
#14157=VECTOR ( 'NONE', #7573, 1000.000000000000227 ) ;
#14158=VERTEX_POINT ( 'NONE', #17367 ) ;
#14159=ORIENTED_EDGE ( 'NONE', *, *, #3165, .F. ) ;
#14166=DIRECTION ( 'NONE',  ( -0.8660254037844355990, -0.5000000000000054401, -1.779954182985030830E-14 ) ) ;
#14169=VECTOR ( 'NONE', #20855, 1000.000000000000227 ) ;
#14172=EDGE_CURVE ( 'NONE', #17905, #13143, #18158, .T. ) ;
#14175=FACE_OUTER_BOUND ( 'NONE', #5000, .T. ) ;
#14176=CARTESIAN_POINT ( 'NONE',  ( 197.9670180026625417, -1.060177954843255499, -16.89203719259486647 ) ) ;
#14177=ORIENTED_EDGE ( 'NONE', *, *, #6646, .T. ) ;
#14185=VECTOR ( 'NONE', #858, 1000.000000000000114 ) ;
#14189=CARTESIAN_POINT ( 'NONE',  ( 209.8373868153248623, 12.26636014609055891, -2.844109184787622535 ) ) ;
#14197=CARTESIAN_POINT ( 'NONE',  ( 211.0762420533076806, 12.80459687405399549, -3.334988897836945743 ) ) ;
#14199=DIRECTION ( 'NONE',  ( 0.5000000000000054401, -0.8660254037844354880, 0.000000000000000000 ) ) ;
#14206=PLANE ( 'NONE',  #7459 ) ;
#14211=ORIENTED_EDGE ( 'NONE', *, *, #5437, .T. ) ;
#14213=DIRECTION ( 'NONE',  ( 0.5000000000000049960, -0.8660254037844357100, 0.000000000000000000 ) ) ;
#14220=EDGE_CURVE ( 'NONE', #2011, #10374, #20216, .T. ) ;
#14221=DIRECTION ( 'NONE',  ( -0.5000000000000049960, 0.8660254037844358210, -0.000000000000000000 ) ) ;
#14225=LINE ( 'NONE', #2661, #2445 ) ;
#14230=CARTESIAN_POINT ( 'NONE',  ( 215.6527207509367088, 8.377847197037317173, -3.480441514389753799 ) ) ;
#14237=EDGE_CURVE ( 'NONE', #3665, #17033, #15689, .T. ) ;
#14240=CIRCLE ( 'NONE', #19615, 11.98469917212512215 ) ;
#14242=B_SPLINE_CURVE_WITH_KNOTS ( 'NONE', 3,
 ( #19648, #5125, #13728, #2381 ),
 .UNSPECIFIED., .F., .F.,
 ( 4, 4 ),
 ( 5.538124335884803249E-06, 0.0008595238623188111412 ),
 .UNSPECIFIED. ) ;
#14250=LINE ( 'NONE', #12335, #8823 ) ;
#14254=CYLINDRICAL_SURFACE ( 'NONE', #7524, 12.47473710546057646 ) ;
#14257=CARTESIAN_POINT ( 'NONE',  ( 209.8762589913676777, 12.46581291157635540, -14.99881147502670586 ) ) ;
#14262=CARTESIAN_POINT ( 'NONE',  ( 195.0522846737218288, 8.031185266226035679, -5.585956497639847029 ) ) ;
#14263=FACE_OUTER_BOUND ( 'NONE', #1674, .T. ) ;
#14275=DIRECTION ( 'NONE',  ( 0.8660254037844352659, 0.5000000000000056621, 0.000000000000000000 ) ) ;
#14276=AXIS2_PLACEMENT_3D ( 'NONE', #9949, #13371, #16657 ) ;
#14281=EDGE_LOOP ( 'NONE', ( #20244, #5532, #8844, #20307, #3683, #9462 ) ) ;
#14287=ORIENTED_EDGE ( 'NONE', *, *, #12418, .F. ) ;
#14291=EDGE_LOOP ( 'NONE', ( #971, #11377, #12882, #18253 ) ) ;
#14292=PLANE ( 'NONE',  #16303 ) ;
#14295=VECTOR ( 'NONE', #20387, 1000.000000000000227 ) ;
#14296=AXIS2_PLACEMENT_3D ( 'NONE', #13403, #15430, #10298 ) ;
#14297=DIRECTION ( 'NONE',  ( 0.8660254037844355990, 0.5000000000000054401, 4.449885457462577074E-15 ) ) ;
#14298=EDGE_CURVE ( 'NONE', #12209, #11821, #15884, .T. ) ;
#14299=CARTESIAN_POINT ( 'NONE',  ( 214.4612834781239314, 14.93596812906266180, -20.67833249884127866 ) ) ;
#14301=CARTESIAN_POINT ( 'NONE',  ( 211.8034485311565049, 13.57847631115287435, -23.60546391700164648 ) ) ;
#14302=CARTESIAN_POINT ( 'NONE',  ( 199.2144802262915846, 21.04890371929339921, -14.00000000000005507 ) ) ;
#14311=DIRECTION ( 'NONE',  ( 0.9987303135603810000, 0.000000000000000000, 0.05037619254750287656 ) ) ;
#14314=ORIENTED_EDGE ( 'NONE', *, *, #9374, .T. ) ;
#14315=ORIENTED_EDGE ( 'NONE', *, *, #4847, .T. ) ;
#14316=DIRECTION ( 'NONE',  ( -0.5000000000000163203, -0.8660254037844291597, 1.060575238724920473E-16 ) ) ;
#14327=DIRECTION ( 'NONE',  ( 0.3430151393149034611, 0.1980398830195791438, -0.9182161068802751069 ) ) ;
#14337=VECTOR ( 'NONE', #6966, 1000.000000000000114 ) ;
#14340=CIRCLE ( 'NONE', #11606, 11.94520687646042667 ) ;
#14345=EDGE_CURVE ( 'NONE', #9708, #12385, #15804, .T. ) ;
#14346=CARTESIAN_POINT ( 'NONE',  ( 203.0246517772566506, 23.22871929987775630, -14.00000000000005507 ) ) ;
#14351=DIRECTION ( 'NONE',  ( 0.5000000000000054401, -0.8660254037844354880, -2.081668171172167774E-16 ) ) ;
#14353=VECTOR ( 'NONE', #2971, 1000.000000000000000 ) ;
#14356=EDGE_CURVE ( 'NONE', #20547, #8036, #14926, .T. ) ;
#14357=EDGE_CURVE ( 'NONE', #20025, #1190, #518, .T. ) ;
#14366=EDGE_CURVE ( 'NONE', #5956, #10193, #17102, .T. ) ;
#14374=ORIENTED_EDGE ( 'NONE', *, *, #18350, .F. ) ;
#14383=EDGE_CURVE ( 'NONE', #8182, #13147, #6722, .T. ) ;
#14389=LINE ( 'NONE', #20915, #2044 ) ;
#14391=FACE_OUTER_BOUND ( 'NONE', #2148, .T. ) ;
#14395=CARTESIAN_POINT ( 'NONE',  ( 193.6079246875219155, 7.197283639386755638, -8.145074743996337574 ) ) ;
#14399=EDGE_LOOP ( 'NONE', ( #8013, #20288, #13717, #8720 ) ) ;
#14400=CARTESIAN_POINT ( 'NONE',  ( 198.6701878702990030, 10.11998265067189529, -3.762296834228767484 ) ) ;
#14406=EDGE_CURVE ( 'NONE', #3434, #6444, #16400, .T. ) ;
#14411=PLANE ( 'NONE',  #9497 ) ;
#14417=DIRECTION ( 'NONE',  ( -0.5000000000000054401, 0.8660254037844354880, -0.000000000000000000 ) ) ;
#14422=CARTESIAN_POINT ( 'NONE',  ( 194.6607596192359040, 7.805138170624078775, -8.669480444820575116 ) ) ;
#14423=VECTOR ( 'NONE', #514, 1000.000000000000114 ) ;
#14424=CARTESIAN_POINT ( 'NONE',  ( 198.9348002504466137, 6.148758762178306192, -4.550945818102817064 ) ) ;
#14425=EDGE_CURVE ( 'NONE', #6007, #17781, #1773, .T. ) ;
#14428=DIRECTION ( 'NONE',  ( -0.1005394128318207458, -0.05804645706261939847, -0.9932383577419421350 ) ) ;
#14433=LINE ( 'NONE', #9419, #19101 ) ;
#14434=DIRECTION ( 'NONE',  ( -0.3886714912512188591, -0.2243995901002276971, 0.8936326403234180482 ) ) ;
#14435=EDGE_CURVE ( 'NONE', #5032, #15249, #6978, .T. ) ;
#14438=AXIS2_PLACEMENT_3D ( 'NONE', #6068, #10738, #17432 ) ;
#14444=B_SPLINE_CURVE_WITH_KNOTS ( 'NONE', 3,
 ( #11786, #20221, #13773, #15482 ),
 .UNSPECIFIED., .F., .F.,
 ( 4, 4 ),
 ( 0.0001001963007107323439, 0.0009541820386879166192 ),
 .UNSPECIFIED. ) ;
#14446=DIRECTION ( 'NONE',  ( -0.5000000000000054401, 0.8660254037844354880, -0.000000000000000000 ) ) ;
#14450=ORIENTED_EDGE ( 'NONE', *, *, #2554, .F. ) ;
#14453=DIRECTION ( 'NONE',  ( 0.2961981327260293506, 0.1710100716628398243, 0.9396926207859056523 ) ) ;
#14454=DIRECTION ( 'NONE',  ( -0.8660254037844355990, -0.5000000000000055511, 0.000000000000000000 ) ) ;
#14455=LINE ( 'NONE', #7856, #3088 ) ;
#14462=FACE_OUTER_BOUND ( 'NONE', #18182, .T. ) ;
#14463=DIRECTION ( 'NONE',  ( 0.5000000000000054401, -0.8660254037844354880, 0.000000000000000000 ) ) ;
#14464=DIRECTION ( 'NONE',  ( 0.8660254037844355990, 0.5000000000000054401, 8.343535232742331521E-16 ) ) ;
#14465=ORIENTED_EDGE ( 'NONE', *, *, #20447, .T. ) ;
#14469=DIRECTION ( 'NONE',  ( 0.8404609622711977091, 0.000000000000000000, -0.5418720982835085742 ) ) ;
#14470=CARTESIAN_POINT ( 'NONE',  ( 203.6497874834091704, 1.447950443965099421, -24.35247136794729528 ) ) ;
#14474=EDGE_CURVE ( 'NONE', #18696, #11314, #1685, .T. ) ;
#14475=AXIS2_PLACEMENT_3D ( 'NONE', #16384, #3139, #6707 ) ;
#14476=CARTESIAN_POINT ( 'NONE',  ( 214.0936945175409676, 14.36970118611001368, -22.03054070023868860 ) ) ;
#14480=CARTESIAN_POINT ( 'NONE',  ( 212.2886526734226607, 13.32755979150977943, -4.003039906354141308 ) ) ;
#14486=VECTOR ( 'NONE', #17590, 1000.000000000000114 ) ;
#14490=VERTEX_POINT ( 'NONE', #2295 ) ;
#14494=EDGE_CURVE ( 'NONE', #112, #7973, #8749, .T. ) ;
#14504=VERTEX_POINT ( 'NONE', #15560 ) ;
#14506=CARTESIAN_POINT ( 'NONE',  ( 212.3836630237427414, 18.03746122203795466, -7.515250618841537111 ) ) ;
#14507=VERTEX_POINT ( 'NONE', #809 ) ;
#14510=DIRECTION ( 'NONE',  ( 0.8689290541588631234, 0.000000000000000000, 0.4949366614412228360 ) ) ;
#14511=EDGE_CURVE ( 'NONE', #20444, #19176, #17128, .T. ) ;
#14512=LINE ( 'NONE', #16399, #16253 ) ;
#14518=ORIENTED_EDGE ( 'NONE', *, *, #10430, .T. ) ;
#14528=CARTESIAN_POINT ( 'NONE',  ( 216.1735466947513942, 15.94087575960949010, -13.99568204168108743 ) ) ;
#14529=CARTESIAN_POINT ( 'NONE',  ( 205.8264633344831225, 9.596613037118636669, -14.00000000000005507 ) ) ;
#14534=CIRCLE ( 'NONE', #16551, 12.47473710546057823 ) ;
#14539=ORIENTED_EDGE ( 'NONE', *, *, #14740, .F. ) ;
#14543=ORIENTED_EDGE ( 'NONE', *, *, #14071, .T. ) ;
#14557=CARTESIAN_POINT ( 'NONE',  ( 212.7108869958215109, 14.10238615300026410, -22.72623880687309139 ) ) ;
#14559=AXIS2_PLACEMENT_3D ( 'NONE', #14400, #19054, #10993 ) ;
#14561=DIRECTION ( 'NONE',  ( -0.8660254037844357100, -0.5000000000000051070, 0.000000000000000000 ) ) ;
#14563=CARTESIAN_POINT ( 'NONE',  ( 208.4761278624580711, 5.007259451653140125, -14.00000000000005507 ) ) ;
#14566=CARTESIAN_POINT ( 'NONE',  ( 218.3559741392791125, 9.938571268484574617, -21.18305361806777043 ) ) ;
#14568=DIRECTION ( 'NONE',  ( 0.6299240516454600591, 0.3636868207865312508, 0.6862416378687270502 ) ) ;
#14570=CYLINDRICAL_SURFACE ( 'NONE', #668, 12.47473710546057646 ) ;
#14589=VERTEX_POINT ( 'NONE', #18513 ) ;
#14592=CARTESIAN_POINT ( 'NONE',  ( 203.8931977501677295, 8.657464312035081377, -1.876704962898965823 ) ) ;
#14597=CIRCLE ( 'NONE', #18292, 12.47473710546057823 ) ;
#14601=DIRECTION ( 'NONE',  ( -0.5000000000000051070, 0.8660254037844359321, -0.000000000000000000 ) ) ;
#14603=EDGE_CURVE ( 'NONE', #9561, #15382, #4302, .T. ) ;
#14606=CIRCLE ( 'NONE', #17979, 11.94520687646042667 ) ;
#14611=LINE ( 'NONE', #1555, #4040 ) ;
#14617=LINE ( 'NONE', #5996, #17061 ) ;
#14623=EDGE_LOOP ( 'NONE', ( #18956, #6996, #16190, #15834, #2567, #1802 ) ) ;
#14624=EDGE_LOOP ( 'NONE', ( #19947, #4716, #15458, #5448, #13514 ) ) ;
#14625=PLANE ( 'NONE',  #8137 ) ;
#14626=DIRECTION ( 'NONE',  ( 0.5000000000000049960, -0.8660254037844358210, 0.000000000000000000 ) ) ;
#14627=EDGE_CURVE ( 'NONE', #10364, #835, #12375, .T. ) ;
#14629=VECTOR ( 'NONE', #2371, 1000.000000000000227 ) ;
#14633=CARTESIAN_POINT ( 'NONE',  ( 198.5997926933885083, 20.69401370670428619, -1.545471579934808215 ) ) ;
#14635=CARTESIAN_POINT ( 'NONE',  ( 209.1514512894397058, 12.04734498975753354, -12.44962402344209274 ) ) ;
#14638=VERTEX_POINT ( 'NONE', #3945 ) ;
#14639=VERTEX_POINT ( 'NONE', #13499 ) ;
#14640=DIRECTION ( 'NONE',  ( 0.5000000000000052180, -0.8660254037844355990, -5.551115123125782086E-17 ) ) ;
#14646=DIRECTION ( 'NONE',  ( -0.5000000000000054401, 0.8660254037844354880, -0.000000000000000000 ) ) ;
#14647=DIRECTION ( 'NONE',  ( -0.7235536692358585098, -0.4177439057064702421, 0.5495089780708132254 ) ) ;
#14659=CIRCLE ( 'NONE', #17346, 12.47473710546057823 ) ;
#14662=VERTEX_POINT ( 'NONE', #19630 ) ;
#14669=ORIENTED_EDGE ( 'NONE', *, *, #186, .F. ) ;
#14671=CARTESIAN_POINT ( 'NONE',  ( 208.4761278624580711, 5.007259451653140125, -14.00000000000005507 ) ) ;
#14677=ORIENTED_EDGE ( 'NONE', *, *, #2821, .T. ) ;
#14689=FACE_OUTER_BOUND ( 'NONE', #2806, .T. ) ;
#14698=AXIS2_PLACEMENT_3D ( 'NONE', #12595, #9490, #4423 ) ;
#14701=CARTESIAN_POINT ( 'NONE',  ( 198.3288405652164670, -0.8512796009538451392, -9.718744748712973447 ) ) ;
#14704=LINE ( 'NONE', #1644, #20017 ) ;
#14706=DIRECTION ( 'NONE',  ( 0.5000000000000051070, -0.8660254037844359321, 0.000000000000000000 ) ) ;
#14712=VECTOR ( 'NONE', #17394, 1000.000000000000114 ) ;
#14716=EDGE_CURVE ( 'NONE', #4917, #9963, #3397, .T. ) ;
#14717=ORIENTED_EDGE ( 'NONE', *, *, #6639, .T. ) ;
#14725=ORIENTED_EDGE ( 'NONE', *, *, #3327, .F. ) ;
#14727=VERTEX_POINT ( 'NONE', #16777 ) ;
#14733=VERTEX_POINT ( 'NONE', #10288 ) ;
#14735=CARTESIAN_POINT ( 'NONE',  ( 205.4973105777689000, 2.514618399827694972, -26.58724934764007841 ) ) ;
#14736=EDGE_CURVE ( 'NONE', #9266, #4941, #13032, .T. ) ;
#14740=EDGE_CURVE ( 'NONE', #12762, #8980, #8713, .T. ) ;
#14756=ORIENTED_EDGE ( 'NONE', *, *, #18302, .F. ) ;
#14757=CARTESIAN_POINT ( 'NONE',  ( 210.4416572331711279, 5.884444511168165803, -1.889534153981373921 ) ) ;
#14768=FACE_OUTER_BOUND ( 'NONE', #2154, .T. ) ;
#14770=CARTESIAN_POINT ( 'NONE',  ( 216.5584123369822009, 15.79270668264091881, -15.43274561385901045 ) ) ;
#14771=CARTESIAN_POINT ( 'NONE',  ( 195.0976485947789456, 3.402328959064704783, -12.53629070788332278 ) ) ;
#14776=DIRECTION ( 'NONE',  ( 0.8660254037844355990, 0.5000000000000054401, -1.334965637238773043E-14 ) ) ;
#14778=CONICAL_SURFACE ( 'NONE', #19474, 13.07248899748297433, 0.6693469023067423196 ) ;
#14784=ORIENTED_EDGE ( 'NONE', *, *, #16022, .F. ) ;
#14791=TOROIDAL_SURFACE ( 'NONE', #11714, 1.003313105759043200, 1.000000000000000000 ) ;
#14803=CIRCLE ( 'NONE', #11391, 11.94520687646042667 ) ;
#14809=LINE ( 'NONE', #258, #17362 ) ;
#14820=DIRECTION ( 'NONE',  ( 0.5000000000000054401, -0.8660254037844354880, 0.000000000000000000 ) ) ;
#14826=DIRECTION ( 'NONE',  ( -0.5000000000000054401, 0.8660254037844354880, -0.000000000000000000 ) ) ;
#14831=CARTESIAN_POINT ( 'NONE',  ( 201.2754665570134591, 0.5923418568450431465, -22.94176278698363092 ) ) ;
#14833=EDGE_CURVE ( 'NONE', #2143, #9868, #18578, .T. ) ;
#14835=ORIENTED_EDGE ( 'NONE', *, *, #18211, .T. ) ;
#14836=CONICAL_SURFACE ( 'NONE', #5651, 13.07248899748297433, 0.6693469023067423196 ) ;
#14839=CARTESIAN_POINT ( 'NONE',  ( 208.4761278624580711, 5.007259451653140125, -14.00000000000005507 ) ) ;
#14843=DIRECTION ( 'NONE',  ( -0.5943026915289566503, -0.3431208189343674109, 0.7273736415730548410 ) ) ;
#14844=EDGE_CURVE ( 'NONE', #13380, #13321, #4587, .T. ) ;
#14847=B_SPLINE_CURVE_WITH_KNOTS ( 'NONE', 3,
 ( #2125, #20333, #6977, #13464 ),
 .UNSPECIFIED., .F., .F.,
 ( 4, 4 ),
 ( 1.122767056962631348E-06, 0.0008551085050396736416 ),
 .UNSPECIFIED. ) ;
#14848=CYLINDRICAL_SURFACE ( 'NONE', #16564, 12.47473710546057646 ) ;
#14850=CARTESIAN_POINT ( 'NONE',  ( 208.2336538649943236, 4.094446933302576142, -25.81526893633797570 ) ) ;
#14854=LINE ( 'NONE', #16215, #12781 ) ;
#14860=DIRECTION ( 'NONE',  ( -0.5000000000000054401, 0.8660254037844354880, -0.000000000000000000 ) ) ;
#14862=EDGE_CURVE ( 'NONE', #18411, #9311, #7272, .T. ) ;
#14865=CARTESIAN_POINT ( 'NONE',  ( 205.5718816476997688, 14.10467741091863658, -2.341985411377013548 ) ) ;
#14871=DIRECTION ( 'NONE',  ( 0.7500000000000015543, 0.4330127018922264037, 0.4999999999999917288 ) ) ;
#14873=CARTESIAN_POINT ( 'NONE',  ( 195.0230240956219347, 3.359244484388281826, -14.00000000000005507 ) ) ;
#14877=CARTESIAN_POINT ( 'NONE',  ( 208.0983737146324870, 5.661548828456886895, -14.00000000000005507 ) ) ;
#14878=DIRECTION ( 'NONE',  ( -0.5000000000000054401, 0.8660254037844354880, -0.000000000000000000 ) ) ;
#14879=ADVANCED_FACE ( 'NONE', ( #16229 ), #20880, .T. ) ;
#14880=ORIENTED_EDGE ( 'NONE', *, *, #11042, .T. ) ;
#14883=CARTESIAN_POINT ( 'NONE',  ( 199.2144802262915846, 21.04890371929339921, -14.00000000000005507 ) ) ;
#14888=ORIENTED_EDGE ( 'NONE', *, *, #11068, .F. ) ;
#14889=VERTEX_POINT ( 'NONE', #12742 ) ;
#14897=DIRECTION ( 'NONE',  ( 0.8660254037844373753, 0.5000000000000022204, 0.000000000000000000 ) ) ;
#14899=DIRECTION ( 'NONE',  ( 0.5000000000000054401, -0.8660254037844354880, 0.000000000000000000 ) ) ;
#14909=CARTESIAN_POINT ( 'NONE',  ( 212.0555786093015911, 13.72404367964075789, -3.627669900420236626 ) ) ;
#14914=CARTESIAN_POINT ( 'NONE',  ( 198.8341126585713425, -1.332380712484759755, -16.70797078425209747 ) ) ;
#14915=VERTEX_POINT ( 'NONE', #14557 ) ;
#14917=VECTOR ( 'NONE', #19117, 1000.000000000000114 ) ;
#14924=DIRECTION ( 'NONE',  ( 0.5000000000000054401, -0.8660254037844354880, 0.000000000000000000 ) ) ;
#14925=CARTESIAN_POINT ( 'NONE',  ( 208.2480327748888556, 26.26442771496472162, -20.84195174293596153 ) ) ;
#14926=LINE ( 'NONE', #5342, #177 ) ;
#14927=EDGE_LOOP ( 'NONE', ( #10925, #16837, #17686, #6105, #12159 ) ) ;
#14928=ORIENTED_EDGE ( 'NONE', *, *, #10826, .T. ) ;
#14930=ORIENTED_EDGE ( 'NONE', *, *, #6956, .F. ) ;
#14932=AXIS2_PLACEMENT_3D ( 'NONE', #420, #16326, #6865 ) ;
#14934=VECTOR ( 'NONE', #4891, 1000.000000000000000 ) ;
#14940=VECTOR ( 'NONE', #20048, 1000.000000000000114 ) ;
#14941=CARTESIAN_POINT ( 'NONE',  ( 214.8856909933734300, 7.826610718103062858, -14.00000000000005507 ) ) ;
#14942=VERTEX_POINT ( 'NONE', #19501 ) ;
#14944=CARTESIAN_POINT ( 'NONE',  ( 215.3464568589922408, 15.62403312296995317, -9.340893379680396791 ) ) ;
#14945=PLANE ( 'NONE',  #10384 ) ;
#14948=ORIENTED_EDGE ( 'NONE', *, *, #7277, .T. ) ;
#14950=TOROIDAL_SURFACE ( 'NONE', #13241, 6.960520131757804485, 1.000000000000000000 ) ;
#14954=CIRCLE ( 'NONE', #4775, 12.47473710546057823 ) ;
#14955=FACE_OUTER_BOUND ( 'NONE', #453, .T. ) ;
#14957=CARTESIAN_POINT ( 'NONE',  ( 198.6079246875219724, -1.462970398457601240, -8.145074743996339350 ) ) ;
#14962=ORIENTED_EDGE ( 'NONE', *, *, #9775, .F. ) ;
#14963=ORIENTED_EDGE ( 'NONE', *, *, #5654, .F. ) ;
#14965=ORIENTED_EDGE ( 'NONE', *, *, #5437, .F. ) ;
#14968=AXIS2_PLACEMENT_3D ( 'NONE', #6298, #11296, #9583 ) ;
#14969=VERTEX_POINT ( 'NONE', #323 ) ;
#14977=CARTESIAN_POINT ( 'NONE',  ( 212.8906072256780533, 14.02913777190325817, -22.83852658738941699 ) ) ;
#14978=LINE ( 'NONE', #16650, #11020 ) ;
#14979=VERTEX_POINT ( 'NONE', #11775 ) ;
#14981=CARTESIAN_POINT ( 'NONE',  ( 207.5029616403657258, 10.91857914292485532, -25.96288910428604879 ) ) ;
#14982=ADVANCED_FACE ( 'NONE', ( #14768 ), #13582, .F. ) ;
#14984=DIRECTION ( 'NONE',  ( 0.5000000000000051070, -0.8660254037844359321, 0.000000000000000000 ) ) ;
#14996=ORIENTED_EDGE ( 'NONE', *, *, #5108, .F. ) ;
#15000=EDGE_CURVE ( 'NONE', #5382, #1746, #8971, .T. ) ;
#15005=CARTESIAN_POINT ( 'NONE',  ( 198.4225180578738161, 5.321943238602927728, -4.915515517929134326 ) ) ;
#15006=LINE ( 'NONE', #7120, #2713 ) ;
#15008=AXIS2_PLACEMENT_3D ( 'NONE', #5643, #19962, #7136 ) ;
#15010=ADVANCED_FACE ( 'NONE', ( #16342 ), #2911, .T. ) ;
#15016=CARTESIAN_POINT ( 'NONE',  ( 192.4890135470689074, 6.551279991246921064, -15.47241223419981537 ) ) ;
#15019=EDGE_CURVE ( 'NONE', #10014, #3518, #16114, .T. ) ;
#15021=ORIENTED_EDGE ( 'NONE', *, *, #13963, .T. ) ;
#15022=DIRECTION ( 'NONE',  ( -0.6048098792058420603, 0.000000000000000000, 0.7963698952214447457 ) ) ;
#15023=LINE ( 'NONE', #14909, #5109 ) ;
#15024=DIRECTION ( 'NONE',  ( -0.5000000000000057732, 0.8660254037844352659, 0.000000000000000000 ) ) ;
#15035=AXIS2_PLACEMENT_3D ( 'NONE', #11098, #12802, #9595 ) ;
#15040=FACE_BOUND ( 'NONE', #3249, .T. ) ;
#15045=ORIENTED_EDGE ( 'NONE', *, *, #2941, .F. ) ;
#15055=VERTEX_POINT ( 'NONE', #13264 ) ;
#15058=EDGE_LOOP ( 'NONE', ( #9692, #20798, #11623, #16077 ) ) ;
#15060=EDGE_CURVE ( 'NONE', #17374, #14979, #14978, .T. ) ;
#15063=CARTESIAN_POINT ( 'NONE',  ( 205.0443405901917231, 9.676103521955072395, -14.65894010836695038 ) ) ;
#15067=DIRECTION ( 'NONE',  ( -0.8660254037844355990, -0.5000000000000054401, 0.000000000000000000 ) ) ;
#15069=ORIENTED_EDGE ( 'NONE', *, *, #13192, .F. ) ;
#15070=ORIENTED_EDGE ( 'NONE', *, *, #8831, .T. ) ;
#15072=VERTEX_POINT ( 'NONE', #13158 ) ;
#15073=ORIENTED_EDGE ( 'NONE', *, *, #1330, .F. ) ;
#15075=DIRECTION ( 'NONE',  ( 0.4330127018922105830, 0.2499999999999990563, -0.8660254037844432595 ) ) ;
#15077=EDGE_LOOP ( 'NONE', ( #12049, #6427, #15877, #8258 ) ) ;
#15079=CIRCLE ( 'NONE', #17766, 12.47473710546057823 ) ;
#15080=CARTESIAN_POINT ( 'NONE',  ( 218.0611881365336444, 9.768376490446161853, -19.34736286182901210 ) ) ;
#15081=ORIENTED_EDGE ( 'NONE', *, *, #8642, .F. ) ;
#15086=PLANE ( 'NONE',  #1756 ) ;
#15091=FACE_OUTER_BOUND ( 'NONE', #17738, .T. ) ;
#15095=CARTESIAN_POINT ( 'NONE',  ( 206.7427512303946457, 3.748880134758005411, -26.11230899909614678 ) ) ;
#15101=VERTEX_POINT ( 'NONE', #3602 ) ;
#15103=CIRCLE ( 'NONE', #8296, 12.47473710546057823 ) ;
#15105=DIRECTION ( 'NONE',  ( 0.5000000000000051070, -0.8660254037844359321, 0.000000000000000000 ) ) ;
#15106=DIRECTION ( 'NONE',  ( 0.5000000000000051070, -0.8660254037844355990, -4.163336342344335178E-17 ) ) ;
#15107=ORIENTED_EDGE ( 'NONE', *, *, #3317, .F. ) ;
#15109=EDGE_CURVE ( 'NONE', #1927, #18151, #14053, .T. ) ;
#15110=CARTESIAN_POINT ( 'NONE',  ( 209.3941655698033912, 12.18747614486167308, -16.05373426534894321 ) ) ;
#15112=DIRECTION ( 'NONE',  ( -0.8660254037844357100, -0.5000000000000051070, 0.000000000000000000 ) ) ;
#15116=FACE_OUTER_BOUND ( 'NONE', #7796, .T. ) ;
#15122=ORIENTED_EDGE ( 'NONE', *, *, #6210, .T. ) ;
#15124=CARTESIAN_POINT ( 'NONE',  ( 200.8946500511725333, -0.1427288941911568354, -6.310089745291766583 ) ) ;
#15131=CARTESIAN_POINT ( 'NONE',  ( 208.8107687779841228, 4.427644383670616079, -14.00000000000005507 ) ) ;
#15136=CARTESIAN_POINT ( 'NONE',  ( 217.4835782137190279, 9.950099484899608271, -7.237580838290172736 ) ) ;
#15143=EDGE_CURVE ( 'NONE', #5172, #4848, #20254, .T. ) ;
#15144=CARTESIAN_POINT ( 'NONE',  ( 204.2542003381767017, 1.796908368366799680, -1.942038651984764996 ) ) ;
#15146=CARTESIAN_POINT ( 'NONE',  ( 208.8107687779841228, 4.427644383670616079, -14.00000000000005507 ) ) ;
#15154=CARTESIAN_POINT ( 'NONE',  ( 195.0976485947789456, 3.402328959064704783, -12.53629070788332278 ) ) ;
#15155=B_SPLINE_CURVE_WITH_KNOTS ( 'NONE', 3,
 ( #18752, #10672, #2745, #15584 ),
 .UNSPECIFIED., .F., .F.,
 ( 4, 4 ),
 ( 6.222750521083429372E-05, 0.0007348782972656951393 ),
 .UNSPECIFIED. ) ;
#15158=ORIENTED_EDGE ( 'NONE', *, *, #15439, .F. ) ;
#15159=EDGE_CURVE ( 'NONE', #437, #15357, #5716, .T. ) ;
#15161=CIRCLE ( 'NONE', #11403, 12.47473710546057823 ) ;
#15165=EDGE_CURVE ( 'NONE', #2805, #8118, #8195, .T. ) ;
#15177=ORIENTED_EDGE ( 'NONE', *, *, #6378, .T. ) ;
#15182=CARTESIAN_POINT ( 'NONE',  ( 212.9776690748797989, 18.38041077556222191, -19.29168348739316130 ) ) ;
#15183=CARTESIAN_POINT ( 'NONE',  ( 218.0822574325961511, 10.03814007800654551, -19.43577154980806299 ) ) ;
#15184=ORIENTED_EDGE ( 'NONE', *, *, #6158, .F. ) ;
#15187=CARTESIAN_POINT ( 'NONE',  ( 213.2500461588270468, 13.88262057910513825, -23.06309126349817618 ) ) ;
#15190=FACE_OUTER_BOUND ( 'NONE', #11141, .T. ) ;
#15194=CARTESIAN_POINT ( 'NONE',  ( 216.6298941398503359, 15.83397672076898566, -14.01558723443205068 ) ) ;
#15196=CARTESIAN_POINT ( 'NONE',  ( 214.8665333410018263, 15.34694915066777909, -8.609703802792745719 ) ) ;
#15197=ORIENTED_EDGE ( 'NONE', *, *, #14844, .T. ) ;
#15198=LINE ( 'NONE', #15306, #14940 ) ;
#15207=CARTESIAN_POINT ( 'NONE',  ( 212.8527399996651752, 6.761277556564890823, -3.125199447383528284 ) ) ;
#15211=CARTESIAN_POINT ( 'NONE',  ( 206.7852296553355131, 3.258198825955272326, -1.053683606938436768 ) ) ;
#15214=VECTOR ( 'NONE', #18789, 1000.000000000000000 ) ;
#15222=CARTESIAN_POINT ( 'NONE',  ( 196.2242827900706175, 4.229814195430575907, -19.53076827296950668 ) ) ;
#15227=EDGE_LOOP ( 'NONE', ( #15380, #20868, #14374, #11339, #19296, #2329 ) ) ;
#15229=ADVANCED_FACE ( 'NONE', ( #15413 ), #9983, .T. ) ;
#15230=DIRECTION ( 'NONE',  ( 0.8660254037844357100, 0.5000000000000053291, 0.000000000000000000 ) ) ;
#15237=ADVANCED_FACE ( 'NONE', ( #3829 ), #6999, .F. ) ;
#15243=CARTESIAN_POINT ( 'NONE',  ( 205.8894739819445761, 2.741034046794848855, -25.34310559273324159 ) ) ;
#15245=EDGE_CURVE ( 'NONE', #8118, #7107, #17129, .T. ) ;
#15246=DIRECTION ( 'NONE',  ( -0.8660254037844354880, -0.5000000000000055511, 0.000000000000000000 ) ) ;
#15249=VERTEX_POINT ( 'NONE', #15311 ) ;
#15253=CARTESIAN_POINT ( 'NONE',  ( 203.2584098944515461, 1.737194726502687470, -24.64792178047091653 ) ) ;
#15254=AXIS2_PLACEMENT_3D ( 'NONE', #16823, #19991, #708 ) ;
#15256=ORIENTED_EDGE ( 'NONE', *, *, #5888, .T. ) ;
#15258=LINE ( 'NONE', #10016, #19651 ) ;
#15259=DIRECTION ( 'NONE',  ( -0.8645602258681718277, -0.4991540791356397500, -0.05814482891046558743 ) ) ;
#15264=EDGE_CURVE ( 'NONE', #10920, #16780, #20776, .T. ) ;
#15265=ORIENTED_EDGE ( 'NONE', *, *, #7824, .T. ) ;
#15266=AXIS2_PLACEMENT_3D ( 'NONE', #8565, #17053, #934 ) ;
#15271=CARTESIAN_POINT ( 'NONE',  ( 203.7983348743963461, 8.956721786528811791, -25.65046807331631129 ) ) ;
#15275=DIRECTION ( 'NONE',  ( -0.8944271909999147452, 0.000000000000000000, 0.4472135954999602592 ) ) ;
#15277=VERTEX_POINT ( 'NONE', #3185 ) ;
#15281=VERTEX_POINT ( 'NONE', #4361 ) ;
#15285=EDGE_CURVE ( 'NONE', #11917, #7471, #6041, .T. ) ;
#15286=CONICAL_SURFACE ( 'NONE', #18651, 4.999999999999944933, 1.566852922939436121 ) ;
#15287=EDGE_LOOP ( 'NONE', ( #13480, #5102, #7210, #20766 ) ) ;
#15290=VERTEX_POINT ( 'NONE', #1495 ) ;
#15291=EDGE_CURVE ( 'NONE', #8683, #13569, #15802, .T. ) ;
#15295=VECTOR ( 'NONE', #15889, 1000.000000000000227 ) ;
#15296=CYLINDRICAL_SURFACE ( 'NONE', #17232, 7.960520131757808038 ) ;
#15298=VECTOR ( 'NONE', #17059, 1000.000000000000000 ) ;
#15300=DIRECTION ( 'NONE',  ( -0.5000000000000054401, 0.8660254037844354880, -0.000000000000000000 ) ) ;
#15304=CARTESIAN_POINT ( 'NONE',  ( 195.3983247169765320, 4.106973660946812821, -14.97708215022677791 ) ) ;
#15306=CARTESIAN_POINT ( 'NONE',  ( 200.0522846737218856, -0.6290687716183213096, -5.585956497639848806 ) ) ;
#15308=ORIENTED_EDGE ( 'NONE', *, *, #15019, .T. ) ;
#15311=CARTESIAN_POINT ( 'NONE',  ( 216.7438708388689292, 9.007822994031293717, -21.66653917424403986 ) ) ;
#15312=VECTOR ( 'NONE', #20178, 1000.000000000000227 ) ;
#15316=ORIENTED_EDGE ( 'NONE', *, *, #7586, .T. ) ;
#15320=DIRECTION ( 'NONE',  ( 0.6634139481689435014, 0.3830222215594971114, 0.6427876096865291489 ) ) ;
#15326=ADVANCED_FACE ( 'NONE', ( #7942 ), #16796, .T. ) ;
#15327=DIRECTION ( 'NONE',  ( -0.5000000000000054401, 0.8660254037844354880, -0.000000000000000000 ) ) ;
#15330=DIRECTION ( 'NONE',  ( 0.5000000000000054401, -0.8660254037844354880, -2.220446049250312834E-16 ) ) ;
#15334=VERTEX_POINT ( 'NONE', #17401 ) ;
#15336=FACE_OUTER_BOUND ( 'NONE', #20667, .T. ) ;
#15338=PLANE ( 'NONE',  #20208 ) ;
#15351=LINE ( 'NONE', #10749, #14157 ) ;
#15352=AXIS2_PLACEMENT_3D ( 'NONE', #7430, #20374, #1096 ) ;
#15355=CARTESIAN_POINT ( 'NONE',  ( 209.4907977912995136, 12.24326678395483725, -12.83329734752810225 ) ) ;
#15357=VERTEX_POINT ( 'NONE', #10932 ) ;
#15358=ORIENTED_EDGE ( 'NONE', *, *, #15371, .T. ) ;
#15363=VERTEX_POINT ( 'NONE', #15822 ) ;
#15370=DIRECTION ( 'NONE',  ( 0.5000000000000054401, -0.8660254037844354880, 0.000000000000000000 ) ) ;
#15371=EDGE_CURVE ( 'NONE', #12727, #15665, #15724, .T. ) ;
#15372=CARTESIAN_POINT ( 'NONE',  ( 205.0584722627656049, 9.507252542736225109, -1.872710068124171290 ) ) ;
#15380=ORIENTED_EDGE ( 'NONE', *, *, #9028, .F. ) ;
#15382=VERTEX_POINT ( 'NONE', #2983 ) ;
#15387=ORIENTED_EDGE ( 'NONE', *, *, #19141, .T. ) ;
#15390=CYLINDRICAL_SURFACE ( 'NONE', #25, 12.47473710546057646 ) ;
#15392=VERTEX_POINT ( 'NONE', #9836 ) ;
#15397=DIRECTION ( 'NONE',  ( 0.5000000000000052180, -0.8660254037844355990, 0.000000000000000000 ) ) ;
#15405=DIRECTION ( 'NONE',  ( -0.2483788854153066994, -0.1434016163555488221, -0.9579895123154877901 ) ) ;
#15406=CARTESIAN_POINT ( 'NONE',  ( 212.8960219706529813, 6.786266414165766925, -3.025685634606239294 ) ) ;
#15413=FACE_OUTER_BOUND ( 'NONE', #15058, .T. ) ;
#15416=LINE ( 'NONE', #7320, #8583 ) ;
#15417=VERTEX_POINT ( 'NONE', #5278 ) ;
#15418=DIRECTION ( 'NONE',  ( -0.5000000000000051070, 0.8660254037844359321, -0.000000000000000000 ) ) ;
#15419=CARTESIAN_POINT ( 'NONE',  ( 201.7020968622623798, 0.3234507395478347092, -5.321846656828017608 ) ) ;
#15422=AXIS2_PLACEMENT_3D ( 'NONE', #6484, #13086, #11282 ) ;
#15424=DIRECTION ( 'NONE',  ( -0.8660254037844354880, -0.5000000000000055511, 0.000000000000000000 ) ) ;
#15426=ORIENTED_EDGE ( 'NONE', *, *, #16298, .T. ) ;
#15430=DIRECTION ( 'NONE',  ( -0.5000000000000054401, 0.8660254037844354880, -0.000000000000000000 ) ) ;
#15431=CARTESIAN_POINT ( 'NONE',  ( 216.2517163971578782, 7.460585314318640471, -14.00000000000005507 ) ) ;
#15432=B_SPLINE_CURVE_WITH_KNOTS ( 'NONE', 3,
 ( #5307, #8819, #7013, #357 ),
 .UNSPECIFIED., .F., .F.,
 ( 4, 4 ),
 ( 5.324950961081164366E-05, 0.0009072352475936213290 ),
 .UNSPECIFIED. ) ;
#15433=ORIENTED_EDGE ( 'NONE', *, *, #6942, .T. ) ;
#15437=VERTEX_POINT ( 'NONE', #8144 ) ;
#15439=EDGE_CURVE ( 'NONE', #13569, #8683, #5609, .T. ) ;
#15440=AXIS2_PLACEMENT_3D ( 'NONE', #10940, #7747, #6250 ) ;
#15442=AXIS2_PLACEMENT_3D ( 'NONE', #756, #10372, #13478 ) ;
#15445=ORIENTED_EDGE ( 'NONE', *, *, #2145, .F. ) ;
#15448=EDGE_LOOP ( 'NONE', ( #12824, #13433, #1314, #8869 ) ) ;
#15450=CARTESIAN_POINT ( 'NONE',  ( 198.2231302758563913, -1.169925316738297028, -11.16899820387730635 ) ) ;
#15453=CARTESIAN_POINT ( 'NONE',  ( 203.9371734008334158, 8.505830985348726614, -1.717498466822810599 ) ) ;
#15455=VECTOR ( 'NONE', #633, 1000.000000000000114 ) ;
#15458=ORIENTED_EDGE ( 'NONE', *, *, #2941, .T. ) ;
#15461=DIRECTION ( 'NONE',  ( -0.5000000000000049960, 0.8660254037844357100, -0.000000000000000000 ) ) ;
#15464=CARTESIAN_POINT ( 'NONE',  ( 210.6089461623840009, 5.465822580604545955, -25.65046807331635748 ) ) ;
#15469=CARTESIAN_POINT ( 'NONE',  ( 199.3642739955437833, 5.865666282727633352, -4.003039906353938804 ) ) ;
#15474=CARTESIAN_POINT ( 'NONE',  ( 214.9156946368443926, 7.952324971666334008, -4.494676796018850951 ) ) ;
#15476=DIRECTION ( 'NONE',  ( 0.7235536692358650601, 0.4177439057064745165, 0.5495089780708014571 ) ) ;
#15480=EDGE_LOOP ( 'NONE', ( #4327, #14465, #3018, #13811 ) ) ;
#15482=CARTESIAN_POINT ( 'NONE',  ( 198.3288405652164670, -0.8512796009538451392, -9.718744748712973447 ) ) ;
#15490=DIRECTION ( 'NONE',  ( -0.6299240516454600591, -0.3636868207865312508, -0.6862416378687270502 ) ) ;
#15491=EDGE_CURVE ( 'NONE', #8387, #12920, #16134, .T. ) ;
#15493=ORIENTED_EDGE ( 'NONE', *, *, #3327, .T. ) ;
#15497=DIRECTION ( 'NONE',  ( 0.8660254037844355990, 0.5000000000000054401, 0.000000000000000000 ) ) ;
#15501=ORIENTED_EDGE ( 'NONE', *, *, #13807, .T. ) ;
#15506=CARTESIAN_POINT ( 'NONE',  ( 215.8932031078481941, 9.031895989412584314, -5.050953241461466625 ) ) ;
#15514=FACE_OUTER_BOUND ( 'NONE', #18282, .T. ) ;
#15516=EDGE_CURVE ( 'NONE', #12209, #4965, #20163, .T. ) ;
#15520=DIRECTION ( 'NONE',  ( 0.5171545105027488543, 0.2985792958513952544, -0.8021231927550450669 ) ) ;
#15526=DIRECTION ( 'NONE',  ( 0.8660254037844355990, 0.5000000000000054401, 0.000000000000000000 ) ) ;
#15528=EDGE_CURVE ( 'NONE', #6296, #17439, #16744, .T. ) ;
#15530=CARTESIAN_POINT ( 'NONE',  ( 210.7044991792821236, 12.94399760702244073, -24.25943249057096907 ) ) ;
#15534=ORIENTED_EDGE ( 'NONE', *, *, #1872, .T. ) ;
#15536=EDGE_CURVE ( 'NONE', #14507, #17368, #10466, .T. ) ;
#15538=PLANE ( 'NONE',  #7846 ) ;
#15546=ORIENTED_EDGE ( 'NONE', *, *, #16792, .F. ) ;
#15552=LINE ( 'NONE', #2500, #764 ) ;
#15553=B_SPLINE_CURVE_WITH_KNOTS ( 'NONE', 3,
 ( #6728, #1671, #89, #18198 ),
 .UNSPECIFIED., .F., .F.,
 ( 4, 4 ),
 ( 3.426792995114292227E-07, 0.0008543284172819957511 ),
 .UNSPECIFIED. ) ;
#15557=DIRECTION ( 'NONE',  ( -0.8660254037844357100, -0.5000000000000051070, 0.000000000000000000 ) ) ;
#15560=CARTESIAN_POINT ( 'NONE',  ( 201.5350480436278531, 7.118963263738831593, -2.551678190571418092 ) ) ;
#15561=VECTOR ( 'NONE', #14327, 1000.000000000000000 ) ;
#15563=ORIENTED_EDGE ( 'NONE', *, *, #13405, .T. ) ;
#15564=CYLINDRICAL_SURFACE ( 'NONE', #12234, 12.47473710546057646 ) ;
#15568=CARTESIAN_POINT ( 'NONE',  ( 196.8077463644258387, 4.389654366710942668, -7.132002368301173512 ) ) ;
#15574=CARTESIAN_POINT ( 'NONE',  ( 213.8895336909654361, 8.132690763974602888, -24.79563718815146345 ) ) ;
#15581=VERTEX_POINT ( 'NONE', #12304 ) ;
#15582=ORIENTED_EDGE ( 'NONE', *, *, #14494, .T. ) ;
#15584=CARTESIAN_POINT ( 'NONE',  ( 208.9119903699346708, 11.37804290162847209, -2.044871543907030631 ) ) ;
#15585=DIRECTION ( 'NONE',  ( 0.5000000000000051070, -0.8660254037844355990, -1.942890293094023946E-16 ) ) ;
#15588=FACE_OUTER_BOUND ( 'NONE', #20573, .T. ) ;
#15595=LINE ( 'NONE', #6123, #14169 ) ;
#15597=DIRECTION ( 'NONE',  ( 0.6634139481689350637, 0.3830222215594922264, -0.6427876096865409172 ) ) ;
#15599=DIRECTION ( 'NONE',  ( -0.8601696498176553130, -0.4966191788709760080, 0.1160929141252378949 ) ) ;
#15610=CIRCLE ( 'NONE', #18988, 12.47473710546057823 ) ;
#15618=EDGE_CURVE ( 'NONE', #15277, #5032, #18802, .T. ) ;
#15620=CIRCLE ( 'NONE', #5756, 12.47473710546057823 ) ;
#15627=LINE ( 'NONE', #18791, #17297 ) ;
#15629=VECTOR ( 'NONE', #1329, 1000.000000000000227 ) ;
#15631=ADVANCED_FACE ( 'NONE', ( #18760 ), #13571, .F. ) ;
#15632=VECTOR ( 'NONE', #20578, 1000.000000000000227 ) ;
#15633=DIRECTION ( 'NONE',  ( 0.8137976813493725814, 0.4698463103929604867, 0.3420201433256626622 ) ) ;
#15639=CARTESIAN_POINT ( 'NONE',  ( 200.9574494032262066, -0.1064716713780056168, -23.53124788243904320 ) ) ;
#15640=FACE_OUTER_BOUND ( 'NONE', #16227, .T. ) ;
#15644=ADVANCED_FACE ( 'NONE', ( #16952 ), #4932, .T. ) ;
#15645=DIRECTION ( 'NONE',  ( 0.5000000000000052180, -0.8660254037844355990, 2.220446049250312341E-16 ) ) ;
#15648=VECTOR ( 'NONE', #20730, 1000.000000000000114 ) ;
#15653=EDGE_CURVE ( 'NONE', #2505, #16451, #4128, .T. ) ;
#15658=CARTESIAN_POINT ( 'NONE',  ( 215.4868200432858600, 15.17402258341379451, -8.415281845792092597 ) ) ;
#15662=CARTESIAN_POINT ( 'NONE',  ( 216.5944766886066759, 8.921570241161999704, -4.392917125964956426 ) ) ;
#15665=VERTEX_POINT ( 'NONE', #20335 ) ;
#15668=CONICAL_SURFACE ( 'NONE', #18358, 13.07248899748297433, 0.6693469023067423196 ) ;
#15669=EDGE_CURVE ( 'NONE', #5690, #10014, #19913, .T. ) ;
#15670=AXIS2_PLACEMENT_3D ( 'NONE', #77, #12800, #18087 ) ;
#15681=DIRECTION ( 'NONE',  ( -0.5000000000000049960, 0.8660254037844357100, -0.000000000000000000 ) ) ;
#15683=CIRCLE ( 'NONE', #8150, 12.47473710546057823 ) ;
#15688=CARTESIAN_POINT ( 'NONE',  ( 200.1750369523376492, -0.5581977105158604235, -20.57673792763505460 ) ) ;
#15689=LINE ( 'NONE', #20429, #3244 ) ;
#15691=ORIENTED_EDGE ( 'NONE', *, *, #5947, .F. ) ;
#15696=VERTEX_POINT ( 'NONE', #7819 ) ;
#15697=LINE ( 'NONE', #12403, #9180 ) ;
#15698=DIRECTION ( 'NONE',  ( 0.9537419254229455579, 0.000000000000000000, -0.3006265784832282684 ) ) ;
#15705=CARTESIAN_POINT ( 'NONE',  ( 208.8107687779841228, 4.427644383670616079, -14.00000000000005507 ) ) ;
#15708=PRODUCT_DEFINITION_SHAPE ( 'NONE', 'NONE',  #8724 ) ;
#15709=CARTESIAN_POINT ( 'NONE',  ( 205.8564897284660731, 2.721990579170014080, -25.44774858730788125 ) ) ;
#15714=VECTOR ( 'NONE', #12751, 1000.000000000000114 ) ;
#15718=ORIENTED_EDGE ( 'NONE', *, *, #5009, .T. ) ;
#15722=ORIENTED_EDGE ( 'NONE', *, *, #16146, .T. ) ;
#15724=LINE ( 'NONE', #1186, #211 ) ;
#15727=ADVANCED_FACE ( 'NONE', ( #10788 ), #15799, .F. ) ;
#15728=CARTESIAN_POINT ( 'NONE',  ( 203.0727098700125737, 1.114774528527234798, -25.36561010639676184 ) ) ;
#15729=ORIENTED_EDGE ( 'NONE', *, *, #10228, .F. ) ;
#15734=CARTESIAN_POINT ( 'NONE',  ( 206.4411508673863409, 9.951503049707822512, -1.545471579934816875 ) ) ;
#15735=FACE_OUTER_BOUND ( 'NONE', #8167, .T. ) ;
#15738=DIRECTION ( 'NONE',  ( 0.6958540455341998276, 0.000000000000000000, 0.7181832268395633712 ) ) ;
#15740=CIRCLE ( 'NONE', #1846, 11.94520687646042667 ) ;
#15742=DIRECTION ( 'NONE',  ( 0.5000000000000054401, -0.8660254037844354880, 0.000000000000000000 ) ) ;
#15747=DIRECTION ( 'NONE',  ( 0.8660254037844355990, 0.5000000000000054401, 0.000000000000000000 ) ) ;
#15755=CIRCLE ( 'NONE', #20464, 12.47473710546057823 ) ;
#15757=CARTESIAN_POINT ( 'NONE',  ( 201.5350480436278531, 7.118963263738831593, -2.551678190571418092 ) ) ;
#15759=ORIENTED_EDGE ( 'NONE', *, *, #17264, .T. ) ;
#15762=CARTESIAN_POINT ( 'NONE',  ( 203.8433579509713809, 8.805705967725675265, -25.96288910428599550 ) ) ;
#15768=ORIENTED_EDGE ( 'NONE', *, *, #7208, .F. ) ;
#15770=CARTESIAN_POINT ( 'NONE',  ( 203.1960812450809897, 12.73300840892584063, -2.187257959407754804 ) ) ;
#15771=CARTESIAN_POINT ( 'NONE',  ( 197.9607918626003311, -1.063772618484184918, -11.13829696442576811 ) ) ;
#15773=EDGE_CURVE ( 'NONE', #20129, #18696, #6976, .T. ) ;
#15774=CARTESIAN_POINT ( 'NONE',  ( 209.8909370991932519, 2.556737970610027499, -14.00000000000005507 ) ) ;
#15776=B_SPLINE_CURVE_WITH_KNOTS ( 'NONE', 3,
 ( #7686, #2626, #9171, #10652 ),
 .UNSPECIFIED., .F., .F.,
 ( 4, 4 ),
 ( 3.280426939632746066E-07, 0.0006729788347498066783 ),
 .UNSPECIFIED. ) ;
#15777=ORIENTED_EDGE ( 'NONE', *, *, #15285, .F. ) ;
#15783=CARTESIAN_POINT ( 'NONE',  ( 198.8278877809574965, -0.5631545566074300790, -19.61257667712936126 ) ) ;
#15788=VERTEX_POINT ( 'NONE', #5049 ) ;
#15790=FACE_OUTER_BOUND ( 'NONE', #1184, .T. ) ;
#15792=CARTESIAN_POINT ( 'NONE',  ( 197.7058429191240521, 9.563217833519331634, -4.494676796018654663 ) ) ;
#15793=ORIENTED_EDGE ( 'NONE', *, *, #16233, .F. ) ;
#15798=CONICAL_SURFACE ( 'NONE', #14104, 10.85470691220533190, 0.8171114040043576665 ) ;
#15799=PLANE ( 'NONE',  #4283 ) ;
#15802=CIRCLE ( 'NONE', #7647, 7.960520131757807150 ) ;
#15804=CIRCLE ( 'NONE', #6619, 4.999999999999977796 ) ;
#15805=EDGE_CURVE ( 'NONE', #12331, #20124, #11476, .T. ) ;
#15807=CARTESIAN_POINT ( 'NONE',  ( 208.4761278624580711, 5.007259451653140125, -14.00000000000005507 ) ) ;
#15812=CIRCLE ( 'NONE', #17143, 12.47473710546057823 ) ;
#15813=DIRECTION ( 'NONE',  ( 0.5000000000000054401, -0.8660254037844354880, 0.000000000000000000 ) ) ;
#15819=ORIENTED_EDGE ( 'NONE', *, *, #15773, .T. ) ;
#15822=CARTESIAN_POINT ( 'NONE',  ( 216.7433590455158878, 9.780347600644502037, -22.03054070023868860 ) ) ;
#15825=AXIS2_PLACEMENT_3D ( 'NONE', #9890, #9584, #6396 ) ;
#15826=LINE ( 'NONE', #12333, #15214 ) ;
#15830=PLANE ( 'NONE',  #15352 ) ;
#15831=CARTESIAN_POINT ( 'NONE',  ( 208.2794616557154370, 15.66789945739891898, -26.10173121575784450 ) ) ;
#15832=CARTESIAN_POINT ( 'NONE',  ( 194.1738290307969805, 7.524008664312185957, -9.972943347741734854 ) ) ;
#15834=ORIENTED_EDGE ( 'NONE', *, *, #18715, .F. ) ;
#15836=CARTESIAN_POINT ( 'NONE',  ( 208.4761278624580711, 5.007259451653140125, -14.00000000000005507 ) ) ;
#15847=CARTESIAN_POINT ( 'NONE',  ( 191.7908974019474613, 16.76289617730678216, -23.06309126349794170 ) ) ;
#15850=EDGE_CURVE ( 'NONE', #2725, #13569, #224, .T. ) ;
#15851=AXIS2_PLACEMENT_3D ( 'NONE', #9964, #11588, #11168 ) ;
#15855=ORIENTED_EDGE ( 'NONE', *, *, #17940, .T. ) ;
#15856=DIRECTION ( 'NONE',  ( 0.2483788854152947367, 0.1434016163555419388, -0.9579895123154918979 ) ) ;
#15859=EDGE_CURVE ( 'NONE', #16512, #12634, #16312, .T. ) ;
#15861=EDGE_CURVE ( 'NONE', #18586, #2903, #13096, .T. ) ;
#15862=VERTEX_POINT ( 'NONE', #13126 ) ;
#15869=LINE ( 'NONE', #2932, #20193 ) ;
#15872=CARTESIAN_POINT ( 'NONE',  ( 200.1915427753721417, 0.2241520214996718663, -5.993340328401664863 ) ) ;
#15877=ORIENTED_EDGE ( 'NONE', *, *, #10268, .F. ) ;
#15880=CARTESIAN_POINT ( 'NONE',  ( 205.0662616026534693, 10.91332106064940888, -14.00000000000005507 ) ) ;
#15881=EDGE_CURVE ( 'NONE', #14889, #5590, #8340, .T. ) ;
#15884=LINE ( 'NONE', #12599, #20507 ) ;
#15885=VERTEX_POINT ( 'NONE', #8865 ) ;
#15888=CARTESIAN_POINT ( 'NONE',  ( 201.7020968622623798, 0.3234507395478347092, -5.321846656828017608 ) ) ;
#15889=DIRECTION ( 'NONE',  ( -0.1997192025788214753, -0.1153079353712215399, -0.9730448705798235842 ) ) ;
#15892=ORIENTED_EDGE ( 'NONE', *, *, #5139, .F. ) ;
#15894=DIRECTION ( 'NONE',  ( 0.2961981327260295171, 0.1710100716628401019, 0.9396926207859056523 ) ) ;
#15898=EDGE_CURVE ( 'NONE', #6007, #2199, #16828, .T. ) ;
#15903=CARTESIAN_POINT ( 'NONE',  ( 0.000000000000000000, 0.000000000000000000, 0.000000000000000000 ) ) ;
#15905=CARTESIAN_POINT ( 'NONE',  ( 209.3710013429994206, 26.91277392005484614, -18.25196083293883120 ) ) ;
#15907=DIRECTION ( 'NONE',  ( 0.5000000000000054401, -0.8660254037844354880, -2.081668171172167774E-16 ) ) ;
#15909=CARTESIAN_POINT ( 'NONE',  ( 202.0455819868764138, 0.5217619687064301015, -24.58554911381517627 ) ) ;
#15915=ORIENTED_EDGE ( 'NONE', *, *, #652, .F. ) ;
#15916=AXIS2_PLACEMENT_3D ( 'NONE', #473, #13401, #12991 ) ;
#15921=VERTEX_POINT ( 'NONE', #13653 ) ;
#15932=CARTESIAN_POINT ( 'NONE',  ( 209.9156946368443357, 16.61257900951069288, -4.494676796018852727 ) ) ;
#15935=VECTOR ( 'NONE', #4491, 1000.000000000000227 ) ;
#15937=CARTESIAN_POINT ( 'NONE',  ( 203.7027818574982518, 1.478546760110915903, -24.25943249057081630 ) ) ;
#15941=VERTEX_POINT ( 'NONE', #3996 ) ;
#15950=VERTEX_POINT ( 'NONE', #16927 ) ;
#15951=VERTEX_POINT ( 'NONE', #16613 ) ;
#15954=CARTESIAN_POINT ( 'NONE',  ( 209.9477407942357843, 12.50708294970442225, -14.41834690440041022 ) ) ;
#15955=VECTOR ( 'NONE', #19071, 1000.000000000000227 ) ;
#15960=AXIS2_PLACEMENT_3D ( 'NONE', #3979, #6934, #2392 ) ;
#15963=DIRECTION ( 'NONE',  ( -0.6518835024542932732, 0.000000000000000000, -0.7583191275630091210 ) ) ;
#15964=CIRCLE ( 'NONE', #9840, 11.98469917212512215 ) ;
#15965=VECTOR ( 'NONE', #7911, 1000.000000000000227 ) ;
#15968=CARTESIAN_POINT ( 'NONE',  ( 218.9878548032870071, 10.30338773994525425, -15.39542905462748479 ) ) ;
#15970=CARTESIAN_POINT ( 'NONE',  ( 203.9035579930133792, 8.663445801030889015, -26.12540443289068293 ) ) ;
#15976=EDGE_LOOP ( 'NONE', ( #18652, #7608, #8910, #15308 ) ) ;
#15980=B_SPLINE_CURVE_WITH_KNOTS ( 'NONE', 3,
 ( #11078, #17231, #2719, #13960 ),
 .UNSPECIFIED., .F., .F.,
 ( 4, 4 ),
 ( 1.578338979776156445E-06, 0.0006742291310223107702 ),
 .UNSPECIFIED. ) ;
#15981=FACE_OUTER_BOUND ( 'NONE', #20199, .T. ) ;
#15984=DIRECTION ( 'NONE',  ( 0.8660254037844355990, 0.5000000000000054401, 0.000000000000000000 ) ) ;
#15986=EDGE_CURVE ( 'NONE', #2041, #5298, #14803, .T. ) ;
#15987=ORIENTED_EDGE ( 'NONE', *, *, #17019, .T. ) ;
#15988=ADVANCED_FACE ( 'NONE', ( #19889 ), #8763, .F. ) ;
#15998=ORIENTED_EDGE ( 'NONE', *, *, #15165, .T. ) ;
#16001=DIRECTION ( 'NONE',  ( -0.5016613886297202063, 0.000000000000000000, 0.8650640734408641119 ) ) ;
#16014=AXIS2_PLACEMENT_3D ( 'NONE', #7017, #2477, #16784 ) ;
#16018=DIRECTION ( 'NONE',  ( 0.8137976813493681405, 0.4698463103929584328, -0.3420201433256762624 ) ) ;
#16022=EDGE_CURVE ( 'NONE', #5656, #14733, #13338, .T. ) ;
#16027=ORIENTED_EDGE ( 'NONE', *, *, #16252, .T. ) ;
#16028=AXIS2_PLACEMENT_3D ( 'NONE', #7404, #4457, #10479 ) ;
#16033=DIRECTION ( 'NONE',  ( -0.1005394128318083391, -0.05804645706261228610, 0.9932383577419438003 ) ) ;
#16039=ORIENTED_EDGE ( 'NONE', *, *, #13779, .F. ) ;
#16044=CARTESIAN_POINT ( 'NONE',  ( 215.7047814394237832, 8.407904449549567616, -14.00000000000005329 ) ) ;
#16047=ADVANCED_FACE ( 'NONE', ( #9475 ), #12276, .F. ) ;
#16051=ADVANCED_FACE ( 'NONE', ( #13864 ), #3942, .T. ) ;
#16052=CARTESIAN_POINT ( 'NONE',  ( 202.6586965015780208, 8.121741361019813255, -25.63868392505618488 ) ) ;
#16054=CARTESIAN_POINT ( 'NONE',  ( 212.8103755628029319, 7.252024676415511628, -2.709673684914666314 ) ) ;
#16058=ADVANCED_FACE ( 'NONE', ( #15981 ), #12426, .T. ) ;
#16060=EDGE_LOOP ( 'NONE', ( #9048, #8686 ) ) ;
#16061=VERTEX_POINT ( 'NONE', #1028 ) ;
#16062=LINE ( 'NONE', #20800, #13961 ) ;
#16064=DIRECTION ( 'NONE',  ( -0.7235536692358586208, -0.4177439057064700756, 0.5495089780708132254 ) ) ;
#16065=ORIENTED_EDGE ( 'NONE', *, *, #11381, .F. ) ;
#16067=EDGE_CURVE ( 'NONE', #7703, #8807, #15869, .T. ) ;
#16070=DIRECTION ( 'NONE',  ( 0.8660254037844352659, 0.5000000000000056621, 0.000000000000000000 ) ) ;
#16071=VECTOR ( 'NONE', #1759, 1000.000000000000000 ) ;
#16073=DIRECTION ( 'NONE',  ( -0.05035489893517527266, -0.02907241445524010384, -0.9983081582712679536 ) ) ;
#16076=CARTESIAN_POINT ( 'NONE',  ( 209.0220424616560422, 2.055081417730487470, -14.00000000000005507 ) ) ;
#16077=ORIENTED_EDGE ( 'NONE', *, *, #11708, .T. ) ;
#16078=LINE ( 'NONE', #6496, #11216 ) ;
#16082=CARTESIAN_POINT ( 'NONE',  ( 197.7136026671465743, -1.979307457663559422, -11.01983352639493496 ) ) ;
#16083=DIRECTION ( 'NONE',  ( -0.5000000000000049960, 0.8660254037844358210, -0.000000000000000000 ) ) ;
#16086=EDGE_LOOP ( 'NONE', ( #10090, #14717, #3827, #4495, #20851, #18399 ) ) ;
#16087=LINE ( 'NONE', #4830, #8084 ) ;
#16093=FACE_OUTER_BOUND ( 'NONE', #12128, .T. ) ;
#16100=CARTESIAN_POINT ( 'NONE',  ( 218.9501057104153006, 10.79679952989121716, -16.84132998195102360 ) ) ;
#16101=LINE ( 'NONE', #1567, #15965 ) ;
#16103=EDGE_LOOP ( 'NONE', ( #4747, #13284, #9092, #10520 ) ) ;
#16104=ORIENTED_EDGE ( 'NONE', *, *, #17565, .T. ) ;
#16113=CARTESIAN_POINT ( 'NONE',  ( 201.7914626300884890, 0.3750460896586316206, -22.62267072728657524 ) ) ;
#16114=CIRCLE ( 'NONE', #14085, 11.94520687646042667 ) ;
#16118=LINE ( 'NONE', #8025, #1085 ) ;
#16120=DIRECTION ( 'NONE',  ( 0.5000000000000055511, -0.8660254037844353769, 1.110223024625156417E-16 ) ) ;
#16127=EDGE_CURVE ( 'NONE', #7288, #10818, #15776, .T. ) ;
#16129=AXIS2_PLACEMENT_3D ( 'NONE', #11661, #3692, #2014 ) ;
#16134=LINE ( 'NONE', #13149, #11710 ) ;
#16137=VERTEX_POINT ( 'NONE', #4522 ) ;
#16139=PLANE ( 'NONE',  #20932 ) ;
#16142=AXIS2_PLACEMENT_3D ( 'NONE', #10443, #5674, #20106 ) ;
#16144=DIRECTION ( 'NONE',  ( 0.8660254037844357100, 0.5000000000000052180, 0.000000000000000000 ) ) ;
#16146=EDGE_CURVE ( 'NONE', #9864, #18037, #20415, .T. ) ;
#16148=DIRECTION ( 'NONE',  ( -0.8660254037844358210, -0.5000000000000049960, 0.000000000000000000 ) ) ;
#16149=CARTESIAN_POINT ( 'NONE',  ( 198.0096515360099261, -1.293177324654909643, -12.56699194733486280 ) ) ;
#16156=ORIENTED_EDGE ( 'NONE', *, *, #19650, .F. ) ;
#16158=DIRECTION ( 'NONE',  ( 0.8645602258681719388, 0.4991540791356394169, 0.05814482891046558050 ) ) ;
#16159=PRODUCT_DEFINITION_CONTEXT ( 'detailed design', #1206, 'design' ) ;
#16161=EDGE_CURVE ( 'NONE', #9686, #8683, #7662, .T. ) ;
#16166=ORIENTED_EDGE ( 'NONE', *, *, #3686, .T. ) ;
#16167=LINE ( 'NONE', #19430, #10549 ) ;
#16168=ADVANCED_FACE ( 'NONE', ( #7584 ), #2833, .F. ) ;
#16170=VECTOR ( 'NONE', #13681, 1000.000000000000227 ) ;
#16172=ORIENTED_EDGE ( 'NONE', *, *, #277, .F. ) ;
#16174=VECTOR ( 'NONE', #20608, 1000.000000000000227 ) ;
#16175=DIRECTION ( 'NONE',  ( -0.5000000000000049960, 0.8660254037844358210, -0.000000000000000000 ) ) ;
#16178=EDGE_CURVE ( 'NONE', #2244, #12371, #160, .T. ) ;
#16187=CIRCLE ( 'NONE', #2309, 12.47473710546057823 ) ;
#16189=CARTESIAN_POINT ( 'NONE',  ( 201.5034618240616453, 7.454766308978539868, -25.15316579317382306 ) ) ;
#16190=ORIENTED_EDGE ( 'NONE', *, *, #15143, .F. ) ;
#16193=DIRECTION ( 'NONE',  ( -0.5000000000000049960, 0.8660254037844358210, -0.000000000000000000 ) ) ;
#16204=CARTESIAN_POINT ( 'NONE',  ( 195.0230325291159090, 3.359249353468287680, -14.01558723443171850 ) ) ;
#16210=DIRECTION ( 'NONE',  ( 0.5000000000000049960, -0.8660254037844358210, 0.000000000000000000 ) ) ;
#16215=CARTESIAN_POINT ( 'NONE',  ( 203.4811056270561664, 23.51224104295614481, -25.46066938576263894 ) ) ;
#16221=DIRECTION ( 'NONE',  ( -2.645739781067712995E-16, -1.527518574805166670E-16, -1.000000000000000000 ) ) ;
#16223=EDGE_CURVE ( 'NONE', #5368, #3353, #11190, .T. ) ;
#16227=EDGE_LOOP ( 'NONE', ( #15265, #6480, #4296, #16027 ) ) ;
#16229=FACE_OUTER_BOUND ( 'NONE', #2910, .T. ) ;
#16230=CARTESIAN_POINT ( 'NONE',  ( 194.9478548255267754, 18.58556639563049018, -25.46066938576250038 ) ) ;
#16231=EDGE_CURVE ( 'NONE', #3522, #14639, #11747, .T. ) ;
#16232=AXIS2_PLACEMENT_3D ( 'NONE', #7374, #12284, #7175 ) ;
#16233=EDGE_CURVE ( 'NONE', #14889, #12331, #17669, .T. ) ;
#16234=CARTESIAN_POINT ( 'NONE',  ( 215.9040783327276358, 15.94597603093701466, -15.40420431385954281 ) ) ;
#16239=VERTEX_POINT ( 'NONE', #18075 ) ;
#16241=CARTESIAN_POINT ( 'NONE',  ( 215.7530533430368394, 15.85878171248467439, -16.01416015924714742 ) ) ;
#16244=DIRECTION ( 'NONE',  ( 0.5000000000000051070, -0.8660254037844359321, 0.000000000000000000 ) ) ;
#16247=ORIENTED_EDGE ( 'NONE', *, *, #20624, .F. ) ;
#16249=VECTOR ( 'NONE', #18475, 1000.000000000000227 ) ;
#16251=ORIENTED_EDGE ( 'NONE', *, *, #7828, .T. ) ;
#16252=EDGE_CURVE ( 'NONE', #17368, #2011, #3603, .T. ) ;
#16253=VECTOR ( 'NONE', #1873, 1000.000000000000114 ) ;
#16259=CARTESIAN_POINT ( 'NONE',  ( 205.0662616026534693, 10.91332106064940888, -14.00000000000005507 ) ) ;
#16275=VECTOR ( 'NONE', #10244, 1000.000000000000227 ) ;
#16286=EDGE_CURVE ( 'NONE', #15417, #6104, #20865, .T. ) ;
#16288=EDGE_CURVE ( 'NONE', #2452, #15788, #16473, .T. ) ;
#16289=CIRCLE ( 'NONE', #7133, 11.94520687646042667 ) ;
#16290=EDGE_LOOP ( 'NONE', ( #3661, #8728, #3874, #13030 ) ) ;
#16297=DIRECTION ( 'NONE',  ( 0.8660254037844355990, 0.5000000000000054401, 8.899770914925154148E-15 ) ) ;
#16298=EDGE_CURVE ( 'NONE', #15249, #15363, #1831, .T. ) ;
#16299=ORIENTED_EDGE ( 'NONE', *, *, #7824, .F. ) ;
#16302=LINE ( 'NONE', #19673, #1728 ) ;
#16303=AXIS2_PLACEMENT_3D ( 'NONE', #14075, #19145, #4619 ) ;
#16306=CIRCLE ( 'NONE', #5783, 1.000000000000000888 ) ;
#16308=ORIENTED_EDGE ( 'NONE', *, *, #8622, .T. ) ;
#16310=DIRECTION ( 'NONE',  ( 0.5000000000000054401, -0.8660254037844353769, 3.330669073875469128E-16 ) ) ;
#16312=LINE ( 'NONE', #11325, #6291 ) ;
#16314=EDGE_CURVE ( 'NONE', #12179, #10014, #14242, .T. ) ;
#16315=VERTEX_POINT ( 'NONE', #260 ) ;
#16319=EDGE_CURVE ( 'NONE', #20139, #9718, #10095, .T. ) ;
#16320=AXIS2_PLACEMENT_3D ( 'NONE', #16696, #8522, #15022 ) ;
#16321=CONICAL_SURFACE ( 'NONE', #20034, 13.07248899748297433, 0.6693469023067423196 ) ;
#16322=CARTESIAN_POINT ( 'NONE',  ( 210.0930887352476759, 12.05995036078138583, -25.46066938576263894 ) ) ;
#16326=DIRECTION ( 'NONE',  ( -0.5000000000000049960, 0.8660254037844357100, -0.000000000000000000 ) ) ;
#16327=LINE ( 'NONE', #4869, #5534 ) ;
#16331=CARTESIAN_POINT ( 'NONE',  ( 218.9129779831750682, 10.51775681150463448, -11.19970074074921662 ) ) ;
#16338=VERTEX_POINT ( 'NONE', #2070 ) ;
#16342=FACE_OUTER_BOUND ( 'NONE', #12115, .T. ) ;
#16343=DIRECTION ( 'NONE',  ( 0.9679941405060890069, 0.000000000000000000, -0.2509727952306343712 ) ) ;
#16344=DIRECTION ( 'NONE',  ( -0.8660254037844355990, -0.5000000000000054401, -1.154189040529355901E-14 ) ) ;
#16348=ADVANCED_FACE ( 'NONE', ( #12032 ), #11928, .T. ) ;
#16350=DIRECTION ( 'NONE',  ( -0.5000000000000049960, 0.8660254037844358210, -0.000000000000000000 ) ) ;
#16351=CARTESIAN_POINT ( 'NONE',  ( 205.8264633344831225, 9.596613037118636669, -14.00000000000005507 ) ) ;
#16355=DIRECTION ( 'NONE',  ( 0.8660254037844352659, 0.5000000000000056621, 0.000000000000000000 ) ) ;
#16367=CARTESIAN_POINT ( 'NONE',  ( 195.4369152048313367, 3.952243985314471075, -11.19512133156234057 ) ) ;
#16376=CARTESIAN_POINT ( 'NONE',  ( 203.9371734008334158, 8.505830985348726614, -1.717498466822810599 ) ) ;
#16381=ADVANCED_FACE ( 'NONE', ( #16584 ), #15338, .F. ) ;
#16382=DIRECTION ( 'NONE',  ( -0.8660254037844349329, -0.5000000000000064393, 0.000000000000000000 ) ) ;
#16384=CARTESIAN_POINT ( 'NONE',  ( 208.8107687779841228, 4.427644383670616079, -14.00000000000005507 ) ) ;
#16385=FACE_OUTER_BOUND ( 'NONE', #17111, .T. ) ;
#16388=AXIS2_PLACEMENT_3D ( 'NONE', #19213, #13063, #16148 ) ;
#16399=CARTESIAN_POINT ( 'NONE',  ( 207.8872982515397609, 15.44148381043179263, -24.85758746085098991 ) ) ;
#16400=LINE ( 'NONE', #599, #18796 ) ;
#16402=ORIENTED_EDGE ( 'NONE', *, *, #13702, .F. ) ;
#16404=AXIS2_PLACEMENT_3D ( 'NONE', #8737, #18181, #10421 ) ;
#16415=CARTESIAN_POINT ( 'NONE',  ( 199.3871399495608898, 6.055890627870659237, -23.87887634647626101 ) ) ;
#16416=EDGE_CURVE ( 'NONE', #2244, #19879, #15161, .T. ) ;
#16419=CIRCLE ( 'NONE', #15422, 12.47473710546057823 ) ;
#16423=CARTESIAN_POINT ( 'NONE',  ( 206.3644977982345665, 10.08427006003479853, -1.709088388254546675 ) ) ;
#16426=DIRECTION ( 'NONE',  ( -0.5000000000000049960, 0.8660254037844357100, -0.000000000000000000 ) ) ;
#16429=ORIENTED_EDGE ( 'NONE', *, *, #5574, .T. ) ;
#16430=CARTESIAN_POINT ( 'NONE',  ( 208.0983737146324870, 5.661548828456886895, -14.00000000000005507 ) ) ;
#16432=ADVANCED_FACE ( 'NONE', ( #20390 ), #19197, .F. ) ;
#16438=CARTESIAN_POINT ( 'NONE',  ( 192.7356731787757838, 6.693688996011149861, -17.08769543353810505 ) ) ;
#16439=FACE_OUTER_BOUND ( 'NONE', #16742, .T. ) ;
#16442=CARTESIAN_POINT ( 'NONE',  ( 212.8872982515398178, 6.781229772587438198, -24.85758746085098991 ) ) ;
#16445=ORIENTED_EDGE ( 'NONE', *, *, #5574, .F. ) ;
#16446=CARTESIAN_POINT ( 'NONE',  ( 199.5603494194345444, -0.9130877231049959741, -19.34736286182874565 ) ) ;
#16450=ORIENTED_EDGE ( 'NONE', *, *, #7784, .F. ) ;
#16451=VERTEX_POINT ( 'NONE', #14346 ) ;
#16455=DIRECTION ( 'NONE',  ( -0.8660254037844358210, -0.5000000000000049960, 0.000000000000000000 ) ) ;
#16459=CIRCLE ( 'NONE', #6961, 1.000000000000000888 ) ;
#16467=EDGE_CURVE ( 'NONE', #2710, #4917, #4670, .T. ) ;
#16469=VERTEX_POINT ( 'NONE', #4572 ) ;
#16470=AXIS2_PLACEMENT_3D ( 'NONE', #4802, #11166, #16455 ) ;
#16471=PLANE ( 'NONE',  #15916 ) ;
#16473=CIRCLE ( 'NONE', #19851, 7.960520131757803597 ) ;
#16476=ORIENTED_EDGE ( 'NONE', *, *, #11982, .T. ) ;
#16483=LINE ( 'NONE', #7722, #7585 ) ;
#16489=ORIENTED_EDGE ( 'NONE', *, *, #19902, .T. ) ;
#16490=ADVANCED_FACE ( 'NONE', ( #4772 ), #8942, .F. ) ;
#16497=B_SPLINE_CURVE_WITH_KNOTS ( 'NONE', 3,
 ( #17706, #17800, #9825, #9623 ),
 .UNSPECIFIED., .F., .F.,
 ( 4, 4 ),
 ( 8.322893307755415259E-06, 0.0004399335472996286221 ),
 .UNSPECIFIED. ) ;
#16500=EDGE_LOOP ( 'NONE', ( #3247, #4854, #14177, #20485 ) ) ;
#16501=DIRECTION ( 'NONE',  ( 0.5566703992264085965, 0.3213938048432680161, -0.7660444431189865622 ) ) ;
#16507=AXIS2_PLACEMENT_3D ( 'NONE', #12382, #17563, #1030 ) ;
#16511=DIRECTION ( 'NONE',  ( -0.5000000000000051070, 0.8660254037844359321, -0.000000000000000000 ) ) ;
#16512=VERTEX_POINT ( 'NONE', #10526 ) ;
#16517=ORIENTED_EDGE ( 'NONE', *, *, #210, .F. ) ;
#16521=DIRECTION ( 'NONE',  ( -0.5000000000000051070, 0.8660254037844359321, -0.000000000000000000 ) ) ;
#16524=AXIS2_PLACEMENT_3D ( 'NONE', #19744, #8190, #11486 ) ;
#16532=ORIENTED_EDGE ( 'NONE', *, *, #6302, .T. ) ;
#16533=CARTESIAN_POINT ( 'NONE',  ( 208.5538622303137686, 11.70232678560638462, -2.669358488461177625 ) ) ;
#16537=FACE_OUTER_BOUND ( 'NONE', #9702, .T. ) ;
#16538=ORIENTED_EDGE ( 'NONE', *, *, #20645, .T. ) ;
#16543=CARTESIAN_POINT ( 'NONE',  ( 198.1209940990830205, -1.744099904769494280, -9.448537646917499089 ) ) ;
#16544=DIRECTION ( 'NONE',  ( 0.5000000000000054401, -0.8660254037844354880, 0.000000000000000000 ) ) ;
#16546=EDGE_CURVE ( 'NONE', #4987, #7633, #5176, .T. ) ;
#16549=FACE_OUTER_BOUND ( 'NONE', #10302, .T. ) ;
#16550=CARTESIAN_POINT ( 'NONE',  ( 215.8997106868019387, 9.293266993639628382, -23.06309126349817618 ) ) ;
#16551=AXIS2_PLACEMENT_3D ( 'NONE', #18699, #9037, #2595 ) ;
#16556=CYLINDRICAL_SURFACE ( 'NONE', #1399, 12.47473710546057646 ) ;
#16564=AXIS2_PLACEMENT_3D ( 'NONE', #8668, #5362, #18318 ) ;
#16569=CARTESIAN_POINT ( 'NONE',  ( 205.3906008270068071, 3.225829587143459243, -2.044871543906942701 ) ) ;
#16570=VERTEX_POINT ( 'NONE', #317 ) ;
#16584=FACE_OUTER_BOUND ( 'NONE', #1774, .T. ) ;
#16585=CARTESIAN_POINT ( 'NONE',  ( 194.8942117681098125, 18.53182819120163671, -14.00000000000005507 ) ) ;
#16588=CARTESIAN_POINT ( 'NONE',  ( 203.0627220339503936, 1.881828139331499727, -24.79563718815128226 ) ) ;
#16589=ORIENTED_EDGE ( 'NONE', *, *, #11493, .T. ) ;
#16597=CARTESIAN_POINT ( 'NONE',  ( 212.7427532632225962, 7.470596775315875071, -25.46066938576263894 ) ) ;
#16598=DIRECTION ( 'NONE',  ( 0.6299240516454601702, 0.3636868207865310287, 0.6862416378687270502 ) ) ;
#16605=CARTESIAN_POINT ( 'NONE',  ( 218.5362608324210782, 10.04265983930142347, -9.928836400542515150 ) ) ;
#16606=VECTOR ( 'NONE', #2532, 1000.000000000000227 ) ;
#16607=FACE_OUTER_BOUND ( 'NONE', #5740, .T. ) ;
#16609=ORIENTED_EDGE ( 'NONE', *, *, #1587, .F. ) ;
#16611=CARTESIAN_POINT ( 'NONE',  ( 193.6293134455680445, 7.209632444602317669, -12.64773574313024085 ) ) ;
#16613=CARTESIAN_POINT ( 'NONE',  ( 197.0442994948038233, 5.057277642004744500, -20.52105855319921091 ) ) ;
#16617=CARTESIAN_POINT ( 'NONE',  ( 201.7640869814541134, 0.3592407515502875626, -5.407152407593845744 ) ) ;
#16636=ORIENTED_EDGE ( 'NONE', *, *, #16792, .T. ) ;
#16638=FACE_OUTER_BOUND ( 'NONE', #11008, .T. ) ;
#16639=CARTESIAN_POINT ( 'NONE',  ( 194.2655634166889342, 7.576971536700876086, -21.18305361806748977 ) ) ;
#16640=ADVANCED_FACE ( 'NONE', ( #16537 ), #10369, .T. ) ;
#16641=AXIS2_PLACEMENT_3D ( 'NONE', #12162, #1238, #18625 ) ;
#16644=VECTOR ( 'NONE', #10163, 999.9999999999998863 ) ;
#16647=CARTESIAN_POINT ( 'NONE',  ( 214.2742449478047604, 15.00499128741754262, -7.425127016398544555 ) ) ;
#16650=CARTESIAN_POINT ( 'NONE',  ( 208.1960812450810465, 4.072754371081482638, -0.8632678296711639998 ) ) ;
#16651=EDGE_CURVE ( 'NONE', #16570, #19425, #2129, .T. ) ;
#16654=FACE_OUTER_BOUND ( 'NONE', #1386, .T. ) ;
#16657=DIRECTION ( 'NONE',  ( -0.8660254037844357100, -0.5000000000000051070, 0.000000000000000000 ) ) ;
#16668=ORIENTED_EDGE ( 'NONE', *, *, #13837, .T. ) ;
#16671=FACE_OUTER_BOUND ( 'NONE', #8600, .T. ) ;
#16684=CARTESIAN_POINT ( 'NONE',  ( 214.9458835816058979, 7.969754567050957306, -23.47937149798938350 ) ) ;
#16686=DIRECTION ( 'NONE',  ( -0.6299240516454601702, -0.3636868207865310287, -0.6862416378687270502 ) ) ;
#16696=CARTESIAN_POINT ( 'NONE',  ( 209.5488276859553594, 16.40076827665816239, -25.36561010639692881 ) ) ;
#16699=EDGE_CURVE ( 'NONE', #18617, #17439, #4131, .T. ) ;
#16704=ORIENTED_EDGE ( 'NONE', *, *, #13807, .F. ) ;
#16712=CARTESIAN_POINT ( 'NONE',  ( 213.3216307924363946, 4.537449897911132624, -14.00000000000005507 ) ) ;
#16717=ORIENTED_EDGE ( 'NONE', *, *, #13583, .T. ) ;
#16719=FACE_OUTER_BOUND ( 'NONE', #2429, .T. ) ;
#16721=ORIENTED_EDGE ( 'NONE', *, *, #9668, .F. ) ;
#16733=CARTESIAN_POINT ( 'NONE',  ( 199.0679134205424816, -0.6821895407469270589, -8.485309299592096011 ) ) ;
#16736=PLANE ( 'NONE',  #8667 ) ;
#16739=VERTEX_POINT ( 'NONE', #2548 ) ;
#16741=EDGE_LOOP ( 'NONE', ( #704, #17145, #16979, #13075, #9431, #13966 ) ) ;
#16742=EDGE_LOOP ( 'NONE', ( #7083, #11278, #11792, #5541 ) ) ;
#16744=LINE ( 'NONE', #8889, #19822 ) ;
#16745=EDGE_LOOP ( 'NONE', ( #11491, #479, #20259, #3106 ) ) ;
#16754=CARTESIAN_POINT ( 'NONE',  ( 205.8264633344831225, 9.596613037118636669, -14.00000000000005507 ) ) ;
#16755=CARTESIAN_POINT ( 'NONE',  ( 207.5960625376490043, 10.79531429386019958, -26.12540443289073977 ) ) ;
#16756=ADVANCED_FACE ( 'NONE', ( #20030 ), #18442, .F. ) ;
#16757=ORIENTED_EDGE ( 'NONE', *, *, #2821, .F. ) ;
#16759=CARTESIAN_POINT ( 'NONE',  ( 208.4761278624580711, 5.007259451653140125, -14.00000000000005507 ) ) ;
#16760=DIRECTION ( 'NONE',  ( 0.5000000000000054401, -0.8660254037844354880, 0.000000000000000000 ) ) ;
#16761=EDGE_CURVE ( 'NONE', #13251, #9080, #8919, .T. ) ;
#16768=EDGE_LOOP ( 'NONE', ( #19177, #17638, #8264, #9456, #20495, #12461 ) ) ;
#16770=PRODUCT_CONTEXT ( 'NONE', #20813, 'mechanical' ) ;
#16774=CARTESIAN_POINT ( 'NONE',  ( 209.8909370991932519, 2.556737970610027499, -14.00000000000005507 ) ) ;
#16776=CARTESIAN_POINT ( 'NONE',  ( 216.6737232845935068, 8.967323284687328311, -21.59012016402729728 ) ) ;
#16777=CARTESIAN_POINT ( 'NONE',  ( 201.5545410371157118, 7.661266810568780450, -3.125199447383423035 ) ) ;
#16780=VERTEX_POINT ( 'NONE', #2439 ) ;
#16782=CARTESIAN_POINT ( 'NONE',  ( 210.6201421056092897, 5.472286561439484665, -25.76107385416583639 ) ) ;
#16784=DIRECTION ( 'NONE',  ( 0.9949159024423646080, 0.000000000000000000, -0.1007092203688184640 ) ) ;
#16787=CYLINDRICAL_SURFACE ( 'NONE', #9466, 12.47473710546057646 ) ;
#16788=DIRECTION ( 'NONE',  ( -0.5000000000000054401, 0.8660254037844354880, -0.000000000000000000 ) ) ;
#16792=EDGE_CURVE ( 'NONE', #10058, #6217, #846, .T. ) ;
#16794=ORIENTED_EDGE ( 'NONE', *, *, #12388, .T. ) ;
#16796=CONICAL_SURFACE ( 'NONE', #6615, 13.07248899748297433, 0.6693469023067423196 ) ;
#16797=PLANE ( 'NONE',  #9886 ) ;
#16803=CARTESIAN_POINT ( 'NONE',  ( 198.7417246237710913, -1.385720969246587497, -16.73990883341915037 ) ) ;
#16808=PLANE ( 'NONE',  #20165 ) ;
#16813=CARTESIAN_POINT ( 'NONE',  ( 219.2795586678252562, 11.24462313530347757, -14.01558723443205068 ) ) ;
#16815=DIRECTION ( 'NONE',  ( -0.5000000000000049960, 0.8660254037844357100, -0.000000000000000000 ) ) ;
#16819=ORIENTED_EDGE ( 'NONE', *, *, #2933, .F. ) ;
#16823=CARTESIAN_POINT ( 'NONE',  ( 214.0136128684463301, 18.97851320364322447, -8.145074743996646660 ) ) ;
#16826=CARTESIAN_POINT ( 'NONE',  ( 195.2234364649848999, 3.828991977397862900, -12.59311507501989702 ) ) ;
#16828=LINE ( 'NONE', #18309, #9996 ) ;
#16834=CARTESIAN_POINT ( 'NONE',  ( 199.3181527907504744, -1.052920011872564343, -6.724618537539361895 ) ) ;
#16836=FACE_OUTER_BOUND ( 'NONE', #4643, .T. ) ;
#16837=ORIENTED_EDGE ( 'NONE', *, *, #11677, .T. ) ;
#16844=VECTOR ( 'NONE', #7403, 1000.000000000000114 ) ;
#16845=VERTEX_POINT ( 'NONE', #18764 ) ;
#16848=DIRECTION ( 'NONE',  ( -0.8660254037844363761, -0.5000000000000037748, 0.000000000000000000 ) ) ;
#16849=CARTESIAN_POINT ( 'NONE',  ( 217.5096804110553137, 10.22278344732445809, -20.84195174293596153 ) ) ;
#16851=ORIENTED_EDGE ( 'NONE', *, *, #8104, .T. ) ;
#16853=B_SPLINE_CURVE_WITH_KNOTS ( 'NONE', 3,
 ( #19488, #16331, #8249, #10580 ),
 .UNSPECIFIED., .F., .F.,
 ( 4, 4 ),
 ( 5.589689327475942692E-05, 0.0009098826312574273935 ),
 .UNSPECIFIED. ) ;
#16861=PLANE ( 'NONE',  #4921 ) ;
#16878=ORIENTED_EDGE ( 'NONE', *, *, #2234, .F. ) ;
#16880=ADVANCED_FACE ( 'NONE', ( #12825 ), #7337, .T. ) ;
#16883=CARTESIAN_POINT ( 'NONE',  ( 214.0593366061550569, 19.00491181591769418, -13.97827067520052324 ) ) ;
#16887=CARTESIAN_POINT ( 'NONE',  ( 208.0983737146324870, 5.661548828456886895, -14.00000000000005507 ) ) ;
#16889=VERTEX_POINT ( 'NONE', #16113 ) ;
#16892=CARTESIAN_POINT ( 'NONE',  ( 196.1782232529825762, 4.026199028858075124, -19.61257667712936126 ) ) ;
#16898=CARTESIAN_POINT ( 'NONE',  ( 204.4254563108872844, 13.44278843410413771, -0.8632678296711639998 ) ) ;
#16899=CARTESIAN_POINT ( 'NONE',  ( 202.6391622872795324, 8.287473181319668925, -2.669358488461094581 ) ) ;
#16901=EDGE_CURVE ( 'NONE', #18151, #15334, #18969, .T. ) ;
#16907=CARTESIAN_POINT ( 'NONE',  ( 217.4610193877672941, 9.421868901786666584, -7.448751785191543462 ) ) ;
#16908=B_SPLINE_CURVE_WITH_KNOTS ( 'NONE', 3,
 ( #1471, #14528, #8017, #12821 ),
 .UNSPECIFIED., .F., .F.,
 ( 4, 4 ),
 ( 0.0003733324143565315990, 0.0006786237464731411642 ),
 .UNSPECIFIED. ) ;
#16919=FACE_OUTER_BOUND ( 'NONE', #8505, .T. ) ;
#16920=CARTESIAN_POINT ( 'NONE',  ( 196.9688168050317643, 9.137695608148359128, -3.480441514389557955 ) ) ;
#16922=ORIENTED_EDGE ( 'NONE', *, *, #1006, .T. ) ;
#16923=ORIENTED_EDGE ( 'NONE', *, *, #6210, .F. ) ;
#16927=CARTESIAN_POINT ( 'NONE',  ( 214.9383172013976093, 8.738206206044257129, -4.003039906354144861 ) ) ;
#16929=CARTESIAN_POINT ( 'NONE',  ( 208.8127379954726166, 11.49776219695108814, -25.79243801023037008 ) ) ;
#16939=CARTESIAN_POINT ( 'NONE',  ( 209.3878836909736663, 4.760841834038437526, -25.81526893633800412 ) ) ;
#16940=EDGE_CURVE ( 'NONE', #600, #14158, #9513, .T. ) ;
#16941=DIRECTION ( 'NONE',  ( 0.5000000000000054401, -0.8660254037844354880, 0.000000000000000000 ) ) ;
#16943=ORIENTED_EDGE ( 'NONE', *, *, #5399, .T. ) ;
#16949=ORIENTED_EDGE ( 'NONE', *, *, #11663, .F. ) ;
#16952=FACE_OUTER_BOUND ( 'NONE', #14927, .T. ) ;
#16957=DIRECTION ( 'NONE',  ( -0.1005394128318080893, -0.05804645706261214733, 0.9932383577419439113 ) ) ;
#16962=AXIS2_PLACEMENT_3D ( 'NONE', #5940, #9026, #15526 ) ;
#16968=CARTESIAN_POINT ( 'NONE',  ( 219.0841311483638947, 10.35897291369198747, -15.40190399002830723 ) ) ;
#16969=LINE ( 'NONE', #14010, #9986 ) ;
#16973=CARTESIAN_POINT ( 'NONE',  ( 202.4338800647615528, 1.003545192306245282, -4.273921076953224762 ) ) ;
#16979=ORIENTED_EDGE ( 'NONE', *, *, #4244, .F. ) ;
#16980=CARTESIAN_POINT ( 'NONE',  ( 217.4465006036304260, 9.413486477856961798, -20.57673792763531040 ) ) ;
#16981=DIRECTION ( 'NONE',  ( 0.5000000000000051070, -0.8660254037844359321, 0.000000000000000000 ) ) ;
#16993=CARTESIAN_POINT ( 'NONE',  ( 199.2144802262915846, 21.04890371929339921, -14.00000000000005507 ) ) ;
#16994=CONICAL_SURFACE ( 'NONE', #3107, 10.85470691220533190, 0.8171114040043576665 ) ;
#16995=AXIS2_PLACEMENT_3D ( 'NONE', #16259, #4704, #11175 ) ;
#16996=VECTOR ( 'NONE', #14428, 1000.000000000000114 ) ;
#16997=CARTESIAN_POINT ( 'NONE',  ( 208.0983737146324870, 5.661548828456886895, -14.00000000000005507 ) ) ;
#17003=EDGE_CURVE ( 'NONE', #14589, #3522, #552, .T. ) ;
#17014=DIRECTION ( 'NONE',  ( -0.9885408208161388099, 0.000000000000000000, -0.1509537862398780406 ) ) ;
#17016=PLANE ( 'NONE',  #12358 ) ;
#17019=EDGE_CURVE ( 'NONE', #11314, #1051, #8232, .T. ) ;
#17021=DIRECTION ( 'NONE',  ( -0.9170191824714367668, 0.000000000000000000, 0.3988431007042967935 ) ) ;
#17023=CARTESIAN_POINT ( 'NONE',  ( 209.1514512894396489, 12.04734498975750512, -15.55037597655807069 ) ) ;
#17033=VERTEX_POINT ( 'NONE', #13132 ) ;
#17036=ORIENTED_EDGE ( 'NONE', *, *, #14220, .F. ) ;
#17038=ORIENTED_EDGE ( 'NONE', *, *, #3165, .T. ) ;
#17042=CARTESIAN_POINT ( 'NONE',  ( 197.4175317442008577, -2.150244084725486005, -14.05525385477288047 ) ) ;
#17043=EDGE_CURVE ( 'NONE', #14727, #7529, #6533, .T. ) ;
#17049=CARTESIAN_POINT ( 'NONE',  ( 208.8107687779841228, 4.427644383670616079, -14.00000000000005507 ) ) ;
#17053=DIRECTION ( 'NONE',  ( -0.5000000000000054401, 0.8660254037844354880, -0.000000000000000000 ) ) ;
#17056=VERTEX_POINT ( 'NONE', #18008 ) ;
#17059=DIRECTION ( 'NONE',  ( -0.6946590618905487124, -0.4010615963775265858, -0.5971585917027844026 ) ) ;
#17061=VECTOR ( 'NONE', #3455, 1000.000000000000114 ) ;
#17063=ORIENTED_EDGE ( 'NONE', *, *, #16288, .T. ) ;
#17064=ORIENTED_EDGE ( 'NONE', *, *, #9017, .F. ) ;
#17068=ADVANCED_FACE ( 'NONE', ( #1994 ), #8341, .F. ) ;
#17069=ADVANCED_FACE ( 'NONE', ( #3477 ), #14945, .F. ) ;
#17071=ORIENTED_EDGE ( 'NONE', *, *, #16231, .T. ) ;
#17090=CARTESIAN_POINT ( 'NONE',  ( 205.8264633344831225, 9.596613037118636669, -14.00000000000005507 ) ) ;
#17097=LINE ( 'NONE', #18577, #8057 ) ;
#17101=CARTESIAN_POINT ( 'NONE',  ( 215.6932043811731603, 15.82422789824195242, -11.22353489230414958 ) ) ;
#17102=CIRCLE ( 'NONE', #5915, 12.47473710546057823 ) ;
#17104=ORIENTED_EDGE ( 'NONE', *, *, #18844, .F. ) ;
#17107=DIRECTION ( 'NONE',  ( 0.5000000000000057732, -0.8660254037844352659, -4.857225732735059248E-17 ) ) ;
#17111=EDGE_LOOP ( 'NONE', ( #10251, #1669, #2639, #16589 ) ) ;
#17115=DIRECTION ( 'NONE',  ( 0.1503837331804321054, 0.08682408883346430517, -0.9848077530122086864 ) ) ;
#17116=AXIS2_PLACEMENT_3D ( 'NONE', #4045, #12334, #2361 ) ;
#17117=DIRECTION ( 'NONE',  ( 0.6299240516454603922, 0.3636868207865314173, 0.6862416378687268281 ) ) ;
#17122=ORIENTED_EDGE ( 'NONE', *, *, #467, .T. ) ;
#17123=CARTESIAN_POINT ( 'NONE',  ( 195.9574494032261498, 8.553782366466350595, -23.53124788243903964 ) ) ;
#17128=LINE ( 'NONE', #13850, #13051 ) ;
#17129=CIRCLE ( 'NONE', #4268, 11.98469917212512215 ) ;
#17133=VECTOR ( 'NONE', #13456, 1000.000000000000114 ) ;
#17135=EDGE_CURVE ( 'NONE', #16137, #12179, #1279, .T. ) ;
#17137=EDGE_LOOP ( 'NONE', ( #579, #9020, #16794, #1942 ) ) ;
#17141=CARTESIAN_POINT ( 'NONE',  ( 211.9556053886519749, 4.903475301695560340, -14.00000000000005507 ) ) ;
#17142=FACE_OUTER_BOUND ( 'NONE', #11375, .T. ) ;
#17143=AXIS2_PLACEMENT_3D ( 'NONE', #8070, #19524, #17643 ) ;
#17145=ORIENTED_EDGE ( 'NONE', *, *, #4324, .F. ) ;
#17146=VECTOR ( 'NONE', #15259, 1000.000000000000227 ) ;
#17147=EDGE_CURVE ( 'NONE', #6174, #8299, #3326, .T. ) ;
#17149=CARTESIAN_POINT ( 'NONE',  ( 199.2144802262915846, 21.04890371929339921, -14.00000000000005507 ) ) ;
#17152=PLANE ( 'NONE',  #9454 ) ;
#17154=EDGE_CURVE ( 'NONE', #13693, #2710, #17755, .T. ) ;
#17157=CARTESIAN_POINT ( 'NONE',  ( 199.2144802262915846, 21.04890371929339921, -14.00000000000005507 ) ) ;
#17158=DIRECTION ( 'NONE',  ( -0.05035489893516277571, -0.02907241445523329332, 0.9983081582712688418 ) ) ;
#17161=AXIS2_PLACEMENT_3D ( 'NONE', #12843, #6148, #19098 ) ;
#17163=CARTESIAN_POINT ( 'NONE',  ( 216.7607129495440859, 9.790366881806683352, -5.993340328401894013 ) ) ;
#17167=ORIENTED_EDGE ( 'NONE', *, *, #15000, .F. ) ;
#17168=EDGE_CURVE ( 'NONE', #19498, #13379, #8878, .T. ) ;
#17169=ORIENTED_EDGE ( 'NONE', *, *, #10534, .T. ) ;
#17170=CARTESIAN_POINT ( 'NONE',  ( 215.9107784512153216, 15.77283444196598694, -16.79818413631500817 ) ) ;
#17171=ADVANCED_FACE ( 'NONE', ( #2412 ), #14836, .T. ) ;
#17175=B_SPLINE_CURVE_WITH_KNOTS ( 'NONE', 3,
 ( #7816, #17582, #12609, #17163 ),
 .UNSPECIFIED., .F., .F.,
 ( 4, 4 ),
 ( 4.835194380548316019E-05, 0.0009023376817886681828 ),
 .UNSPECIFIED. ) ;
#17177=CARTESIAN_POINT ( 'NONE',  ( 216.6495311407713871, 8.953355943939367734, -6.376588578941993823 ) ) ;
#17181=CARTESIAN_POINT ( 'NONE',  ( 216.5107763960967020, 15.86188268823392278, -14.01039157610429520 ) ) ;
#17184=EDGE_CURVE ( 'NONE', #3711, #16338, #13656, .T. ) ;
#17188=ORIENTED_EDGE ( 'NONE', *, *, #18168, .F. ) ;
#17189=CARTESIAN_POINT ( 'NONE',  ( 204.7342393044282289, 2.074058994753574581, -24.85758746085085846 ) ) ;
#17190=CARTESIAN_POINT ( 'NONE',  ( 196.8077463644258387, 4.389654366710942668, -7.132002368301173512 ) ) ;
#17194=FACE_OUTER_BOUND ( 'NONE', #17238, .T. ) ;
#17203=CARTESIAN_POINT ( 'NONE',  ( 205.5965122587965084, 9.994899983462953941, -14.00000000000005507 ) ) ;
#17207=ORIENTED_EDGE ( 'NONE', *, *, #11828, .T. ) ;
#17213=VERTEX_POINT ( 'NONE', #18421 ) ;
#17217=ORIENTED_EDGE ( 'NONE', *, *, #18350, .T. ) ;
#17220=AXIS2_PLACEMENT_3D ( 'NONE', #7118, #19840, #13708 ) ;
#17229=CARTESIAN_POINT ( 'NONE',  ( 198.7417246237710913, -1.385720969246587497, -16.73990883341915037 ) ) ;
#17231=CARTESIAN_POINT ( 'NONE',  ( 216.1256026380747244, 15.71984656690478310, -11.16670872502649914 ) ) ;
#17232=AXIS2_PLACEMENT_3D ( 'NONE', #20238, #17276, #2658 ) ;
#17233=ORIENTED_EDGE ( 'NONE', *, *, #3043, .F. ) ;
#17238=EDGE_LOOP ( 'NONE', ( #9223, #5707, #18490, #16609, #13293, #14314 ) ) ;
#17245=VERTEX_POINT ( 'NONE', #7173 ) ;
#17264=EDGE_CURVE ( 'NONE', #3323, #13300, #12955, .T. ) ;
#17274=CARTESIAN_POINT ( 'NONE',  ( 214.8766030929655813, 15.35276292467472103, -19.36714384557541990 ) ) ;
#17275=DIRECTION ( 'NONE',  ( 0.5000000000000049960, -0.8660254037844358210, 0.000000000000000000 ) ) ;
#17276=DIRECTION ( 'NONE',  ( -0.5000000000000049960, 0.8660254037844357100, -0.000000000000000000 ) ) ;
#17284=VECTOR ( 'NONE', #18484, 1000.000000000000114 ) ;
#17286=DIRECTION ( 'NONE',  ( -0.8296432542242747621, -0.4789947561577490021, 0.2868032327110942581 ) ) ;
#17287=ORIENTED_EDGE ( 'NONE', *, *, #13945, .F. ) ;
#17290=ADVANCED_FACE ( 'NONE', ( #4624 ), #2304, .T. ) ;
#17291=VERTEX_POINT ( 'NONE', #20620 ) ;
#17295=CARTESIAN_POINT ( 'NONE',  ( 201.0771824364471172, 22.12433534174682492, -26.28791492288521781 ) ) ;
#17297=VECTOR ( 'NONE', #5726, 1000.000000000000114 ) ;
#17301=ADVANCED_FACE ( 'NONE', ( #17142 ), #1144, .F. ) ;
#17305=CARTESIAN_POINT ( 'NONE',  ( 199.7342393044281437, 10.73431303259792813, -24.85758746085085491 ) ) ;
#17309=VECTOR ( 'NONE', #17286, 1000.000000000000114 ) ;
#17311=CARTESIAN_POINT ( 'NONE',  ( 216.5584123369822009, 15.79270668264091881, -15.43274561385901045 ) ) ;
#17315=AXIS2_PLACEMENT_3D ( 'NONE', #5845, #14147, #11151 ) ;
#17318=DIRECTION ( 'NONE',  ( 0.8660254037844373753, 0.5000000000000022204, 0.000000000000000000 ) ) ;
#17326=EDGE_CURVE ( 'NONE', #1522, #11167, #284, .T. ) ;
#17328=PLANE ( 'NONE',  #5618 ) ;
#17331=CIRCLE ( 'NONE', #12596, 12.47473710546057823 ) ;
#17333=DIRECTION ( 'NONE',  ( 0.5000000000000054401, -0.8660254037844354880, 0.000000000000000000 ) ) ;
#17341=FACE_OUTER_BOUND ( 'NONE', #2299, .T. ) ;
#17346=AXIS2_PLACEMENT_3D ( 'NONE', #2666, #7835, #9105 ) ;
#17351=ORIENTED_EDGE ( 'NONE', *, *, #6392, .T. ) ;
#17352=ORIENTED_EDGE ( 'NONE', *, *, #13049, .T. ) ;
#17360=DIRECTION ( 'NONE',  ( -0.5000000000000051070, 0.8660254037844355990, 0.000000000000000000 ) ) ;
#17361=AXIS2_PLACEMENT_3D ( 'NONE', #1926, #8589, #328 ) ;
#17362=VECTOR ( 'NONE', #13203, 1000.000000000000114 ) ;
#17367=CARTESIAN_POINT ( 'NONE',  ( 199.6607596192359608, -0.8551158672202783251, -8.669480444820576892 ) ) ;
#17368=VERTEX_POINT ( 'NONE', #11501 ) ;
#17370=ORIENTED_EDGE ( 'NONE', *, *, #11895, .F. ) ;
#17372=CARTESIAN_POINT ( 'NONE',  ( 205.8264633344831225, 9.596613037118636669, -14.00000000000005507 ) ) ;
#17374=VERTEX_POINT ( 'NONE', #17879 ) ;
#17380=ORIENTED_EDGE ( 'NONE', *, *, #5380, .F. ) ;
#17382=CARTESIAN_POINT ( 'NONE',  ( 208.0983737146324870, 5.661548828456886895, -14.00000000000005507 ) ) ;
#17383=DIRECTION ( 'NONE',  ( 0.5000000000000049960, -0.8660254037844358210, 0.000000000000000000 ) ) ;
#17384=FACE_OUTER_BOUND ( 'NONE', #9940, .T. ) ;
#17389=DIRECTION ( 'NONE',  ( -0.2483788854152945980, -0.1434016163555415502, 0.9579895123154918979 ) ) ;
#17394=DIRECTION ( 'NONE',  ( -0.5566703992264184775, -0.3213938048432737893, -0.7660444431189769032 ) ) ;
#17396=ORIENTED_EDGE ( 'NONE', *, *, #455, .F. ) ;
#17401=CARTESIAN_POINT ( 'NONE',  ( 211.7014381176568065, 13.51958057145868253, -4.494676796018852727 ) ) ;
#17404=VECTOR ( 'NONE', #17275, 1000.000000000000227 ) ;
#17412=EDGE_CURVE ( 'NONE', #11656, #20827, #3545, .T. ) ;
#17415=LINE ( 'NONE', #7753, #5852 ) ;
#17418=ORIENTED_EDGE ( 'NONE', *, *, #7441, .T. ) ;
#17420=CARTESIAN_POINT ( 'NONE',  ( 201.9636910742785005, 0.3660905863451732745, -14.00000000000005507 ) ) ;
#17423=CARTESIAN_POINT ( 'NONE',  ( 195.2889461848653525, 4.043823935988862139, -15.40420431385919464 ) ) ;
#17425=ORIENTED_EDGE ( 'NONE', *, *, #15805, .T. ) ;
#17428=CARTESIAN_POINT ( 'NONE',  ( 205.1848235957376403, 9.226162161231169279, -26.45271578590682893 ) ) ;
#17432=DIRECTION ( 'NONE',  ( -0.8660254037844355990, -0.5000000000000055511, 0.000000000000000000 ) ) ;
#17436=CARTESIAN_POINT ( 'NONE',  ( 195.6791760372415183, 3.738073984511642855, -9.718744748712971671 ) ) ;
#17439=VERTEX_POINT ( 'NONE', #12670 ) ;
#17440=PLANE ( 'NONE',  #18682 ) ;
#17441=DIRECTION ( 'NONE',  ( 0.8660254037844355990, 0.5000000000000054401, 0.000000000000000000 ) ) ;
#17448=LINE ( 'NONE', #1136, #8151 ) ;
#17449=ORIENTED_EDGE ( 'NONE', *, *, #12890, .T. ) ;
#17451=DIRECTION ( 'NONE',  ( -0.5000000000000051070, 0.8660254037844359321, -0.000000000000000000 ) ) ;
#17452=DIRECTION ( 'NONE',  ( 0.5000000000000052180, -0.8660254037844355990, -1.665334536937734071E-16 ) ) ;
#17455=DIRECTION ( 'NONE',  ( -1.060575238724903217E-16, -6.123233995736827666E-17, 1.000000000000000000 ) ) ;
#17456=CARTESIAN_POINT ( 'NONE',  ( 214.2619155600624481, 14.99787291208556539, -20.59651891138172530 ) ) ;
#17469=CARTESIAN_POINT ( 'NONE',  ( 215.4747034159835550, 15.16702704537912183, -19.61257667712965258 ) ) ;
#17474=DIRECTION ( 'NONE',  ( -0.6958540455341891695, 0.000000000000000000, 0.7181832268395738073 ) ) ;
#17475=CARTESIAN_POINT ( 'NONE',  ( 199.2144802262915846, 21.04890371929339921, -14.00000000000005507 ) ) ;
#17480=FACE_OUTER_BOUND ( 'NONE', #13307, .T. ) ;
#17484=VERTEX_POINT ( 'NONE', #7769 ) ;
#17490=CARTESIAN_POINT ( 'NONE',  ( 189.0579591095837202, 15.18503351853190608, -18.25196083293855054 ) ) ;
#17491=CARTESIAN_POINT ( 'NONE',  ( 200.4973105777688431, 11.17487243767204852, -26.58724934764007486 ) ) ;
#17493=DIRECTION ( 'NONE',  ( -0.5000000000000049960, 0.8660254037844357100, -0.000000000000000000 ) ) ;
#17495=CARTESIAN_POINT ( 'NONE',  ( 216.7268875047958829, 8.998017661532479394, -6.310089745291985963 ) ) ;
#17497=ORIENTED_EDGE ( 'NONE', *, *, #2209, .T. ) ;
#17498=DIRECTION ( 'NONE',  ( 0.5000000000000051070, -0.8660254037844359321, 0.000000000000000000 ) ) ;
#17499=DIRECTION ( 'NONE',  ( 0.7739085681710394793, 0.4468163201617139091, 0.4487991802004502873 ) ) ;
#17502=ORIENTED_EDGE ( 'NONE', *, *, #7537, .F. ) ;
#17504=ORIENTED_EDGE ( 'NONE', *, *, #20931, .F. ) ;
#17505=ORIENTED_EDGE ( 'NONE', *, *, #13250, .T. ) ;
#17509=CARTESIAN_POINT ( 'NONE',  ( 205.8363079006329883, 14.25734397923043772, -1.053683606938506045 ) ) ;
#17516=DIRECTION ( 'NONE',  ( -0.5000000000000051070, 0.8660254037844359321, -0.000000000000000000 ) ) ;
#17529=CARTESIAN_POINT ( 'NONE',  ( 213.8661528393178060, 8.119191822981960627, -3.188775577416895324 ) ) ;
#17530=ADVANCED_FACE ( 'NONE', ( #4185 ), #4601, .F. ) ;
#17543=SHAPE_REPRESENTATION_RELATIONSHIP ( 'NONE' , 'NONE' ,  #9759, #7549 ) ;
#17544=AXIS2_PLACEMENT_3D ( 'NONE', #18554, #7511, #20135 ) ;
#17547=DIRECTION ( 'NONE',  ( 0.7951984747223626027, 0.4591080534401424385, 0.3960797660391544017 ) ) ;
#17554=EDGE_CURVE ( 'NONE', #11821, #19224, #19990, .T. ) ;
#17557=AXIS2_PLACEMENT_3D ( 'NONE', #6353, #17726, #19203 ) ;
#17558=CARTESIAN_POINT ( 'NONE',  ( 208.8107687779841228, 4.427644383670616079, -14.00000000000005507 ) ) ;
#17559=CARTESIAN_POINT ( 'NONE',  ( 205.0042238655992719, 9.652942120212628652, -25.96516918080906677 ) ) ;
#17560=DIRECTION ( 'NONE',  ( 0.000000000000000000, -0.000000000000000000, -1.000000000000000000 ) ) ;
#17563=DIRECTION ( 'NONE',  ( 0.8528685319524385022, 0.4924038765061083955, -0.1736481776669415444 ) ) ;
#17565=EDGE_CURVE ( 'NONE', #5172, #3434, #19232, .T. ) ;
#17568=EDGE_LOOP ( 'NONE', ( #3001, #4426, #8278, #18254 ) ) ;
#17573=CARTESIAN_POINT ( 'NONE',  ( 199.6867264275208527, -0.3249176845898890664, -20.75355104716098964 ) ) ;
#17579=ADVANCED_FACE ( 'NONE', ( #14689 ), #145, .T. ) ;
#17582=CARTESIAN_POINT ( 'NONE',  ( 216.7381715613988433, 9.262131738456792718, -6.204501730076263932 ) ) ;
#17584=DIRECTION ( 'NONE',  ( -0.8660254037844355990, -0.5000000000000054401, -1.334965637238773043E-14 ) ) ;
#17586=DIRECTION ( 'NONE',  ( -0.8137976813493725814, -0.4698463103929604867, -0.3420201433256626622 ) ) ;
#17590=DIRECTION ( 'NONE',  ( -0.5566703992264184775, -0.3213938048432735117, -0.7660444431189770143 ) ) ;
#17593=EDGE_CURVE ( 'NONE', #18887, #844, #8183, .T. ) ;
#17601=CARTESIAN_POINT ( 'NONE',  ( 217.5692528822465306, 9.484357538959612199, -5.585956497640099272 ) ) ;
#17603=DIRECTION ( 'NONE',  ( -0.5000000000000049960, 0.8660254037844358210, 0.000000000000000000 ) ) ;
#17605=EDGE_LOOP ( 'NONE', ( #1371, #19877, #10757, #650 ) ) ;
#17610=ORIENTED_EDGE ( 'NONE', *, *, #12022, .F. ) ;
#17614=CARTESIAN_POINT ( 'NONE',  ( 202.3258709495397625, 22.84526599091486077, -25.94618751764496878 ) ) ;
#17617=EDGE_LOOP ( 'NONE', ( #18107, #18569, #14948, #9952 ) ) ;
#17621=CARTESIAN_POINT ( 'NONE',  ( 199.2144802262915846, 21.04890371929339921, -14.00000000000005507 ) ) ;
#17623=FACE_OUTER_BOUND ( 'NONE', #5759, .T. ) ;
#17626=CARTESIAN_POINT ( 'NONE',  ( 216.6737232845935068, 8.967323284687328311, -21.59012016402729728 ) ) ;
#17629=EDGE_LOOP ( 'NONE', ( #17449, #12242, #12847, #3611 ) ) ;
#17630=CARTESIAN_POINT ( 'NONE',  ( 195.4150569263803732, 4.116634006550261127, -12.64773574313024440 ) ) ;
#17638=ORIENTED_EDGE ( 'NONE', *, *, #20680, .F. ) ;
#17641=ORIENTED_EDGE ( 'NONE', *, *, #20728, .F. ) ;
#17643=DIRECTION ( 'NONE',  ( 0.8660254037844355990, 0.5000000000000054401, 0.000000000000000000 ) ) ;
#17649=CONICAL_SURFACE ( 'NONE', #15960, 10.85470691220533190, 0.8171114040043576665 ) ;
#17650=ORIENTED_EDGE ( 'NONE', *, *, #6938, .F. ) ;
#17652=DIRECTION ( 'NONE',  ( 0.6946590618905410519, 0.4010615963775224224, -0.5971585917027962820 ) ) ;
#17657=CARTESIAN_POINT ( 'NONE',  ( 210.5263754848605231, 5.675749601516248077, -25.93669565428271184 ) ) ;
#17660=ORIENTED_EDGE ( 'NONE', *, *, #20779, .F. ) ;
#17665=CIRCLE ( 'NONE', #11230, 11.94520687646042667 ) ;
#17666=VERTEX_POINT ( 'NONE', #3623 ) ;
#17667=CARTESIAN_POINT ( 'NONE',  ( 197.0455819868763570, 9.182016006550787424, -24.58554911381517627 ) ) ;
#17669=LINE ( 'NONE', #7894, #14140 ) ;
#17670=EDGE_CURVE ( 'NONE', #9756, #4589, #7375, .T. ) ;
#17675=FACE_OUTER_BOUND ( 'NONE', #5632, .T. ) ;
#17681=DIRECTION ( 'NONE',  ( 0.8660254037844377084, 0.5000000000000015543, 0.000000000000000000 ) ) ;
#17682=VECTOR ( 'NONE', #2112, 1000.000000000000000 ) ;
#17686=ORIENTED_EDGE ( 'NONE', *, *, #3179, .T. ) ;
#17688=DIRECTION ( 'NONE',  ( -0.8660254037844355990, -0.5000000000000054401, 1.070753688201932557E-14 ) ) ;
#17693=CARTESIAN_POINT ( 'NONE',  ( 211.6737232845934500, 17.62757732253168541, -21.59012016402730083 ) ) ;
#17695=ORIENTED_EDGE ( 'NONE', *, *, #14716, .F. ) ;
#17698=ORIENTED_EDGE ( 'NONE', *, *, #10967, .T. ) ;
#17701=EDGE_CURVE ( 'NONE', #2297, #18411, #6309, .T. ) ;
#17703=VECTOR ( 'NONE', #3241, 1000.000000000000227 ) ;
#17706=CARTESIAN_POINT ( 'NONE',  ( 197.6726970570908293, -1.230104231997219300, -14.01558723443171850 ) ) ;
#17709=DIRECTION ( 'NONE',  ( 0.5000000000000054401, -0.8660254037844354880, 0.000000000000000000 ) ) ;
#17713=CONICAL_SURFACE ( 'NONE', #4161, 10.85470691220533190, 0.8171114040043576665 ) ;
#17716=VERTEX_POINT ( 'NONE', #18998 ) ;
#17720=DIRECTION ( 'NONE',  ( -0.5000000000000049960, 0.8660254037844358210, -0.000000000000000000 ) ) ;
#17725=ORIENTED_EDGE ( 'NONE', *, *, #10434, .T. ) ;
#17726=DIRECTION ( 'NONE',  ( -0.5000000000000054401, 0.8660254037844354880, -0.000000000000000000 ) ) ;
#17727=DIRECTION ( 'NONE',  ( -0.5000000000000051070, 0.8660254037844359321, -0.000000000000000000 ) ) ;
#17731=PLANE ( 'NONE',  #14089 ) ;
#17736=FACE_OUTER_BOUND ( 'NONE', #1766, .T. ) ;
#17738=EDGE_LOOP ( 'NONE', ( #13120, #7576, #4799, #4254 ) ) ;
#17743=AXIS2_PLACEMENT_3D ( 'NONE', #5385, #534, #320 ) ;
#17744=CARTESIAN_POINT ( 'NONE',  ( 202.0139385235187035, 1.276312697262135920, -4.003039906353937916 ) ) ;
#17745=CIRCLE ( 'NONE', #3848, 4.730184897849355252 ) ;
#17746=ORIENTED_EDGE ( 'NONE', *, *, #9644, .F. ) ;
#17747=ORIENTED_EDGE ( 'NONE', *, *, #13268, .F. ) ;
#17754=AXIS2_PLACEMENT_3D ( 'NONE', #7143, #13315, #489 ) ;
#17755=B_SPLINE_CURVE_WITH_KNOTS ( 'NONE', 3,
 ( #10235, #3786, #16929, #20209 ),
 .UNSPECIFIED., .F., .F.,
 ( 4, 4 ),
 ( 8.047005770514206345E-05, 0.0007531208497576732160 ),
 .UNSPECIFIED. ) ;
#17758=ORIENTED_EDGE ( 'NONE', *, *, #12280, .F. ) ;
#17760=FACE_OUTER_BOUND ( 'NONE', #8602, .T. ) ;
#17763=CARTESIAN_POINT ( 'NONE',  ( 200.2088966793999987, 0.2341713026616738524, -22.03054070023845767 ) ) ;
#17766=AXIS2_PLACEMENT_3D ( 'NONE', #13840, #20286, #5751 ) ;
#17767=CARTESIAN_POINT ( 'NONE',  ( 209.3990796341988982, 4.767305814873403769, -25.92587471718750436 ) ) ;
#17771=CARTESIAN_POINT ( 'NONE',  ( 201.4752803508637271, 7.615505632025055149, -24.99940654434229970 ) ) ;
#17781=VERTEX_POINT ( 'NONE', #19105 ) ;
#17783=CARTESIAN_POINT ( 'NONE',  ( 202.3000072617431329, 22.83033358380322753, -2.044871543907030631 ) ) ;
#17787=ORIENTED_EDGE ( 'NONE', *, *, #14435, .F. ) ;
#17789=CARTESIAN_POINT ( 'NONE',  ( 214.4645575845060534, 14.93785843526373647, -7.327415643059550732 ) ) ;
#17790=DIRECTION ( 'NONE',  ( -0.8660254037844358210, -0.5000000000000049960, 0.000000000000000000 ) ) ;
#17793=EDGE_CURVE ( 'NONE', #13143, #10497, #8839, .T. ) ;
#17795=EDGE_CURVE ( 'NONE', #10818, #6868, #9119, .T. ) ;
#17799=LINE ( 'NONE', #11854, #11480 ) ;
#17800=CARTESIAN_POINT ( 'NONE',  ( 197.8063295462453652, -1.283151408128118565, -14.01039160325040989 ) ) ;
#17803=ORIENTED_EDGE ( 'NONE', *, *, #17841, .T. ) ;
#17807=AXIS2_PLACEMENT_3D ( 'NONE', #17141, #17455, #20619 ) ;
#17809=EDGE_CURVE ( 'NONE', #17666, #18042, #4001, .T. ) ;
#17810=ORIENTED_EDGE ( 'NONE', *, *, #10809, .F. ) ;
#17816=DIRECTION ( 'NONE',  ( -0.5000000000000054401, 0.8660254037844354880, -0.000000000000000000 ) ) ;
#17820=EDGE_CURVE ( 'NONE', #9718, #12634, #9432, .T. ) ;
#17822=ORIENTED_EDGE ( 'NONE', *, *, #5637, .T. ) ;
#17824=AXIS2_PLACEMENT_3D ( 'NONE', #3621, #11904, #13285 ) ;
#17831=CARTESIAN_POINT ( 'NONE',  ( 214.8858643771922630, 19.48210784701872811, -17.08769543353844611 ) ) ;
#17838=ORIENTED_EDGE ( 'NONE', *, *, #478, .F. ) ;
#17839=ORIENTED_EDGE ( 'NONE', *, *, #536, .F. ) ;
#17840=LINE ( 'NONE', #19721, #19972 ) ;
#17841=EDGE_CURVE ( 'NONE', #19523, #12371, #1634, .T. ) ;
#17843=MANIFOLD_SOLID_BREP ( 'Fillet5', #9965 ) ;
#17846=ORIENTED_EDGE ( 'NONE', *, *, #1537, .T. ) ;
#17861=EDGE_CURVE ( 'NONE', #15334, #10335, #9085, .T. ) ;
#17864=FACE_OUTER_BOUND ( 'NONE', #4678, .T. ) ;
#17867=EDGE_CURVE ( 'NONE', #1053, #8779, #12297, .T. ) ;
#17872=ORIENTED_EDGE ( 'NONE', *, *, #295, .F. ) ;
#17875=CARTESIAN_POINT ( 'NONE',  ( 208.8107687779840944, 4.427644383670621409, -14.00000000000005507 ) ) ;
#17879=CARTESIAN_POINT ( 'NONE',  ( 208.1960812450810465, 4.072754371081502178, -2.075899210536066963 ) ) ;
#17886=CARTESIAN_POINT ( 'NONE',  ( 209.7235900860870572, 27.11634112578974154, -16.89203719259520753 ) ) ;
#17889=LINE ( 'NONE', #14925, #19609 ) ;
#17892=AXIS2_PLACEMENT_3D ( 'NONE', #8922, #15418, #872 ) ;
#17899=DIRECTION ( 'NONE',  ( 0.8660254037844355990, 0.5000000000000054401, 0.000000000000000000 ) ) ;
#17901=DIRECTION ( 'NONE',  ( 0.8660254037844352659, 0.5000000000000056621, 0.000000000000000000 ) ) ;
#17905=VERTEX_POINT ( 'NONE', #1049 ) ;
#17907=CARTESIAN_POINT ( 'NONE',  ( 199.3859296228393134, 5.878169164976177363, -24.01557619556968248 ) ) ;
#17911=CARTESIAN_POINT ( 'NONE',  ( 204.4254563108872844, 13.44278843410413771, -2.187257959407755248 ) ) ;
#17913=FACE_OUTER_BOUND ( 'NONE', #7720, .T. ) ;
#17916=CARTESIAN_POINT ( 'NONE',  ( 208.5220424616560422, 2.921106821514924512, -14.00000000000005507 ) ) ;
#17920=ADVANCED_FACE ( 'NONE', ( #10409, #4174 ), #13721, .F. ) ;
#17929=FACE_OUTER_BOUND ( 'NONE', #6634, .T. ) ;
#17930=CARTESIAN_POINT ( 'NONE',  ( 195.2585560139913810, 8.150276080056761074, -20.52105855319921446 ) ) ;
#17932=ORIENTED_EDGE ( 'NONE', *, *, #2209, .F. ) ;
#17934=FACE_OUTER_BOUND ( 'NONE', #1877, .T. ) ;
#17937=DIRECTION ( 'NONE',  ( 0.8426815769442684845, 0.4865224352899188420, 0.2306158707424263155 ) ) ;
#17940=EDGE_CURVE ( 'NONE', #16469, #1522, #14534, .T. ) ;
#17941=VERTEX_POINT ( 'NONE', #2486 ) ;
#17942=CARTESIAN_POINT ( 'NONE',  ( 208.0983737146324870, 5.661548828456886895, -14.00000000000005507 ) ) ;
#17950=ORIENTED_EDGE ( 'NONE', *, *, #18302, .T. ) ;
#17952=AXIS2_PLACEMENT_3D ( 'NONE', #13217, #4937, #17681 ) ;
#17955=CARTESIAN_POINT ( 'NONE',  ( 198.4028805101389992, 5.310605495132000975, -23.06309126349794170 ) ) ;
#17960=CARTESIAN_POINT ( 'NONE',  ( 208.5178070548358278, 11.68151032033851600, -25.34310559273333396 ) ) ;
#17961=EDGE_LOOP ( 'NONE', ( #10532, #14888, #11685, #19695 ) ) ;
#17964=DIRECTION ( 'NONE',  ( 0.8660254037844355990, 0.5000000000000054401, 0.000000000000000000 ) ) ;
#17965=CONICAL_SURFACE ( 'NONE', #19975, 13.07248899748297433, 0.6693469023067423196 ) ;
#17972=CARTESIAN_POINT ( 'NONE',  ( 209.6243204174557206, 3.018531609524862880, -14.00000000000005507 ) ) ;
#17976=VECTOR ( 'NONE', #11743, 999.9999999999998863 ) ;
#17979=AXIS2_PLACEMENT_3D ( 'NONE', #11520, #8112, #3357 ) ;
#17987=CARTESIAN_POINT ( 'NONE',  ( 207.7157532681331134, 10.68739508888871548, -1.717498466822861225 ) ) ;
#17991=CARTESIAN_POINT ( 'NONE',  ( 195.6523656023913702, 4.253644234526245071, -11.09368851308730974 ) ) ;
#17993=DIRECTION ( 'NONE',  ( 0.5000000000000055511, -0.8660254037844353769, 1.110223024625156417E-16 ) ) ;
#17994=ORIENTED_EDGE ( 'NONE', *, *, #13502, .F. ) ;
#17995=ORIENTED_EDGE ( 'NONE', *, *, #8998, .F. ) ;
#17998=CIRCLE ( 'NONE', #12252, 12.47473710546057823 ) ;
#18001=ORIENTED_EDGE ( 'NONE', *, *, #20424, .T. ) ;
#18008=CARTESIAN_POINT ( 'NONE',  ( 200.4364383576235866, 6.484680665789935183, -3.188775577416750995 ) ) ;
#18009=DIRECTION ( 'NONE',  ( -0.8528685319524407227, -0.4924038765061096168, -0.1736481776669271115 ) ) ;
#18014=LINE ( 'NONE', #13453, #14337 ) ;
#18022=CARTESIAN_POINT ( 'NONE',  ( 208.1960812450810465, 4.072754371081502178, -2.075899210536066963 ) ) ;
#18024=CIRCLE ( 'NONE', #4133, 12.47473710546057823 ) ;
#18026=ORIENTED_EDGE ( 'NONE', *, *, #10228, .T. ) ;
#18029=EDGE_LOOP ( 'NONE', ( #8172, #2399, #13647 ) ) ;
#18031=CARTESIAN_POINT ( 'NONE',  ( 204.1847125716027733, 2.529609678273321727, -2.551678190571418092 ) ) ;
#18037=VERTEX_POINT ( 'NONE', #17529 ) ;
#18038=CARTESIAN_POINT ( 'NONE',  ( 208.5367637565365158, 11.69245497716835480, -16.77975104236438497 ) ) ;
#18041=CARTESIAN_POINT ( 'NONE',  ( 205.8264633344831225, 9.596613037118636669, -14.00000000000005507 ) ) ;
#18042=VERTEX_POINT ( 'NONE', #14470 ) ;
#18053=EDGE_CURVE ( 'NONE', #17781, #18441, #9447, .T. ) ;
#18054=PLANE ( 'NONE',  #17824 ) ;
#18060=DIRECTION ( 'NONE',  ( 0.5000000000000052180, -0.8660254037844355990, 2.220446049250312341E-16 ) ) ;
#18063=DIRECTION ( 'NONE',  ( -0.8660254037844354880, -0.5000000000000055511, 0.000000000000000000 ) ) ;
#18067=AXIS2_PLACEMENT_3D ( 'NONE', #15831, #15633, #5844 ) ;
#18070=DIRECTION ( 'NONE',  ( -0.5566703992264088185, -0.3213938048432679051, 0.7660444431189864511 ) ) ;
#18072=ORIENTED_EDGE ( 'NONE', *, *, #536, .T. ) ;
#18074=LINE ( 'NONE', #2274, #10187 ) ;
#18075=CARTESIAN_POINT ( 'NONE',  ( 205.8311783259423464, 2.707377034109388347, -2.561001429077326197 ) ) ;
#18077=DIRECTION ( 'NONE',  ( -0.8640469734401363677, -0.5034111914617517280, 1.224637277265100606E-16 ) ) ;
#18080=ORIENTED_EDGE ( 'NONE', *, *, #17809, .F. ) ;
#18087=DIRECTION ( 'NONE',  ( 0.8660254037844369313, 0.5000000000000027756, 0.000000000000000000 ) ) ;
#18090=LINE ( 'NONE', #2085, #19332 ) ;
#18096=VERTEX_POINT ( 'NONE', #17744 ) ;
#18099=DIRECTION ( 'NONE',  ( 0.5000000000000054401, -0.8660254037844354880, 0.000000000000000000 ) ) ;
#18100=EDGE_CURVE ( 'NONE', #15951, #10374, #3207, .T. ) ;
#18106=ORIENTED_EDGE ( 'NONE', *, *, #6141, .F. ) ;
#18107=ORIENTED_EDGE ( 'NONE', *, *, #11302, .T. ) ;
#18112=ADVANCED_FACE ( 'NONE', ( #3524 ), #13390, .T. ) ;
#18119=ORIENTED_EDGE ( 'NONE', *, *, #15159, .F. ) ;
#18121=EDGE_LOOP ( 'NONE', ( #18150, #12447, #8109, #2467, #19062, #2855 ) ) ;
#18122=CARTESIAN_POINT ( 'NONE',  ( 198.3196067457501783, -0.8566107491083605474, -18.25196083293855409 ) ) ;
#18127=ORIENTED_EDGE ( 'NONE', *, *, #17043, .T. ) ;
#18128=AXIS2_PLACEMENT_3D ( 'NONE', #16754, #5602, #7205 ) ;
#18133=DIRECTION ( 'NONE',  ( 0.5000000000000049960, -0.8660254037844358210, 0.000000000000000000 ) ) ;
#18134=DIRECTION ( 'NONE',  ( 0.5000000000000054401, -0.8660254037844354880, 0.000000000000000000 ) ) ;
#18138=DIRECTION ( 'NONE',  ( -0.5000000000000054401, 0.8660254037844354880, -0.000000000000000000 ) ) ;
#18141=VECTOR ( 'NONE', #7834, 1000.000000000000114 ) ;
#18142=CARTESIAN_POINT ( 'NONE',  ( 205.5965122587965084, 9.994899983462953941, -14.00000000000005507 ) ) ;
#18144=B_SPLINE_CURVE_WITH_KNOTS ( 'NONE', 3,
 ( #17771, #16189, #20735, #8097 ),
 .UNSPECIFIED., .F., .F.,
 ( 4, 4 ),
 ( 3.628021920466675907E-05, 0.0007089310112617852253 ),
 .UNSPECIFIED. ) ;
#18145=EDGE_CURVE ( 'NONE', #13448, #6800, #18260, .T. ) ;
#18150=ORIENTED_EDGE ( 'NONE', *, *, #10953, .F. ) ;
#18151=VERTEX_POINT ( 'NONE', #8607 ) ;
#18155=ORIENTED_EDGE ( 'NONE', *, *, #6658, .F. ) ;
#18158=CIRCLE ( 'NONE', #18830, 12.47473710546057823 ) ;
#18162=VERTEX_POINT ( 'NONE', #8712 ) ;
#18164=PLANE ( 'NONE',  #6483 ) ;
#18168=EDGE_CURVE ( 'NONE', #17905, #10545, #17097, .T. ) ;
#18181=DIRECTION ( 'NONE',  ( -0.5171545105027488543, -0.2985792958513952544, 0.8021231927550450669 ) ) ;
#18182=EDGE_LOOP ( 'NONE', ( #5650, #286, #14756, #6218, #3684, #7865 ) ) ;
#18194=CARTESIAN_POINT ( 'NONE',  ( 205.6925730159677244, 2.884952444891475842, -25.61390257072243770 ) ) ;
#18198=CARTESIAN_POINT ( 'NONE',  ( 204.7012550509497260, 2.055015527128745578, -24.96223045542551233 ) ) ;
#18199=DIRECTION ( 'NONE',  ( 0.8660254037844355990, 0.5000000000000054401, 3.462567121588067547E-14 ) ) ;
#18200=ORIENTED_EDGE ( 'NONE', *, *, #10984, .F. ) ;
#18206=VECTOR ( 'NONE', #17389, 1000.000000000000114 ) ;
#18207=EDGE_CURVE ( 'NONE', #5044, #17666, #20469, .T. ) ;
#18210=CARTESIAN_POINT ( 'NONE',  ( 198.5343390728978932, -1.505455072869313238, -12.62839849932143643 ) ) ;
#18211=EDGE_CURVE ( 'NONE', #8949, #16469, #4785, .T. ) ;
#18217=VECTOR ( 'NONE', #5733, 1000.000000000000114 ) ;
#18218=CYLINDRICAL_SURFACE ( 'NONE', #14932, 12.47473710546057646 ) ;
#18221=ORIENTED_EDGE ( 'NONE', *, *, #4874, .T. ) ;
#18224=B_SPLINE_CURVE_WITH_KNOTS ( 'NONE', 3,
 ( #15154, #18624, #16826, #10119 ),
 .UNSPECIFIED., .F., .F.,
 ( 4, 4 ),
 ( 1.578338979930638950E-06, 0.0006742291310329615386 ),
 .UNSPECIFIED. ) ;
#18225=PLANE ( 'NONE',  #6097 ) ;
#18231=DIRECTION ( 'NONE',  ( 0.5000000000000051070, -0.8660254037844355990, -1.942890293094023946E-16 ) ) ;
#18233=AXIS2_PLACEMENT_3D ( 'NONE', #15903, #1274, #19656 ) ;
#18234=DIRECTION ( 'NONE',  ( -0.5000000000000049960, 0.8660254037844358210, -0.000000000000000000 ) ) ;
#18236=LINE ( 'NONE', #5283, #649 ) ;
#18239=CARTESIAN_POINT ( 'NONE',  ( 205.8264633344831225, 9.596613037118636669, -14.00000000000005507 ) ) ;
#18241=ORIENTED_EDGE ( 'NONE', *, *, #16223, .F. ) ;
#18242=CARTESIAN_POINT ( 'NONE',  ( 196.3264911765913041, 4.642850816258196289, -8.609703802792473937 ) ) ;
#18246=EDGE_LOOP ( 'NONE', ( #1181, #19812, #10503, #2907 ) ) ;
#18250=LINE ( 'NONE', #13877, #15298 ) ;
#18253=ORIENTED_EDGE ( 'NONE', *, *, #7420, .T. ) ;
#18254=ORIENTED_EDGE ( 'NONE', *, *, #8069, .T. ) ;
#18256=LINE ( 'NONE', #12008, #13420 ) ;
#18258=ORIENTED_EDGE ( 'NONE', *, *, #10300, .F. ) ;
#18260=LINE ( 'NONE', #16776, #10091 ) ;
#18263=ORIENTED_EDGE ( 'NONE', *, *, #6092, .F. ) ;
#18264=CARTESIAN_POINT ( 'NONE',  ( 203.8052576239561802, 8.960718637850693113, -2.195132782454258358 ) ) ;
#18270=DIRECTION ( 'NONE',  ( 0.8689290541588563510, 0.000000000000000000, -0.4949366614412345489 ) ) ;
#18278=DIRECTION ( 'NONE',  ( 0.8601696498176563122, 0.4966191788709776733, 0.1160929141252233648 ) ) ;
#18279=CARTESIAN_POINT ( 'NONE',  ( 212.3629815419766373, 18.02552076297307337, -20.52105855319947025 ) ) ;
#18282=EDGE_LOOP ( 'NONE', ( #1696, #16489, #3320, #13163 ) ) ;
#18283=EDGE_CURVE ( 'NONE', #10895, #3900, #15826, .T. ) ;
#18292=AXIS2_PLACEMENT_3D ( 'NONE', #10678, #14417, #1055 ) ;
#18293=CARTESIAN_POINT ( 'NONE',  ( 205.5965122587965084, 9.994899983462953941, -14.00000000000005507 ) ) ;
#18298=ORIENTED_EDGE ( 'NONE', *, *, #12394, .F. ) ;
#18299=CARTESIAN_POINT ( 'NONE',  ( 198.4225180578738161, 5.321943238602927728, -4.915515517929134326 ) ) ;
#18302=EDGE_CURVE ( 'NONE', #19734, #16889, #12537, .T. ) ;
#18307=CARTESIAN_POINT ( 'NONE',  ( 205.9193846489986583, 10.18131044486005443, -11.67614332468980365 ) ) ;
#18308=AXIS2_PLACEMENT_3D ( 'NONE', #17942, #8269, #233 ) ;
#18309=CARTESIAN_POINT ( 'NONE',  ( 206.3904739784021842, 10.45329399600353959, -16.68557076349156176 ) ) ;
#18311=B_SPLINE_CURVE_WITH_KNOTS ( 'NONE', 3,
 ( #3356, #19564, #11316, #16605 ),
 .UNSPECIFIED., .F., .F.,
 ( 4, 4 ),
 ( 8.130009260317344714E-07, 0.0008547987389088694586 ),
 .UNSPECIFIED. ) ;
#18317=EDGE_CURVE ( 'NONE', #3711, #15941, #6038, .T. ) ;
#18318=DIRECTION ( 'NONE',  ( -0.8660254037844357100, -0.5000000000000051070, 0.000000000000000000 ) ) ;
#18319=VECTOR ( 'NONE', #3766, 1000.000000000000114 ) ;
#18324=VERTEX_POINT ( 'NONE', #12741 ) ;
#18329=ORIENTED_EDGE ( 'NONE', *, *, #16940, .F. ) ;
#18332=VERTEX_POINT ( 'NONE', #19106 ) ;
#18344=LINE ( 'NONE', #6877, #5533 ) ;
#18345=ORIENTED_EDGE ( 'NONE', *, *, #13388, .F. ) ;
#18348=CARTESIAN_POINT ( 'NONE',  ( 214.9166615741016244, 8.725703323795450217, -24.01557619556987078 ) ) ;
#18349=DIRECTION ( 'NONE',  ( 1.000000000000000000, 2.509104035652853150E-14, 0.000000000000000000 ) ) ;
#18350=EDGE_CURVE ( 'NONE', #7973, #13380, #3506, .T. ) ;
#18352=VECTOR ( 'NONE', #16158, 1000.000000000000000 ) ;
#18358=AXIS2_PLACEMENT_3D ( 'NONE', #6282, #3325, #12776 ) ;
#18360=CIRCLE ( 'NONE', #10912, 12.47473710546057823 ) ;
#18361=DIRECTION ( 'NONE',  ( -0.5000000000000049960, 0.8660254037844357100, -0.000000000000000000 ) ) ;
#18363=EDGE_CURVE ( 'NONE', #11167, #8949, #12826, .T. ) ;
#18367=CARTESIAN_POINT ( 'NONE',  ( 209.3909370991932235, 3.422763374394450775, -14.00000000000005507 ) ) ;
#18374=LINE ( 'NONE', #13710, #346 ) ;
#18375=AXIS2_PLACEMENT_3D ( 'NONE', #13973, #20510, #12274 ) ;
#18378=DIRECTION ( 'NONE',  ( -0.6299240516454519545, -0.3636868207865264768, 0.6862416378687370422 ) ) ;
#18379=CYLINDRICAL_SURFACE ( 'NONE', #12464, 12.47473710546057646 ) ;
#18383=CARTESIAN_POINT ( 'NONE',  ( 197.6158938898029191, 5.210277915641273516, -6.188753603159779182 ) ) ;
#18384=CARTESIAN_POINT ( 'NONE',  ( 198.7027818574981666, 10.13880079795527323, -24.25943249057081630 ) ) ;
#18388=VERTEX_POINT ( 'NONE', #12646 ) ;
#18394=CARTESIAN_POINT ( 'NONE',  ( 197.9670180026625417, -1.060177954843255499, -16.89203719259486647 ) ) ;
#18395=VERTEX_POINT ( 'NONE', #4675 ) ;
#18397=CARTESIAN_POINT ( 'NONE',  ( 217.4723034443702545, 9.685982978710988789, -7.343163769975822319 ) ) ;
#18399=ORIENTED_EDGE ( 'NONE', *, *, #18559, .F. ) ;
#18406=ORIENTED_EDGE ( 'NONE', *, *, #16298, .F. ) ;
#18407=VERTEX_POINT ( 'NONE', #3192 ) ;
#18409=CARTESIAN_POINT ( 'NONE',  ( 213.4477085251712936, 18.65178817871777994, -9.972943347742015519 ) ) ;
#18411=VERTEX_POINT ( 'NONE', #11143 ) ;
#18414=CARTESIAN_POINT ( 'NONE',  ( 205.5965122587965084, 9.994899983462953941, -14.00000000000005507 ) ) ;
#18421=CARTESIAN_POINT ( 'NONE',  ( 203.9637611243273057, 8.521181414665040421, -26.28791492288515386 ) ) ;
#18423=LINE ( 'NONE', #3892, #20623 ) ;
#18424=ADVANCED_FACE ( 'NONE', ( #17929 ), #16139, .F. ) ;
#18425=CARTESIAN_POINT ( 'NONE',  ( 196.7772661521197222, -0.8746956702846723219, -14.00000000000005507 ) ) ;
#18427=CARTESIAN_POINT ( 'NONE',  ( 210.5759555690915192, 16.99378083647902216, -24.58554911381534325 ) ) ;
#18428=VECTOR ( 'NONE', #11616, 1000.000000000000114 ) ;
#18430=DIRECTION ( 'NONE',  ( 0.5000000000000054401, -0.8660254037844354880, 0.000000000000000000 ) ) ;
#18431=ORIENTED_EDGE ( 'NONE', *, *, #16901, .T. ) ;
#18435=ORIENTED_EDGE ( 'NONE', *, *, #11493, .F. ) ;
#18437=EDGE_CURVE ( 'NONE', #15696, #3474, #11258, .T. ) ;
#18439=DIRECTION ( 'NONE',  ( -0.5000000000000049960, 0.8660254037844357100, -0.000000000000000000 ) ) ;
#18441=VERTEX_POINT ( 'NONE', #20879 ) ;
#18442=PLANE ( 'NONE',  #10032 ) ;
#18446=CARTESIAN_POINT ( 'NONE',  ( 204.7255155853154918, 2.069022353175566931, -3.025685634606110952 ) ) ;
#18450=B_SPLINE_CURVE_WITH_KNOTS ( 'NONE', 3,
 ( #696, #15450, #806, #7152 ),
 .UNSPECIFIED., .F., .F.,
 ( 4, 4 ),
 ( 1.854400302406807709E-06, 0.0008558401382792385015 ),
 .UNSPECIFIED. ) ;
#18454=CARTESIAN_POINT ( 'NONE',  ( 216.2725394319739110, 15.91768827161142674, -14.00000000000005507 ) ) ;
#18462=CARTESIAN_POINT ( 'NONE',  ( 207.8527399996651184, 15.42153159440924881, -3.125199447383529172 ) ) ;
#18470=ORIENTED_EDGE ( 'NONE', *, *, #1844, .F. ) ;
#18471=DIRECTION ( 'NONE',  ( -0.8660254037844350439, -0.5000000000000061062, 0.000000000000000000 ) ) ;
#18475=DIRECTION ( 'NONE',  ( 0.5000000000000049960, -0.8660254037844358210, 0.000000000000000000 ) ) ;
#18482=ORIENTED_EDGE ( 'NONE', *, *, #6886, .F. ) ;
#18483=CARTESIAN_POINT ( 'NONE',  ( 199.2144802262915846, 21.04890371929339921, -14.00000000000005507 ) ) ;
#18484=DIRECTION ( 'NONE',  ( -0.2961981327260175823, -0.1710100716628329964, 0.9396926207859105373 ) ) ;
#18489=EDGE_CURVE ( 'NONE', #5298, #12547, #19601, .T. ) ;
#18490=ORIENTED_EDGE ( 'NONE', *, *, #5637, .F. ) ;
#18491=ORIENTED_EDGE ( 'NONE', *, *, #13316, .T. ) ;
#18494=DIRECTION ( 'NONE',  ( -0.5000000000000052180, 0.8660254037844355990, 0.000000000000000000 ) ) ;
#18502=VERTEX_POINT ( 'NONE', #6769 ) ;
#18510=DIRECTION ( 'NONE',  ( -0.8137976813493682515, -0.4698463103929579887, 0.3420201433256764290 ) ) ;
#18513=CARTESIAN_POINT ( 'NONE',  ( 199.3895759864363413, 6.411323655772897645, -23.60546391700144397 ) ) ;
#18514=ORIENTED_EDGE ( 'NONE', *, *, #4022, .F. ) ;
#18516=VERTEX_POINT ( 'NONE', #18031 ) ;
#18520=ORIENTED_EDGE ( 'NONE', *, *, #18437, .F. ) ;
#18544=VECTOR ( 'NONE', #2290, 1000.000000000000000 ) ;
#18547=CARTESIAN_POINT ( 'NONE',  ( 199.2144802262915846, 21.04890371929339921, -14.00000000000005507 ) ) ;
#18549=EDGE_CURVE ( 'NONE', #14915, #2174, #19684, .T. ) ;
#18550=ORIENTED_EDGE ( 'NONE', *, *, #15491, .F. ) ;
#18554=CARTESIAN_POINT ( 'NONE',  ( 208.8107687779841228, 4.427644383670616079, -14.00000000000005507 ) ) ;
#18558=VECTOR ( 'NONE', #6696, 1000.000000000000114 ) ;
#18559=EDGE_CURVE ( 'NONE', #16469, #9266, #18236, .T. ) ;
#18566=ORIENTED_EDGE ( 'NONE', *, *, #20937, .F. ) ;
#18568=MECHANICAL_DESIGN_GEOMETRIC_PRESENTATION_REPRESENTATION('',(#11120),#1978);
#18569=ORIENTED_EDGE ( 'NONE', *, *, #15881, .T. ) ;
#18570=LINE ( 'NONE', #18462, #19982 ) ;
#18577=CARTESIAN_POINT ( 'NONE',  ( 203.5058955171470814, 23.52655349267333307, -2.551678190571530891 ) ) ;
#18578=LINE ( 'NONE', #6047, #5575 ) ;
#18586=VERTEX_POINT ( 'NONE', #2762 ) ;
#18588=CARTESIAN_POINT ( 'NONE',  ( 197.5788830768223647, 5.011893035631070248, -6.091045511236785615 ) ) ;
#18590=CARTESIAN_POINT ( 'NONE',  ( 195.9724448824713932, 4.438442093042461956, -18.06789442459577089 ) ) ;
#18595=CARTESIAN_POINT ( 'NONE',  ( 218.9914638623158396, 11.07829152179047760, -11.13829696442610029 ) ) ;
#18600=DIRECTION ( 'NONE',  ( -0.5000000000000049960, 0.8660254037844357100, -0.000000000000000000 ) ) ;
#18601=FACE_OUTER_BOUND ( 'NONE', #15227, .T. ) ;
#18605=CARTESIAN_POINT ( 'NONE',  ( 217.4948448325154970, 10.21421812206089541, -7.132002368301439077 ) ) ;
#18606=ORIENTED_EDGE ( 'NONE', *, *, #12280, .T. ) ;
#18617=VERTEX_POINT ( 'NONE', #10798 ) ;
#18618=DIRECTION ( 'NONE',  ( 0.8660254037844355990, 0.5000000000000054401, 0.000000000000000000 ) ) ;
#18619=DIRECTION ( 'NONE',  ( -0.5000000000000049960, 0.8660254037844357100, -0.000000000000000000 ) ) ;
#18624=CARTESIAN_POINT ( 'NONE',  ( 195.1605391527415350, 3.615661520069893164, -12.56470246848373229 ) ) ;
#18625=DIRECTION ( 'NONE',  ( 0.8660254037844352659, 0.5000000000000056621, 0.000000000000000000 ) ) ;
#18628=LINE ( 'NONE', #14944, #14423 ) ;
#18636=DIRECTION ( 'NONE',  ( -0.8660254037844355990, -0.5000000000000055511, 0.000000000000000000 ) ) ;
#18641=VERTEX_POINT ( 'NONE', #18973 ) ;
#18647=ORIENTED_EDGE ( 'NONE', *, *, #10793, .F. ) ;
#18650=CARTESIAN_POINT ( 'NONE',  ( 217.4465006036304260, 9.413486477856961798, -20.57673792763531040 ) ) ;
#18651=AXIS2_PLACEMENT_3D ( 'NONE', #12500, #14213, #13996 ) ;
#18652=ORIENTED_EDGE ( 'NONE', *, *, #9017, .T. ) ;
#18657=CONICAL_SURFACE ( 'NONE', #16962, 10.85470691220533190, 0.8171114040043576665 ) ;
#18658=DIRECTION ( 'NONE',  ( -0.8645602258681711616, -0.4991540791356392504, 0.05814482891047982605 ) ) ;
#18659=CONICAL_SURFACE ( 'NONE', #10152, 13.07248899748297433, 0.6693469023067423196 ) ;
#18674=ORIENTED_EDGE ( 'NONE', *, *, #20819, .T. ) ;
#18679=AXIS2_PLACEMENT_3D ( 'NONE', #10955, #20588, #2901 ) ;
#18680=B_SPLINE_CURVE_WITH_KNOTS ( 'NONE', 3,
 ( #10158, #16755, #14981, #2025 ),
 .UNSPECIFIED., .F., .F.,
 ( 4, 4 ),
 ( 2.759414894271772668E-07, 0.0006729267335465118505 ),
 .UNSPECIFIED. ) ;
#18681=ADVANCED_FACE ( 'NONE', ( #10690 ), #15296, .T. ) ;
#18682=AXIS2_PLACEMENT_3D ( 'NONE', #12879, #15856, #11074 ) ;
#18683=PLANE ( 'NONE',  #6879 ) ;
#18687=DIRECTION ( 'NONE',  ( 0.8660254037844352659, 0.5000000000000056621, 0.000000000000000000 ) ) ;
#18689=DIRECTION ( 'NONE',  ( 0.8660254037844352659, 0.5000000000000056621, 0.000000000000000000 ) ) ;
#18694=PLANE ( 'NONE',  #16014 ) ;
#18696=VERTEX_POINT ( 'NONE', #15709 ) ;
#18699=CARTESIAN_POINT ( 'NONE',  ( 208.4761278624580711, 5.007259451653140125, -14.00000000000005507 ) ) ;
#18700=EDGE_CURVE ( 'NONE', #15334, #18407, #7203, .T. ) ;
#18702=ORIENTED_EDGE ( 'NONE', *, *, #16233, .T. ) ;
#18704=EDGE_CURVE ( 'NONE', #9959, #10895, #2553, .T. ) ;
#18708=CONICAL_SURFACE ( 'NONE', #8539, 13.07248899748297433, 0.6693469023067423196 ) ;
#18710=UNCERTAINTY_MEASURE_WITH_UNIT (LENGTH_MEASURE( 1.000000000000000082E-05 ), #20717, 'distance_accuracy_value', 'NONE');
#18712=DIRECTION ( 'NONE',  ( -0.5000000000000049960, 0.8660254037844358210, -0.000000000000000000 ) ) ;
#18715=EDGE_CURVE ( 'NONE', #5971, #5172, #12314, .T. ) ;
#18716=DIRECTION ( 'NONE',  ( 0.5000000000000054401, -0.8660254037844354880, 0.000000000000000000 ) ) ;
#18719=DIRECTION ( 'NONE',  ( -0.6946590618905412740, -0.4010615963775223669, 0.5971585917027958379 ) ) ;
#18721=VECTOR ( 'NONE', #2320, 1000.000000000000000 ) ;
#18727=ORIENTED_EDGE ( 'NONE', *, *, #16127, .T. ) ;
#18730=ORIENTED_EDGE ( 'NONE', *, *, #19229, .F. ) ;
#18734=CARTESIAN_POINT ( 'NONE',  ( 208.0983737146324870, 5.661548828456886895, -14.00000000000005507 ) ) ;
#18735=CARTESIAN_POINT ( 'NONE',  ( 205.8264633344831225, 9.596613037118636669, -14.00000000000005507 ) ) ;
#18742=CARTESIAN_POINT ( 'NONE',  ( 209.8909370991932235, 2.556737970610013733, -14.00000000000005507 ) ) ;
#18752=CARTESIAN_POINT ( 'NONE',  ( 208.5840039954387066, 11.71972914181512060, -2.522505859538486828 ) ) ;
#18755=ORIENTED_EDGE ( 'NONE', *, *, #7537, .T. ) ;
#18758=DIRECTION ( 'NONE',  ( -0.05035489893517486326, -0.02907241445524025303, -0.9983081582712680646 ) ) ;
#18760=FACE_OUTER_BOUND ( 'NONE', #3026, .T. ) ;
#18764=CARTESIAN_POINT ( 'NONE',  ( 215.3457899893760725, 15.62364810561754958, -18.11117897393244647 ) ) ;
#18773=CARTESIAN_POINT ( 'NONE',  ( 213.8661528393178060, 8.119191822981960627, -3.188775577416895324 ) ) ;
#18782=DIRECTION ( 'NONE',  ( -0.5000000000000054401, 0.8660254037844354880, -0.000000000000000000 ) ) ;
#18783=AXIS2_PLACEMENT_3D ( 'NONE', #10634, #2914, #19030 ) ;
#18784=DIRECTION ( 'NONE',  ( 0.8660254037844355990, 0.5000000000000054401, 0.000000000000000000 ) ) ;
#18786=CARTESIAN_POINT ( 'NONE',  ( 214.9079348888216998, 19.49485026284914113, -11.01983352639526892 ) ) ;
#18789=DIRECTION ( 'NONE',  ( 0.3430151393149032946, 0.1980398830195792548, -0.9182161068802751069 ) ) ;
#18791=CARTESIAN_POINT ( 'NONE',  ( 197.7356731787758690, -1.966565041833207017, -17.08769543353810860 ) ) ;
#18792=CARTESIAN_POINT ( 'NONE',  ( 202.6529885701316971, 8.118445885262769224, -2.363289276295887920 ) ) ;
#18793=CARTESIAN_POINT ( 'NONE',  ( 216.3403026830736735, 15.84380369567995039, -15.42323214253238284 ) ) ;
#18795=EDGE_CURVE ( 'NONE', #4228, #12427, #1684, .T. ) ;
#18796=VECTOR ( 'NONE', #19669, 1000.000000000000114 ) ;
#18800=CARTESIAN_POINT ( 'NONE',  ( 208.0983737146324870, 5.661548828456886895, -14.00000000000005507 ) ) ;
#18802=B_SPLINE_CURVE_WITH_KNOTS ( 'NONE', 3,
 ( #16849, #8787, #3802, #18650 ),
 .UNSPECIFIED., .F., .F.,
 ( 4, 4 ),
 ( 6.440264277512764414E-07, 0.0008546297644107766264 ),
 .UNSPECIFIED. ) ;
#18804=ORIENTED_EDGE ( 'NONE', *, *, #7965, .F. ) ;
#18819=EDGE_LOOP ( 'NONE', ( #10734, #4090, #12245 ) ) ;
#18820=ADVANCED_FACE ( 'NONE', ( #6534 ), #9516, .F. ) ;
#18827=VERTEX_POINT ( 'NONE', #13035 ) ;
#18829=EDGE_LOOP ( 'NONE', ( #20556, #16923, #6557, #9449, #9785, #10692 ) ) ;
#18830=AXIS2_PLACEMENT_3D ( 'NONE', #9183, #16941, #18949 ) ;
#18837=CARTESIAN_POINT ( 'NONE',  ( 202.8297164780629487, 0.8660905863451863196, -14.00000000000005507 ) ) ;
#18838=DIRECTION ( 'NONE',  ( -0.5000000000000054401, 0.8660254037844354880, -0.000000000000000000 ) ) ;
#18839=TOROIDAL_SURFACE ( 'NONE', #1244, 6.960520131757804485, 1.000000000000000000 ) ;
#18841=AXIS2_PLACEMENT_3D ( 'NONE', #18937, #20512, #20618 ) ;
#18844=EDGE_CURVE ( 'NONE', #9959, #112, #6431, .T. ) ;
#18852=EDGE_LOOP ( 'NONE', ( #6440, #13386, #12498, #17504 ) ) ;
#18854=CARTESIAN_POINT ( 'NONE',  ( 215.9829844511909300, 15.46048323788008361, -18.25196083293883120 ) ) ;
#18856=VERTEX_POINT ( 'NONE', #20856 ) ;
#18858=EDGE_CURVE ( 'NONE', #19734, #10275, #6329, .T. ) ;
#18859=EDGE_LOOP ( 'NONE', ( #10646, #15563, #17746, #10963 ) ) ;
#18861=DIRECTION ( 'NONE',  ( 0.8660254037844355990, 0.5000000000000054401, 0.000000000000000000 ) ) ;
#18862=CARTESIAN_POINT ( 'NONE',  ( 196.1782232529825762, 4.026199028858075124, -19.61257667712936126 ) ) ;
#18865=ORIENTED_EDGE ( 'NONE', *, *, #9775, .T. ) ;
#18868=ADVANCED_FACE ( 'NONE', ( #19284 ), #8022, .F. ) ;
#18869=LINE ( 'NONE', #12084, #13139 ) ;
#18872=EDGE_CURVE ( 'NONE', #1818, #17716, #17799, .T. ) ;
#18877=VERTEX_POINT ( 'NONE', #18210 ) ;
#18881=LINE ( 'NONE', #4353, #17309 ) ;
#18886=ADVANCED_FACE ( 'NONE', ( #10024 ), #14848, .T. ) ;
#18887=VERTEX_POINT ( 'NONE', #6743 ) ;
#18895=EDGE_LOOP ( 'NONE', ( #14315, #15819, #3489, #20622 ) ) ;
#18899=FACE_OUTER_BOUND ( 'NONE', #3986, .T. ) ;
#18902=EDGE_CURVE ( 'NONE', #6444, #16315, #6013, .T. ) ;
#18907=ORIENTED_EDGE ( 'NONE', *, *, #2554, .T. ) ;
#18910=DIRECTION ( 'NONE',  ( -0.5000000000000054401, 0.8660254037844354880, -0.000000000000000000 ) ) ;
#18917=DIRECTION ( 'NONE',  ( 0.5000000000000051070, -0.8660254037844359321, 0.000000000000000000 ) ) ;
#18920=CARTESIAN_POINT ( 'NONE',  ( 206.2654030616020293, 10.38108426852119770, -13.50586075465474423 ) ) ;
#18921=CARTESIAN_POINT ( 'NONE',  ( 201.5089327760127844, 7.457924964560246117, -2.844109184787520839 ) ) ;
#18924=CARTESIAN_POINT ( 'NONE',  ( 205.0662616026534693, 10.91332106064940888, -14.00000000000005507 ) ) ;
#18927=VECTOR ( 'NONE', #6881, 1000.000000000000114 ) ;
#18928=ORIENTED_EDGE ( 'NONE', *, *, #12744, .T. ) ;
#18930=VERTEX_POINT ( 'NONE', #3675 ) ;
#18935=LINE ( 'NONE', #15770, #2127 ) ;
#18937=CARTESIAN_POINT ( 'NONE',  ( 211.6737232845934500, 17.62757732253168541, -21.59012016402730083 ) ) ;
#18939=EDGE_CURVE ( 'NONE', #18162, #4848, #11534, .T. ) ;
#18943=CARTESIAN_POINT ( 'NONE',  ( 205.5965122587965084, 9.994899983462953941, -14.00000000000005507 ) ) ;
#18946=CIRCLE ( 'NONE', #5731, 11.94520687646042667 ) ;
#18949=DIRECTION ( 'NONE',  ( -0.8660254037844355990, -0.5000000000000054401, -1.599177586275613688E-14 ) ) ;
#18951=ORIENTED_EDGE ( 'NONE', *, *, #12744, .F. ) ;
#18956=ORIENTED_EDGE ( 'NONE', *, *, #5232, .F. ) ;
#18957=ORIENTED_EDGE ( 'NONE', *, *, #19792, .F. ) ;
#18959=CARTESIAN_POINT ( 'NONE',  ( 195.4216187824591202, 18.83910615367374675, -14.00000000000005507 ) ) ;
#18969=LINE ( 'NONE', #10905, #14486 ) ;
#18971=AXIS2_PLACEMENT_3D ( 'NONE', #8702, #972, #7108 ) ;
#18973=CARTESIAN_POINT ( 'NONE',  ( 195.0692117681097955, 18.22871929987706352, -14.00000000000005507 ) ) ;
#18974=CIRCLE ( 'NONE', #689, 11.98469917212512215 ) ;
#18976=LINE ( 'NONE', #10916, #7495 ) ;
#18977=LINE ( 'NONE', #1176, #18206 ) ;
#18980=DIRECTION ( 'NONE',  ( -0.8660254037844355990, -0.5000000000000054401, 3.379131769260644202E-14 ) ) ;
#18982=DIRECTION ( 'NONE',  ( 0.000000000000000000, -0.000000000000000000, -1.000000000000000000 ) ) ;
#18985=ORIENTED_EDGE ( 'NONE', *, *, #16467, .T. ) ;
#18988=AXIS2_PLACEMENT_3D ( 'NONE', #17090, #18782, #3935 ) ;
#18989=ORIENTED_EDGE ( 'NONE', *, *, #6610, .F. ) ;
#18993=VECTOR ( 'NONE', #1707, 1000.000000000000227 ) ;
#18996=CIRCLE ( 'NONE', #11883, 12.47473710546057823 ) ;
#18998=CARTESIAN_POINT ( 'NONE',  ( 218.4348361543091812, 9.984102274091050333, -18.06789442459602668 ) ) ;
#19001=DIRECTION ( 'NONE',  ( 0.5000000000000051070, -0.8660254037844359321, 0.000000000000000000 ) ) ;
#19005=FACE_OUTER_BOUND ( 'NONE', #7660, .T. ) ;
#19007=CIRCLE ( 'NONE', #6806, 11.94520687646042667 ) ;
#19008=CARTESIAN_POINT ( 'NONE',  ( 219.1969384858217325, 10.68170148414690779, -13.99502662667482866 ) ) ;
#19013=AXIS2_PLACEMENT_3D ( 'NONE', #17972, #14706, #16382 ) ;
#19018=DIRECTION ( 'NONE',  ( 0.5171545105027588463, 0.2985792958514009166, 0.8021231927550366292 ) ) ;
#19019=CARTESIAN_POINT ( 'NONE',  ( 203.2336538649942668, 12.75470097114692969, -25.81526893633797570 ) ) ;
#19022=ORIENTED_EDGE ( 'NONE', *, *, #9891, .F. ) ;
#19030=DIRECTION ( 'NONE',  ( 0.8660254037844352659, 0.5000000000000056621, 0.000000000000000000 ) ) ;
#19031=ADVANCED_FACE ( 'NONE', ( #5889 ), #9072, .T. ) ;
#19035=ORIENTED_EDGE ( 'NONE', *, *, #12792, .T. ) ;
#19038=DIRECTION ( 'NONE',  ( 0.5000000000000051070, -0.8660254037844359321, 0.000000000000000000 ) ) ;
#19040=ORIENTED_EDGE ( 'NONE', *, *, #17554, .T. ) ;
#19044=CIRCLE ( 'NONE', #4807, 11.98469917212512215 ) ;
#19047=ORIENTED_EDGE ( 'NONE', *, *, #17554, .F. ) ;
#19048=DIRECTION ( 'NONE',  ( -0.8601696498176565342, -0.4966191788709772847, -0.1160929141252230318 ) ) ;
#19052=CARTESIAN_POINT ( 'NONE',  ( 214.8600158830803650, 14.81213703278996618, -20.84195174293595443 ) ) ;
#19054=DIRECTION ( 'NONE',  ( 0.3886714912512186371, 0.2243995901002275029, -0.8936326403234182703 ) ) ;
#19058=FACE_OUTER_BOUND ( 'NONE', #15480, .T. ) ;
#19059=LINE ( 'NONE', #6208, #19294 ) ;
#19062=ORIENTED_EDGE ( 'NONE', *, *, #8567, .T. ) ;
#19066=DIRECTION ( 'NONE',  ( -0.7739085681710395903, -0.4468163201617135760, -0.4487991802004505648 ) ) ;
#19071=DIRECTION ( 'NONE',  ( -0.05035489893516267162, -0.02907241445523285617, 0.9983081582712687307 ) ) ;
#19073=DIRECTION ( 'NONE',  ( 0.5000000000000055511, -0.8660254037844354880, 0.000000000000000000 ) ) ;
#19076=ORIENTED_EDGE ( 'NONE', *, *, #12550, .T. ) ;
#19077=DIRECTION ( 'NONE',  ( -0.8660254037844354880, -0.5000000000000055511, 0.000000000000000000 ) ) ;
#19078=CARTESIAN_POINT ( 'NONE',  ( 192.7522908873522738, 17.31795696490239678, -4.003039906353937916 ) ) ;
#19079=EDGE_CURVE ( 'NONE', #15072, #17245, #6487, .T. ) ;
#19084=LINE ( 'NONE', #6232, #20896 ) ;
#19088=CARTESIAN_POINT ( 'NONE',  ( 205.5965122587965084, 9.994899983462953941, -14.00000000000005507 ) ) ;
#19089=LINE ( 'NONE', #8031, #18141 ) ;
#19092=ORIENTED_EDGE ( 'NONE', *, *, #13159, .F. ) ;
#19098=DIRECTION ( 'NONE',  ( -0.9795788631971381610, 0.000000000000000000, 0.2010603162670408506 ) ) ;
#19101=VECTOR ( 'NONE', #12833, 1000.000000000000114 ) ;
#19105=CARTESIAN_POINT ( 'NONE',  ( 213.9187556984697380, 7.376742007230097542, -24.25943249057096907 ) ) ;
#19106=CARTESIAN_POINT ( 'NONE',  ( 205.2612434495831621, 1.115232799514996209, -14.00000000000005507 ) ) ;
#19109=ADVANCED_FACE ( 'NONE', ( #7271 ), #1999, .T. ) ;
#19113=CARTESIAN_POINT ( 'NONE',  ( 215.9737506317248119, 15.45515208972567756, -9.718744748713270099 ) ) ;
#19117=DIRECTION ( 'NONE',  ( 0.2961981327260175267, 0.1710100716628331352, -0.9396926207859105373 ) ) ;
#19120=FACE_OUTER_BOUND ( 'NONE', #18829, .T. ) ;
#19125=EDGE_CURVE ( 'NONE', #6033, #8359, #11826, .T. ) ;
#19136=ADVANCED_FACE ( 'NONE', ( #4319 ), #13761, .F. ) ;
#19140=DIRECTION ( 'NONE',  ( 0.6946590618905486014, 0.4010615963775267523, 0.5971585917027842916 ) ) ;
#19141=EDGE_CURVE ( 'NONE', #1190, #6217, #18423, .T. ) ;
#19145=DIRECTION ( 'NONE',  ( 0.8426815769442658199, 0.4865224352899169546, -0.2306158707424407761 ) ) ;
#19153=DIRECTION ( 'NONE',  ( -0.7951984747223628247, -0.4591080534401421609, -0.3960797660391544572 ) ) ;
#19155=DIRECTION ( 'NONE',  ( -0.8660254037844357100, -0.5000000000000051070, 0.000000000000000000 ) ) ;
#19157=DIRECTION ( 'NONE',  ( -0.4758887346169382027, -0.2747544890354036706, 0.8354878114129395961 ) ) ;
#19159=EDGE_CURVE ( 'NONE', #2247, #14942, #7514, .T. ) ;
#19162=B_SPLINE_CURVE_WITH_KNOTS ( 'NONE', 3,
 ( #18605, #15136, #18397, #16907 ),
 .UNSPECIFIED., .F., .F.,
 ( 4, 4 ),
 ( 5.392423665750742885E-07, 0.0008545249803497876294 ),
 .UNSPECIFIED. ) ;
#19164=ORIENTED_EDGE ( 'NONE', *, *, #11184, .F. ) ;
#19166=CARTESIAN_POINT ( 'NONE',  ( 213.2304086110926278, 13.87128283563446018, -4.915515517929359035 ) ) ;
#19169=ORIENTED_EDGE ( 'NONE', *, *, #15491, .T. ) ;
#19171=CARTESIAN_POINT ( 'NONE',  ( 206.6134256523022259, 3.931827829199530999, -26.28791492288515386 ) ) ;
#19176=VERTEX_POINT ( 'NONE', #9591 ) ;
#19177=ORIENTED_EDGE ( 'NONE', *, *, #10551, .F. ) ;
#19178=VECTOR ( 'NONE', #11086, 1000.000000000000227 ) ;
#19183=LINE ( 'NONE', #2969, #16996 ) ;
#19186=EDGE_LOOP ( 'NONE', ( #11109, #12557, #10537, #3797, #8895, #6791 ) ) ;
#19193=ORIENTED_EDGE ( 'NONE', *, *, #7216, .T. ) ;
#19195=ORIENTED_EDGE ( 'NONE', *, *, #4975, .T. ) ;
#19197=PLANE ( 'NONE',  #17161 ) ;
#19199=CARTESIAN_POINT ( 'NONE',  ( 209.7177441667290339, 12.37429433490069997, -24.99940654434242759 ) ) ;
#19202=B_SPLINE_CURVE_WITH_KNOTS ( 'NONE', 3,
 ( #10636, #20289, #5755, #1122 ),
 .UNSPECIFIED., .F., .F.,
 ( 4, 4 ),
 ( 0.0004399335472996286221, 0.0008623086312854339732 ),
 .UNSPECIFIED. ) ;
#19203=DIRECTION ( 'NONE',  ( 0.8660254037844355990, 0.5000000000000054401, 0.000000000000000000 ) ) ;
#19204=ADVANCED_FACE ( 'NONE', ( #17675 ), #12797, .F. ) ;
#19212=CARTESIAN_POINT ( 'NONE',  ( 208.0154570403101104, 11.39147840422468150, -16.96430480073851399 ) ) ;
#19213=CARTESIAN_POINT ( 'NONE',  ( 209.3909370991932519, 3.422763374394458769, -14.00000000000005507 ) ) ;
#19214=LINE ( 'NONE', #4586, #13598 ) ;
#19215=DIRECTION ( 'NONE',  ( 0.5000000000000049960, -0.8660254037844358210, 0.000000000000000000 ) ) ;
#19219=EDGE_CURVE ( 'NONE', #6001, #3962, #16087, .T. ) ;
#19224=VERTEX_POINT ( 'NONE', #1248 ) ;
#19228=ORIENTED_EDGE ( 'NONE', *, *, #16161, .F. ) ;
#19229=EDGE_CURVE ( 'NONE', #6453, #9959, #14611, .T. ) ;
#19230=FACE_OUTER_BOUND ( 'NONE', #7813, .T. ) ;
#19232=LINE ( 'NONE', #9769, #11433 ) ;
#19233=EDGE_CURVE ( 'NONE', #15281, #6173, #3992, .T. ) ;
#19235=CARTESIAN_POINT ( 'NONE',  ( 208.0983737146324870, 5.661548828456886895, -14.00000000000005507 ) ) ;
#19236=AXIS2_PLACEMENT_3D ( 'NONE', #15431, #12126, #13937 ) ;
#19238=EDGE_CURVE ( 'NONE', #1853, #6314, #18144, .T. ) ;
#19241=CARTESIAN_POINT ( 'NONE',  ( 205.8894739819445761, 2.741034046794848855, -25.34310559273324159 ) ) ;
#19244=VERTEX_POINT ( 'NONE', #1347 ) ;
#19246=EDGE_CURVE ( 'NONE', #11760, #2644, #6204, .T. ) ;
#19250=CARTESIAN_POINT ( 'NONE',  ( 201.4958824572256333, 7.627400263678961068, -2.990331769139143780 ) ) ;
#19252=EDGE_CURVE ( 'NONE', #6453, #1337, #13526, .T. ) ;
#19254=DIRECTION ( 'NONE',  ( -0.8660254037844358210, -0.5000000000000049960, 0.000000000000000000 ) ) ;
#19257=EDGE_CURVE ( 'NONE', #20124, #16739, #7084, .T. ) ;
#19258=ADVANCED_FACE ( 'NONE', ( #6096 ), #9276, .F. ) ;
#19264=CARTESIAN_POINT ( 'NONE',  ( 199.4425753138606296, -0.2082645440182918917, -20.84195174293567376 ) ) ;
#19266=ORIENTED_EDGE ( 'NONE', *, *, #16940, .T. ) ;
#19274=ORIENTED_EDGE ( 'NONE', *, *, #20007, .T. ) ;
#19276=LINE ( 'NONE', #7777, #15629 ) ;
#19278=DIRECTION ( 'NONE',  ( -0.5000000000000054401, 0.8660254037844354880, -0.000000000000000000 ) ) ;
#19279=VERTEX_POINT ( 'NONE', #2939 ) ;
#19284=FACE_OUTER_BOUND ( 'NONE', #12351, .T. ) ;
#19285=DIRECTION ( 'NONE',  ( 0.8660254037844355990, 0.5000000000000054401, 8.899770914925154148E-15 ) ) ;
#19294=VECTOR ( 'NONE', #9283, 1000.000000000000227 ) ;
#19296=ORIENTED_EDGE ( 'NONE', *, *, #9251, .T. ) ;
#19301=CARTESIAN_POINT ( 'NONE',  ( 210.0930887352476759, 12.05995036078138583, -25.46066938576263894 ) ) ;
#19302=ORIENTED_EDGE ( 'NONE', *, *, #15653, .T. ) ;
#19310=DIRECTION ( 'NONE',  ( 0.8528685319524387243, 0.4924038765061080070, -0.1736481776669413502 ) ) ;
#19319=CIRCLE ( 'NONE', #6106, 12.47473710546057823 ) ;
#19323=AXIS2_PLACEMENT_3D ( 'NONE', #10780, #9287, #17474 ) ;
#19331=CARTESIAN_POINT ( 'NONE',  ( 198.4821375217713353, 5.887413813925527428, -22.72623880687287468 ) ) ;
#19332=VECTOR ( 'NONE', #3178, 999.9999999999998863 ) ;
#19340=ORIENTED_EDGE ( 'NONE', *, *, #13714, .T. ) ;
#19341=CARTESIAN_POINT ( 'NONE',  ( 193.6508758837858011, 7.222081524111755968, -19.95367855226118081 ) ) ;
#19342=ADVANCED_FACE ( 'NONE', ( #384 ), #8784, .T. ) ;
#19345=ORIENTED_EDGE ( 'NONE', *, *, #4362, .F. ) ;
#19349=DIRECTION ( 'NONE',  ( -0.5000000000000049960, 0.8660254037844358210, -0.000000000000000000 ) ) ;
#19350=CONICAL_SURFACE ( 'NONE', #6465, 10.85470691220533190, 0.8171114040043576665 ) ;
#19365=DIRECTION ( 'NONE',  ( -0.8660254037844355990, -0.5000000000000051070, 0.000000000000000000 ) ) ;
#19366=ORIENTED_EDGE ( 'NONE', *, *, #15245, .F. ) ;
#19367=ORIENTED_EDGE ( 'NONE', *, *, #1008, .T. ) ;
#19368=ORIENTED_EDGE ( 'NONE', *, *, #2394, .F. ) ;
#19369=CARTESIAN_POINT ( 'NONE',  ( 196.7640869814540565, 9.019494789394645551, -5.407152407593843968 ) ) ;
#19372=EDGE_LOOP ( 'NONE', ( #6015, #17725, #7733, #14930, #2619, #13151 ) ) ;
#19373=ORIENTED_EDGE ( 'NONE', *, *, #3990, .F. ) ;
#19374=ORIENTED_EDGE ( 'NONE', *, *, #1350, .F. ) ;
#19376=CARTESIAN_POINT ( 'NONE',  ( 214.6548693368118848, 14.87071829951450930, -7.229707551136565158 ) ) ;
#19377=DIRECTION ( 'NONE',  ( -0.5000000000000049960, 0.8660254037844357100, -0.000000000000000000 ) ) ;
#19382=DIRECTION ( 'NONE',  ( 0.7743856023693594937, 0.000000000000000000, -0.6327139470906613106 ) ) ;
#19393=ADVANCED_FACE ( 'NONE', ( #19005 ), #11699, .T. ) ;
#19400=CARTESIAN_POINT ( 'NONE',  ( 208.0983737146324870, 5.661548828456886895, -14.00000000000005507 ) ) ;
#19403=CARTESIAN_POINT ( 'NONE',  ( 209.9679726729889921, 12.16473724899237041, -25.30691987834803669 ) ) ;
#19404=ORIENTED_EDGE ( 'NONE', *, *, #10268, .T. ) ;
#19406=CIRCLE ( 'NONE', #3502, 1.000000000000000888 ) ;
#19411=FACE_OUTER_BOUND ( 'NONE', #16103, .T. ) ;
#19413=DIRECTION ( 'NONE',  ( 0.5016613886297202063, 0.000000000000000000, -0.8650640734408641119 ) ) ;
#19415=ORIENTED_EDGE ( 'NONE', *, *, #12418, .T. ) ;
#19425=VERTEX_POINT ( 'NONE', #2286 ) ;
#19428=DIRECTION ( 'NONE',  ( -0.8660254037844354880, -0.5000000000000055511, 0.000000000000000000 ) ) ;
#19430=CARTESIAN_POINT ( 'NONE',  ( 209.9266392777186923, 12.49489998346296638, -2.187257959407756136 ) ) ;
#19435=ORIENTED_EDGE ( 'NONE', *, *, #1060, .T. ) ;
#19436=LINE ( 'NONE', #4916, #8845 ) ;
#19439=DIRECTION ( 'NONE',  ( 0.6048098792058536066, 0.000000000000000000, 0.7963698952214358640 ) ) ;
#19445=EDGE_CURVE ( 'NONE', #20929, #7471, #802, .T. ) ;
#19446=ORIENTED_EDGE ( 'NONE', *, *, #19845, .T. ) ;
#19448=ADVANCED_FACE ( 'NONE', ( #590 ), #16808, .F. ) ;
#19453=DIRECTION ( 'NONE',  ( 0.1503837331804444843, 0.08682408883347161876, 0.9848077530122060219 ) ) ;
#19458=VERTEX_POINT ( 'NONE', #12143 ) ;
#19468=ORIENTED_EDGE ( 'NONE', *, *, #13951, .T. ) ;
#19471=EDGE_CURVE ( 'NONE', #9396, #19458, #19162, .T. ) ;
#19473=ADVANCED_FACE ( 'NONE', ( #1302 ), #14778, .T. ) ;
#19474=AXIS2_PLACEMENT_3D ( 'NONE', #4583, #5757, #2996 ) ;
#19476=LINE ( 'NONE', #4959, #1099 ) ;
#19480=ORIENTED_EDGE ( 'NONE', *, *, #8290, .T. ) ;
#19481=DIRECTION ( 'NONE',  ( -0.6048098792058536066, 0.000000000000000000, -0.7963698952214358640 ) ) ;
#19483=EDGE_CURVE ( 'NONE', #5859, #1000, #4080, .T. ) ;
#19488=CARTESIAN_POINT ( 'NONE',  ( 218.8737197432240293, 10.23749183229395676, -11.23040475586419085 ) ) ;
#19492=B_SPLINE_CURVE_WITH_KNOTS ( 'NONE', 3,
 ( #19811, #9843, #10259, #5281 ),
 .UNSPECIFIED., .F., .F.,
 ( 4, 4 ),
 ( 3.993865398787763773E-07, 0.0006730501785855516356 ),
 .UNSPECIFIED. ) ;
#19496=ADVANCED_FACE ( 'NONE', ( #17623 ), #11355, .T. ) ;
#19498=VERTEX_POINT ( 'NONE', #3299 ) ;
#19501=CARTESIAN_POINT ( 'NONE',  ( 211.8034485311565049, 13.57847631115287435, -23.60546391700164648 ) ) ;
#19502=AXIS2_PLACEMENT_3D ( 'NONE', #18837, #17560, #4311 ) ;
#19506=FACE_OUTER_BOUND ( 'NONE', #19372, .T. ) ;
#19508=FACE_OUTER_BOUND ( 'NONE', #6813, .T. ) ;
#19509=ADVANCED_FACE ( 'NONE', ( #23 ), #17731, .F. ) ;
#19511=ORIENTED_EDGE ( 'NONE', *, *, #19711, .F. ) ;
#19520=VECTOR ( 'NONE', #4183, 1000.000000000000227 ) ;
#19521=CIRCLE ( 'NONE', #1264, 12.47473710546057823 ) ;
#19523=VERTEX_POINT ( 'NONE', #7954 ) ;
#19524=DIRECTION ( 'NONE',  ( -0.5000000000000054401, 0.8660254037844354880, -0.000000000000000000 ) ) ;
#19527=ADVANCED_FACE ( 'NONE', ( #9546 ), #6277, .T. ) ;
#19537=VECTOR ( 'NONE', #17547, 1000.000000000000114 ) ;
#19539=EDGE_LOOP ( 'NONE', ( #15045, #17846, #19340, #5511, #12952, #8210, #1565, #16476, #20723, #8701, #19988, #10767, #5244, #5571, #17169, #5769, #12272, #14, #7214, #703, #11528, #4386, #11428, #16538, #18263, #20897, #1777, #4822, #3604, #8546, #12028, #10328, #6324, #1112, #257, #14111, #11836, #706, #4234, #4308, #6166, #7806, #10789, #16166, #3469, #18907, #20509, #7642, #18470, #8520, #5982, #5476, #20633, #13354, #20467, #10072, #6992, #13353, #11176, #8730, #11593, #6413, #16251, #7365, #19366, #13522, #19883, #1261, #18647, #20536, #19969, #8604, #9286, #13795, #7251, #7264, #18435, #1836, #17351, #4041, #10174, #20325, #17207, #3447, #306, #20386, #17038, #16943, #7038, #185, #5352, #15177, #11925, #18431, #1162, #9854, #9572, #8248, #20188, #2277, #9935, #5483, #11905, #15582, #11062, #10199, #16104, #3622 ) ) ;
#19548=VECTOR ( 'NONE', #963, 1000.000000000000114 ) ;
#19551=CIRCLE ( 'NONE', #17544, 11.94520687646042667 ) ;
#19557=CARTESIAN_POINT ( 'NONE',  ( 205.8264633344831225, 9.596613037118636669, -14.00000000000005507 ) ) ;
#19559=DIRECTION ( 'NONE',  ( -0.5000000000000051070, 0.8660254037844359321, -0.000000000000000000 ) ) ;
#19561=ORIENTED_EDGE ( 'NONE', *, *, #7606, .F. ) ;
#19564=CARTESIAN_POINT ( 'NONE',  ( 218.5943730328090737, 10.59141717271569938, -9.788772202513543519 ) ) ;
#19567=ORIENTED_EDGE ( 'NONE', *, *, #15019, .F. ) ;
#19576=VERTEX_POINT ( 'NONE', #14770 ) ;
#19583=CARTESIAN_POINT ( 'NONE',  ( 205.0662616026534693, 10.91332106064940888, -14.00000000000005507 ) ) ;
#19588=EDGE_CURVE ( 'NONE', #18617, #11306, #1709, .T. ) ;
#19590=VECTOR ( 'NONE', #18009, 1000.000000000000114 ) ;
#19592=VERTEX_POINT ( 'NONE', #16234 ) ;
#19595=ORIENTED_EDGE ( 'NONE', *, *, #315, .T. ) ;
#19597=CARTESIAN_POINT ( 'NONE',  ( 218.1243679439584469, 10.57767345991361552, -19.61257667712965258 ) ) ;
#19601=LINE ( 'NONE', #16543, #18927 ) ;
#19607=ORIENTED_EDGE ( 'NONE', *, *, #799, .F. ) ;
#19609=VECTOR ( 'NONE', #3351, 1000.000000000000227 ) ;
#19611=CARTESIAN_POINT ( 'NONE',  ( 198.6336827526812669, -1.448098972604089374, -15.39542905462715261 ) ) ;
#19612=B_SPLINE_CURVE_WITH_KNOTS ( 'NONE', 3,
 ( #13358, #1911, #14757, #11446 ),
 .UNSPECIFIED., .F., .F.,
 ( 4, 4 ),
 ( 1.737996164779797019E-05, 0.0008713656996325849693 ),
 .UNSPECIFIED. ) ;
#19615=AXIS2_PLACEMENT_3D ( 'NONE', #3514, #16244, #16355 ) ;
#19618=DIRECTION ( 'NONE',  ( -0.8660254037844357100, -0.5000000000000051070, 0.000000000000000000 ) ) ;
#19621=ORIENTED_EDGE ( 'NONE', *, *, #3282, .T. ) ;
#19624=AXIS2_PLACEMENT_3D ( 'NONE', #19341, #3021, #9680 ) ;
#19627=FACE_OUTER_BOUND ( 'NONE', #16290, .T. ) ;
#19628=EDGE_CURVE ( 'NONE', #8182, #15072, #6261, .T. ) ;
#19630=CARTESIAN_POINT ( 'NONE',  ( 219.0593366061551137, 10.34465777807333531, -13.97827067520052147 ) ) ;
#19632=EDGE_CURVE ( 'NONE', #4064, #12664, #19810, .T. ) ;
#19634=DIRECTION ( 'NONE',  ( -0.5000000000000054401, 0.8660254037844354880, -0.000000000000000000 ) ) ;
#19638=FACE_OUTER_BOUND ( 'NONE', #20308, .T. ) ;
#19643=ADVANCED_FACE ( 'NONE', ( #5392 ), #16861, .F. ) ;
#19648=CARTESIAN_POINT ( 'NONE',  ( 219.2080768649571496, 11.20335309717537520, -15.43274561385901400 ) ) ;
#19649=AXIS2_PLACEMENT_3D ( 'NONE', #17123, #5975, #7354 ) ;
#19650=EDGE_CURVE ( 'NONE', #11656, #15055, #11312, .T. ) ;
#19651=VECTOR ( 'NONE', #610, 1000.000000000000227 ) ;
#19654=AXIS2_PLACEMENT_3D ( 'NONE', #15832, #20789, #6257 ) ;
#19655=AXIS2_PLACEMENT_3D ( 'NONE', #4640, #17158, #14311 ) ;
#19656=DIRECTION ( 'NONE',  ( 1.000000000000000000, 0.000000000000000000, 0.000000000000000000 ) ) ;
#19658=ORIENTED_EDGE ( 'NONE', *, *, #7456, .T. ) ;
#19666=FACE_OUTER_BOUND ( 'NONE', #13029, .T. ) ;
#19667=LINE ( 'NONE', #17991, #11507 ) ;
#19669=DIRECTION ( 'NONE',  ( 0.8528685319524408337, 0.4924038765061092282, 0.1736481776669271115 ) ) ;
#19673=CARTESIAN_POINT ( 'NONE',  ( 188.4856654865874077, 14.85461964123948242, -12.53629070788332278 ) ) ;
#19675=FACE_OUTER_BOUND ( 'NONE', #18029, .T. ) ;
#19678=CARTESIAN_POINT ( 'NONE',  ( 215.8800731390675764, 9.281929250168950318, -4.915515517929356371 ) ) ;
#19683=CARTESIAN_POINT ( 'NONE',  ( 199.3895759864363413, 6.411323655772897645, -23.60546391700144397 ) ) ;
#19684=B_SPLINE_CURVE_WITH_KNOTS ( 'NONE', 3,
 ( #438, #14977, #6662, #15187 ),
 .UNSPECIFIED., .F., .F.,
 ( 4, 4 ),
 ( 0.0001188559543176825488, 0.0007915067463633553230 ),
 .UNSPECIFIED. ) ;
#19685=CONICAL_SURFACE ( 'NONE', #10547, 13.07248899748297433, 0.6693469023067423196 ) ;
#19686=CARTESIAN_POINT ( 'NONE',  ( 216.5552780741873278, 15.79089711517258188, -12.53629070788368338 ) ) ;
#19687=VECTOR ( 'NONE', #10505, 1000.000000000000114 ) ;
#19690=DIRECTION ( 'NONE',  ( 0.5000000000000052180, -0.8660254037844355990, -0.000000000000000000 ) ) ;
#19693=DIRECTION ( 'NONE',  ( -0.8660254037844355990, -0.5000000000000055511, 0.000000000000000000 ) ) ;
#19695=ORIENTED_EDGE ( 'NONE', *, *, #20908, .F. ) ;
#19701=AXIS2_PLACEMENT_3D ( 'NONE', #9438, #11148, #16144 ) ;
#19703=CONICAL_SURFACE ( 'NONE', #10206, 13.07248899748297433, 0.6693469023067423196 ) ;
#19704=ORIENTED_EDGE ( 'NONE', *, *, #1306, .F. ) ;
#19711=EDGE_CURVE ( 'NONE', #16315, #18586, #8975, .T. ) ;
#19713=LINE ( 'NONE', #11671, #9318 ) ;
#19714=DIRECTION ( 'NONE',  ( 0.7739085681710339282, 0.4468163201617103009, -0.4487991802004634434 ) ) ;
#19715=ORIENTED_EDGE ( 'NONE', *, *, #6308, .T. ) ;
#19716=B_SPLINE_CURVE_WITH_KNOTS ( 'NONE', 3,
 ( #248, #4808, #1532, #9673 ),
 .UNSPECIFIED., .F., .F.,
 ( 4, 4 ),
 ( 0.0001323875665768755629, 0.0008050383586195956074 ),
 .UNSPECIFIED. ) ;
#19717=CARTESIAN_POINT ( 'NONE',  ( 218.1243679439584469, 10.57767345991361552, -19.61257667712965258 ) ) ;
#19718=DIRECTION ( 'NONE',  ( -0.5000000000000049960, 0.8660254037844357100, -0.000000000000000000 ) ) ;
#19721=CARTESIAN_POINT ( 'NONE',  ( 214.9156946368443926, 7.952324971666334008, -4.494676796018850951 ) ) ;
#19723=DIRECTION ( 'NONE',  ( -0.8137976813493685846, -0.4698463103929575446, 0.3420201433256764290 ) ) ;
#19730=ORIENTED_EDGE ( 'NONE', *, *, #10551, .T. ) ;
#19734=VERTEX_POINT ( 'NONE', #8692 ) ;
#19744=CARTESIAN_POINT ( 'NONE',  ( 205.0662616026534693, 10.91332106064940888, -14.00000000000005507 ) ) ;
#19747=AXIS2_PLACEMENT_3D ( 'NONE', #6137, #15405, #13797 ) ;
#19758=DIRECTION ( 'NONE',  ( 0.5000000000000054401, -0.8660254037844354880, 0.000000000000000000 ) ) ;
#19759=EDGE_CURVE ( 'NONE', #19523, #19879, #19713, .T. ) ;
#19763=DIRECTION ( 'NONE',  ( -0.5000000000000051070, 0.8660254037844359321, -0.000000000000000000 ) ) ;
#19773=LINE ( 'NONE', #5239, #8145 ) ;
#19783=ORIENTED_EDGE ( 'NONE', *, *, #2917, .T. ) ;
#19787=ORIENTED_EDGE ( 'NONE', *, *, #295, .T. ) ;
#19790=CARTESIAN_POINT ( 'NONE',  ( 199.3883551940873247, 6.233608926798073213, -23.74217242726227894 ) ) ;
#19792=EDGE_CURVE ( 'NONE', #13943, #12995, #5820, .T. ) ;
#19794=LINE ( 'NONE', #16834, #415 ) ;
#19797=CARTESIAN_POINT ( 'NONE',  ( 205.1246204644237423, 9.368426547597012544, -26.29020529591235444 ) ) ;
#19799=EDGE_LOOP ( 'NONE', ( #9358, #12465, #7876, #531 ) ) ;
#19808=ORIENTED_EDGE ( 'NONE', *, *, #14406, .F. ) ;
#19810=CIRCLE ( 'NONE', #15442, 11.94520687646042667 ) ;
#19811=CARTESIAN_POINT ( 'NONE',  ( 214.0936945175409676, 14.36970118611001368, -22.03054070023868860 ) ) ;
#19812=ORIENTED_EDGE ( 'NONE', *, *, #4682, .T. ) ;
#19816=CARTESIAN_POINT ( 'NONE',  ( 203.0246517772554853, 23.22871929987706707, -14.00000000000005507 ) ) ;
#19819=CARTESIAN_POINT ( 'NONE',  ( 205.8534188064671469, 2.720217581527302642, -2.669358488461094581 ) ) ;
#19820=FACE_OUTER_BOUND ( 'NONE', #1832, .T. ) ;
#19821=LINE ( 'NONE', #860, #16644 ) ;
#19822=VECTOR ( 'NONE', #13465, 1000.000000000000114 ) ;
#19828=CARTESIAN_POINT ( 'NONE',  ( 205.9211985038822093, 10.18235767446534012, -26.70731555100845611 ) ) ;
#19830=ORIENTED_EDGE ( 'NONE', *, *, #1917, .T. ) ;
#19832=ADVANCED_FACE ( 'NONE', ( #10595 ), #4246, .F. ) ;
#19836=ORIENTED_EDGE ( 'NONE', *, *, #2933, .T. ) ;
#19840=DIRECTION ( 'NONE',  ( -0.5000000000000049960, 0.8660254037844357100, -0.000000000000000000 ) ) ;
#19845=EDGE_CURVE ( 'NONE', #14490, #3353, #2913, .T. ) ;
#19848=ORIENTED_EDGE ( 'NONE', *, *, #5993, .F. ) ;
#19850=DIRECTION ( 'NONE',  ( 0.05035489893516277571, 0.02907241445523329332, -0.9983081582712688418 ) ) ;
#19851=AXIS2_PLACEMENT_3D ( 'NONE', #17875, #14601, #12894 ) ;
#19852=CARTESIAN_POINT ( 'NONE',  ( 209.9266392777186923, 12.49489998346296105, -14.00000000000005507 ) ) ;
#19854=EDGE_CURVE ( 'NONE', #6173, #4965, #16969, .T. ) ;
#19856=ADVANCED_FACE ( 'NONE', ( #6133 ), #20349, .F. ) ;
#19858=DIRECTION ( 'NONE',  ( -0.5000000000000049960, 0.8660254037844358210, -0.000000000000000000 ) ) ;
#19860=CARTESIAN_POINT ( 'NONE',  ( 206.3750000662386697, 10.09033354729407428, -26.29020529591238287 ) ) ;
#19863=ORIENTED_EDGE ( 'NONE', *, *, #5399, .F. ) ;
#19870=CARTESIAN_POINT ( 'NONE',  ( 215.8300749258796145, 8.480242677682491959, -22.62267072728681327 ) ) ;
#19874=LINE ( 'NONE', #6720, #18319 ) ;
#19876=DIRECTION ( 'NONE',  ( 0.1005394128318207181, 0.05804645706261944010, 0.9932383577419421350 ) ) ;
#19877=ORIENTED_EDGE ( 'NONE', *, *, #11454, .T. ) ;
#19878=ORIENTED_EDGE ( 'NONE', *, *, #17670, .F. ) ;
#19879=VERTEX_POINT ( 'NONE', #10801 ) ;
#19881=CARTESIAN_POINT ( 'NONE',  ( 203.6497874834091704, 1.447950443965099421, -24.35247136794729528 ) ) ;
#19883=ORIENTED_EDGE ( 'NONE', *, *, #20931, .T. ) ;
#19889=FACE_OUTER_BOUND ( 'NONE', #9130, .T. ) ;
#19895=EDGE_CURVE ( 'NONE', #1475, #2644, #9305, .T. ) ;
#19898=B_SPLINE_CURVE_WITH_KNOTS ( 'NONE', 3,
 ( #202, #2114, #16423, #8564 ),
 .UNSPECIFIED., .F., .F.,
 ( 4, 4 ),
 ( 3.377843907047678752E-07, 0.0006729885764489780845 ),
 .UNSPECIFIED. ) ;
#19899=DIRECTION ( 'NONE',  ( 0.5000000000000054401, -0.8660254037844354880, 0.000000000000000000 ) ) ;
#19902=EDGE_CURVE ( 'NONE', #12634, #1760, #18977, .T. ) ;
#19905=LINE ( 'NONE', #6968, #16275 ) ;
#19912=FACE_OUTER_BOUND ( 'NONE', #15448, .T. ) ;
#19913=LINE ( 'NONE', #2223, #15455 ) ;
#19919=EDGE_LOOP ( 'NONE', ( #16819, #2488, #11646, #6723 ) ) ;
#19924=DIRECTION ( 'NONE',  ( 0.8660254037844355990, 0.5000000000000054401, -2.489154677768128945E-14 ) ) ;
#19929=DIRECTION ( 'NONE',  ( -0.5000000000000054401, 0.8660254037844354880, -0.000000000000000000 ) ) ;
#19935=CARTESIAN_POINT ( 'NONE',  ( 196.8447511938509535, 4.588041795376833321, -7.229707551136296040 ) ) ;
#19936=ORIENTED_EDGE ( 'NONE', *, *, #18207, .T. ) ;
#19942=ORIENTED_EDGE ( 'NONE', *, *, #1872, .F. ) ;
#19945=CARTESIAN_POINT ( 'NONE',  ( 211.7058770681882152, 6.356735158160116583, -25.61390257072256560 ) ) ;
#19946=LINE ( 'NONE', #12013, #16249 ) ;
#19947=ORIENTED_EDGE ( 'NONE', *, *, #5489, .F. ) ;
#19948=LINE ( 'NONE', #15110, #7176 ) ;
#19954=DIRECTION ( 'NONE',  ( -0.5000000000000049960, 0.8660254037844357100, -0.000000000000000000 ) ) ;
#19956=LINE ( 'NONE', #18384, #751 ) ;
#19959=VERTEX_POINT ( 'NONE', #3371 ) ;
#19961=ORIENTED_EDGE ( 'NONE', *, *, #19759, .F. ) ;
#19962=DIRECTION ( 'NONE',  ( 0.5000000000000051070, -0.8660254037844359321, 0.000000000000000000 ) ) ;
#19969=ORIENTED_EDGE ( 'NONE', *, *, #2145, .T. ) ;
#19972=VECTOR ( 'NONE', #3307, 1000.000000000000114 ) ;
#19975=AXIS2_PLACEMENT_3D ( 'NONE', #4056, #16788, #2267 ) ;
#19976=ORIENTED_EDGE ( 'NONE', *, *, #14119, .F. ) ;
#19980=PLANE ( 'NONE',  #18067 ) ;
#19982=VECTOR ( 'NONE', #866, 1000.000000000000114 ) ;
#19988=ORIENTED_EDGE ( 'NONE', *, *, #19588, .T. ) ;
#19989=CARTESIAN_POINT ( 'NONE',  ( 199.2144802262915846, 21.04890371929339921, -14.00000000000005507 ) ) ;
#19990=B_SPLINE_CURVE_WITH_KNOTS ( 'NONE', 3,
 ( #8281, #12874, #6377, #9870 ),
 .UNSPECIFIED., .F., .F.,
 ( 4, 4 ),
 ( 5.481513501809308120E-07, 0.0006731989434038709343 ),
 .UNSPECIFIED. ) ;
#19991=DIRECTION ( 'NONE',  ( -0.3430151393149036276, -0.1980398830195791438, 0.9182161068802751069 ) ) ;
#19992=VECTOR ( 'NONE', #8479, 1000.000000000000114 ) ;
#19994=ORIENTED_EDGE ( 'NONE', *, *, #343, .T. ) ;
#19995=ORIENTED_EDGE ( 'NONE', *, *, #14220, .T. ) ;
#19996=ORIENTED_EDGE ( 'NONE', *, *, #9891, .T. ) ;
#20001=AXIS2_PLACEMENT_3D ( 'NONE', #14883, #5687, #6783 ) ;
#20007=EDGE_CURVE ( 'NONE', #12264, #11172, #19084, .T. ) ;
#20017=VECTOR ( 'NONE', #18070, 999.9999999999998863 ) ;
#20018=DIRECTION ( 'NONE',  ( -0.8660254037844357100, -0.5000000000000049960, 0.000000000000000000 ) ) ;
#20019=VERTEX_POINT ( 'NONE', #1378 ) ;
#20023=ORIENTED_EDGE ( 'NONE', *, *, #7606, .T. ) ;
#20025=VERTEX_POINT ( 'NONE', #17229 ) ;
#20027=CARTESIAN_POINT ( 'NONE',  ( 203.5544658059540666, 23.53182819120163671, -14.00000000000005507 ) ) ;
#20030=FACE_OUTER_BOUND ( 'NONE', #8275, .T. ) ;
#20034=AXIS2_PLACEMENT_3D ( 'NONE', #18800, #18910, #4173 ) ;
#20040=EDGE_CURVE ( 'NONE', #4395, #14638, #5658, .T. ) ;
#20045=ORIENTED_EDGE ( 'NONE', *, *, #8707, .F. ) ;
#20047=AXIS2_PLACEMENT_3D ( 'NONE', #9356, #904, #4507 ) ;
#20048=DIRECTION ( 'NONE',  ( -0.6946590618905411629, -0.4010615963775225890, 0.5971585917027958379 ) ) ;
#20049=ADVANCED_FACE ( 'NONE', ( #20092 ), #14062, .T. ) ;
#20052=FACE_OUTER_BOUND ( 'NONE', #5164, .T. ) ;
#20053=CARTESIAN_POINT ( 'NONE',  ( 205.5965122587965084, 9.994899983462953941, -14.00000000000005507 ) ) ;
#20054=EDGE_LOOP ( 'NONE', ( #852, #19404, #14677, #12218 ) ) ;
#20062=CONICAL_SURFACE ( 'NONE', #2126, 10.85470691220533190, 0.8171114040043576665 ) ;
#20064=CARTESIAN_POINT ( 'NONE',  ( 213.2500461588270468, 13.88262057910513825, -23.06309126349817618 ) ) ;
#20072=LINE ( 'NONE', #8518, #14629 ) ;
#20082=EDGE_CURVE ( 'NONE', #2368, #425, #15351, .T. ) ;
#20085=DIRECTION ( 'NONE',  ( -0.9367698044638429478, 0.000000000000000000, -0.3499461864984006465 ) ) ;
#20086=ORIENTED_EDGE ( 'NONE', *, *, #15850, .T. ) ;
#20092=FACE_OUTER_BOUND ( 'NONE', #14399, .T. ) ;
#20094=DIRECTION ( 'NONE',  ( -0.5000000000000054401, 0.8660254037844354880, -0.000000000000000000 ) ) ;
#20095=EDGE_CURVE ( 'NONE', #20283, #5044, #20294, .T. ) ;
#20106=DIRECTION ( 'NONE',  ( -0.5016613886297335290, 0.000000000000000000, -0.8650640734408565624 ) ) ;
#20108=VECTOR ( 'NONE', #17499, 1000.000000000000227 ) ;
#20111=EDGE_CURVE ( 'NONE', #2861, #2041, #18450, .T. ) ;
#20113=EDGE_LOOP ( 'NONE', ( #2732, #10703, #8274, #10147 ) ) ;
#20114=DIRECTION ( 'NONE',  ( -0.8660254037844373753, -0.5000000000000022204, 0.000000000000000000 ) ) ;
#20124=VERTEX_POINT ( 'NONE', #13639 ) ;
#20125=ORIENTED_EDGE ( 'NONE', *, *, #20256, .F. ) ;
#20127=DIRECTION ( 'NONE',  ( -0.8944271909999204073, 0.000000000000000000, -0.4472135954999487684 ) ) ;
#20129=VERTEX_POINT ( 'NONE', #7355 ) ;
#20135=DIRECTION ( 'NONE',  ( -0.8660254037844355990, -0.5000000000000055511, 0.000000000000000000 ) ) ;
#20139=VERTEX_POINT ( 'NONE', #12147 ) ;
#20141=CARTESIAN_POINT ( 'NONE',  ( 214.9714796170919442, 8.242131668836057301, -23.72013913782489425 ) ) ;
#20144=CYLINDRICAL_SURFACE ( 'NONE', #3175, 12.47473710546057646 ) ;
#20155=ORIENTED_EDGE ( 'NONE', *, *, #12815, .F. ) ;
#20163=CIRCLE ( 'NONE', #6960, 12.47473710546057823 ) ;
#20164=DIRECTION ( 'NONE',  ( -0.8660254037844355990, -0.5000000000000053291, 0.000000000000000000 ) ) ;
#20165=AXIS2_PLACEMENT_3D ( 'NONE', #3976, #20686, #17021 ) ;
#20170=EDGE_CURVE ( 'NONE', #11314, #11315, #7693, .T. ) ;
#20173=DIRECTION ( 'NONE',  ( 0.000000000000000000, -0.000000000000000000, -1.000000000000000000 ) ) ;
#20176=VERTEX_POINT ( 'NONE', #4399 ) ;
#20177=ORIENTED_EDGE ( 'NONE', *, *, #1517, .F. ) ;
#20178=DIRECTION ( 'NONE',  ( 0.5000000000000053291, -0.8660254037844355990, -2.220446049250312588E-16 ) ) ;
#20184=CARTESIAN_POINT ( 'NONE',  ( 196.4465031000483179, 4.712139732572081741, -8.669480444820576892 ) ) ;
#20188=ORIENTED_EDGE ( 'NONE', *, *, #39, .T. ) ;
#20192=ORIENTED_EDGE ( 'NONE', *, *, #1246, .F. ) ;
#20193=VECTOR ( 'NONE', #4621, 1000.000000000000000 ) ;
#20196=DIRECTION ( 'NONE',  ( 0.8660254037844355990, 0.5000000000000054401, 3.615531934188343626E-15 ) ) ;
#20199=EDGE_LOOP ( 'NONE', ( #16532, #1805, #5373, #7364 ) ) ;
#20202=ORIENTED_EDGE ( 'NONE', *, *, #11032, .T. ) ;
#20204=CARTESIAN_POINT ( 'NONE',  ( 196.1661066256804986, 4.019203490823548997, -8.415281845791808379 ) ) ;
#20207=ORIENTED_EDGE ( 'NONE', *, *, #10809, .T. ) ;
#20208=AXIS2_PLACEMENT_3D ( 'NONE', #3859, #18278, #15024 ) ;
#20209=CARTESIAN_POINT ( 'NONE',  ( 208.9378540577313004, 11.39297530874010000, -25.94618751764496878 ) ) ;
#20215=DIRECTION ( 'NONE',  ( 0.8660254037844355990, 0.5000000000000054401, -1.334965637238773043E-14 ) ) ;
#20216=LINE ( 'NONE', #5684, #1560 ) ;
#20221=CARTESIAN_POINT ( 'NONE',  ( 198.8331280799749550, -1.075349935395403689, -9.858802615641089062 ) ) ;
#20224=ORIENTED_EDGE ( 'NONE', *, *, #16761, .F. ) ;
#20226=ORIENTED_EDGE ( 'NONE', *, *, #12890, .F. ) ;
#20234=EDGE_CURVE ( 'NONE', #9307, #6007, #7778, .T. ) ;
#20238=CARTESIAN_POINT ( 'NONE',  ( 199.2144802262915846, 21.04890371929339921, -14.00000000000005507 ) ) ;
#20244=ORIENTED_EDGE ( 'NONE', *, *, #17701, .F. ) ;
#20247=LINE ( 'NONE', #15304, #20710 ) ;
#20253=CARTESIAN_POINT ( 'NONE',  ( 199.2144802262915846, 21.04890371929339921, -14.00000000000005507 ) ) ;
#20254=LINE ( 'NONE', #3936, #4255 ) ;
#20256=EDGE_CURVE ( 'NONE', #3900, #1433, #1226, .T. ) ;
#20258=CARTESIAN_POINT ( 'NONE',  ( 206.4249228987308413, 10.47318308942859133, -14.95831141195905190 ) ) ;
#20259=ORIENTED_EDGE ( 'NONE', *, *, #171, .F. ) ;
#20264=EDGE_CURVE ( 'NONE', #14662, #5690, #52, .T. ) ;
#20267=ADVANCED_FACE ( 'NONE', ( #6490 ), #7007, .T. ) ;
#20268=LINE ( 'NONE', #3952, #6841 ) ;
#20278=ORIENTED_EDGE ( 'NONE', *, *, #6158, .T. ) ;
#20283=VERTEX_POINT ( 'NONE', #19241 ) ;
#20285=CARTESIAN_POINT ( 'NONE',  ( 197.5001239273001659, -2.102559465580161380, -12.41782726985249319 ) ) ;
#20286=DIRECTION ( 'NONE',  ( 0.5000000000000054401, -0.8660254037844354880, 0.000000000000000000 ) ) ;
#20288=ORIENTED_EDGE ( 'NONE', *, *, #8441, .T. ) ;
#20289=CARTESIAN_POINT ( 'NONE',  ( 198.2043721129365395, -1.441146303136960682, -13.99491531967994007 ) ) ;
#20293=PLANE ( 'NONE',  #19649 ) ;
#20294=LINE ( 'NONE', #15243, #8029 ) ;
#20295=AXIS2_PLACEMENT_3D ( 'NONE', #11180, #19038, #4513 ) ;
#20307=ORIENTED_EDGE ( 'NONE', *, *, #13828, .F. ) ;
#20308=EDGE_LOOP ( 'NONE', ( #13745, #5926, #1722, #8041, #11465, #18241 ) ) ;
#20313=DIRECTION ( 'NONE',  ( -0.8660254037844350439, -0.5000000000000061062, 0.000000000000000000 ) ) ;
#20318=AXIS2_PLACEMENT_3D ( 'NONE', #10710, #2248, #4036 ) ;
#20319=CARTESIAN_POINT ( 'NONE',  ( 213.9169459704606879, 7.890903399153988751, -24.64792178047109417 ) ) ;
#20325=ORIENTED_EDGE ( 'NONE', *, *, #8874, .T. ) ;
#20329=DIRECTION ( 'NONE',  ( 0.5000000000000049960, -0.8660254037844358210, 0.000000000000000000 ) ) ;
#20332=ORIENTED_EDGE ( 'NONE', *, *, #118, .F. ) ;
#20333=CARTESIAN_POINT ( 'NONE',  ( 218.5975169673276355, 10.59323232415630756, -18.20125362229464372 ) ) ;
#20335=CARTESIAN_POINT ( 'NONE',  ( 213.9946316566572193, 7.420549012114688203, -3.662783021451589960 ) ) ;
#20336=VECTOR ( 'NONE', #16310, 1000.000000000000114 ) ;
#20337=ORIENTED_EDGE ( 'NONE', *, *, #7090, .T. ) ;
#20341=TOROIDAL_SURFACE ( 'NONE', #2760, 4.730184897849351700, 1.000000000000000000 ) ;
#20342=CARTESIAN_POINT ( 'NONE',  ( 199.8561199650368110, 21.41935459518070317, -26.45271578590685380 ) ) ;
#20344=VECTOR ( 'NONE', #12752, 1000.000000000000114 ) ;
#20349=PLANE ( 'NONE',  #879 ) ;
#20351=CARTESIAN_POINT ( 'NONE',  ( 200.4130575059754733, 6.471181724797008705, -24.79563718815128226 ) ) ;
#20352=CARTESIAN_POINT ( 'NONE',  ( 202.6438527999323185, 0.8671737836725290638, -4.409371045252821197 ) ) ;
#20357=CIRCLE ( 'NONE', #9515, 1.000000000000000888 ) ;
#20361=DIRECTION ( 'NONE',  ( 0.5000000000000054401, -0.8660254037844354880, 2.220446049250312834E-16 ) ) ;
#20367=ORIENTED_EDGE ( 'NONE', *, *, #652, .T. ) ;
#20372=FACE_OUTER_BOUND ( 'NONE', #4767, .T. ) ;
#20374=DIRECTION ( 'NONE',  ( 0.5000000000000049960, -0.8660254037844358210, 0.000000000000000000 ) ) ;
#20376=CARTESIAN_POINT ( 'NONE',  ( 216.1221914169060199, 15.89489377461772079, -15.41371838795031657 ) ) ;
#20378=CARTESIAN_POINT ( 'NONE',  ( 199.2144802262915846, 21.04890371929339921, -14.00000000000005507 ) ) ;
#20382=DIRECTION ( 'NONE',  ( 0.5000000000000052180, -0.8660254037844355990, -1.665334536937734071E-16 ) ) ;
#20386=ORIENTED_EDGE ( 'NONE', *, *, #4208, .T. ) ;
#20387=DIRECTION ( 'NONE',  ( -0.5000000000000049960, 0.8660254037844358210, -0.000000000000000000 ) ) ;
#20390=FACE_OUTER_BOUND ( 'NONE', #2517, .T. ) ;
#20393=AXIS2_PLACEMENT_3D ( 'NONE', #8318, #11202, #11624 ) ;
#20394=B_SPLINE_CURVE_WITH_KNOTS ( 'NONE', 3,
 ( #10828, #20376, #18793, #17311 ),
 .UNSPECIFIED., .F., .F.,
 ( 4, 4 ),
 ( 0.0001343368750301437032, 0.0008069876670732752024 ),
 .UNSPECIFIED. ) ;
#20397=DIRECTION ( 'NONE',  ( 0.5000000000000051070, -0.8660254037844359321, 0.000000000000000000 ) ) ;
#20401=CARTESIAN_POINT ( 'NONE',  ( 208.7495889232815216, 11.81532964447892375, -15.82564276083900445 ) ) ;
#20407=ORIENTED_EDGE ( 'NONE', *, *, #15528, .T. ) ;
#20411=VERTEX_POINT ( 'NONE', #6591 ) ;
#20415=LINE ( 'NONE', #10987, #19178 ) ;
#20423=ADVANCED_FACE ( 'NONE', ( #17864 ), #7022, .T. ) ;
#20424=EDGE_CURVE ( 'NONE', #18395, #2861, #13398, .T. ) ;
#20428=CARTESIAN_POINT ( 'NONE',  ( 197.8194874830827814, 5.504832635710179112, -22.07143452975716258 ) ) ;
#20429=CARTESIAN_POINT ( 'NONE',  ( 208.8748369350943506, 26.62631326558856060, -8.415281845792092597 ) ) ;
#20430=ORIENTED_EDGE ( 'NONE', *, *, #15371, .F. ) ;
#20432=AXIS2_PLACEMENT_3D ( 'NONE', #1701, #20778, #16 ) ;
#20435=CYLINDRICAL_SURFACE ( 'NONE', #3736, 12.47473710546057646 ) ;
#20438=ORIENTED_EDGE ( 'NONE', *, *, #9644, .T. ) ;
#20444=VERTEX_POINT ( 'NONE', #17960 ) ;
#20446=ORIENTED_EDGE ( 'NONE', *, *, #629, .T. ) ;
#20447=EDGE_CURVE ( 'NONE', #20827, #17781, #251, .T. ) ;
#20449=CARTESIAN_POINT ( 'NONE',  ( 218.5362608324210782, 10.04265983930142347, -9.928836400542515150 ) ) ;
#20451=CARTESIAN_POINT ( 'NONE',  ( 212.2886526734226607, 13.32755979150977943, -4.003039906354141308 ) ) ;
#20452=CARTESIAN_POINT ( 'NONE',  ( 194.8843532073694291, 18.54890371929339565, -14.00000000000005507 ) ) ;
#20464=AXIS2_PLACEMENT_3D ( 'NONE', #7770, #17333, #14166 ) ;
#20466=DIRECTION ( 'NONE',  ( 0.8660254037844353769, 0.5000000000000054401, -3.055037149610300800E-16 ) ) ;
#20467=ORIENTED_EDGE ( 'NONE', *, *, #6403, .T. ) ;
#20468=CARTESIAN_POINT ( 'NONE',  ( 207.4176018615384010, 11.04630655582441356, -12.09449022909012328 ) ) ;
#20469=LINE ( 'NONE', #10821, #13503 ) ;
#20475=LINE ( 'NONE', #1101, #10872 ) ;
#20477=PLANE ( 'NONE',  #5331 ) ;
#20479=CARTESIAN_POINT ( 'NONE',  ( 209.4907977912994568, 12.24326678395481949, -15.16670265247205585 ) ) ;
#20485=ORIENTED_EDGE ( 'NONE', *, *, #1844, .T. ) ;
#20489=FACE_OUTER_BOUND ( 'NONE', #11487, .T. ) ;
#20491=ORIENTED_EDGE ( 'NONE', *, *, #15264, .F. ) ;
#20492=CARTESIAN_POINT ( 'NONE',  ( 195.8395605881523522, 4.361721309946301695, -9.913166705713630122 ) ) ;
#20493=EDGE_CURVE ( 'NONE', #13116, #4077, #9051, .T. ) ;
#20495=ORIENTED_EDGE ( 'NONE', *, *, #14425, .T. ) ;
#20496=CARTESIAN_POINT ( 'NONE',  ( 210.4326046345175314, 5.879217990898649049, -26.11230899909619652 ) ) ;
#20497=LINE ( 'NONE', #19212, #32 ) ;
#20500=DIRECTION ( 'NONE',  ( -0.8660254037844357100, -0.5000000000000051070, 0.000000000000000000 ) ) ;
#20501=EDGE_CURVE ( 'NONE', #2200, #14662, #13506, .T. ) ;
#20507=VECTOR ( 'NONE', #20631, 1000.000000000000227 ) ;
#20509=ORIENTED_EDGE ( 'NONE', *, *, #7784, .T. ) ;
#20510=DIRECTION ( 'NONE',  ( 0.5000000000000049960, -0.8660254037844357100, 0.000000000000000000 ) ) ;
#20511=DIRECTION ( 'NONE',  ( 0.5000000000000053291, -0.8660254037844355990, -3.330669073875468142E-16 ) ) ;
#20512=DIRECTION ( 'NONE',  ( -0.6299240516454518435, -0.3636868207865263103, 0.6862416378687374863 ) ) ;
#20517=VECTOR ( 'NONE', #18712, 1000.000000000000227 ) ;
#20518=EDGE_LOOP ( 'NONE', ( #1931, #19561, #17995, #11784, #792, #13494 ) ) ;
#20519=AXIS2_PLACEMENT_3D ( 'NONE', #13028, #5567, #11846 ) ;
#20520=DIRECTION ( 'NONE',  ( -0.8528685319524407227, -0.4924038765061097833, -0.1736481776669268062 ) ) ;
#20521=EDGE_CURVE ( 'NONE', #14504, #9868, #12123, .T. ) ;
#20522=B_SPLINE_CURVE_WITH_KNOTS ( 'NONE', 3,
 ( #5784, #1241, #14189, #6199 ),
 .UNSPECIFIED., .F., .F.,
 ( 4, 4 ),
 ( 3.066983677343236917E-07, 0.0006729574904181037653 ),
 .UNSPECIFIED. ) ;
#20530=EDGE_LOOP ( 'NONE', ( #4237, #20561 ) ) ;
#20531=ORIENTED_EDGE ( 'NONE', *, *, #11677, .F. ) ;
#20533=CARTESIAN_POINT ( 'NONE',  ( 212.8949410924155927, 14.03163993103081886, -5.166194743381471888 ) ) ;
#20536=ORIENTED_EDGE ( 'NONE', *, *, #5131, .T. ) ;
#20542=ORIENTED_EDGE ( 'NONE', *, *, #18704, .F. ) ;
#20543=ADVANCED_FACE ( 'NONE', ( #10726 ), #18379, .T. ) ;
#20547=VERTEX_POINT ( 'NONE', #3845 ) ;
#20552=AXIS2_PLACEMENT_3D ( 'NONE', #17382, #12507, #19077 ) ;
#20556=ORIENTED_EDGE ( 'NONE', *, *, #17326, .F. ) ;
#20561=ORIENTED_EDGE ( 'NONE', *, *, #13692, .T. ) ;
#20571=CIRCLE ( 'NONE', #11438, 11.94520687646042667 ) ;
#20572=DIRECTION ( 'NONE',  ( -0.5000000000000049960, 0.8660254037844358210, -0.000000000000000000 ) ) ;
#20573=EDGE_LOOP ( 'NONE', ( #17396, #19302, #17352 ) ) ;
#20578=DIRECTION ( 'NONE',  ( 0.5000000000000057732, -0.8660254037844352659, -1.942890293094023699E-16 ) ) ;
#20579=DIRECTION ( 'NONE',  ( -0.8660254037844369313, -0.5000000000000027756, 0.000000000000000000 ) ) ;
#20582=VECTOR ( 'NONE', #15585, 1000.000000000000114 ) ;
#20583=CARTESIAN_POINT ( 'NONE',  ( 204.6278860547989780, 24.17433503161487351, -24.79563718815146345 ) ) ;
#20587=CARTESIAN_POINT ( 'NONE',  ( 199.3993387870319509, 20.72871929987707063, -14.00000000000005507 ) ) ;
#20588=DIRECTION ( 'NONE',  ( -0.5000000000000049960, 0.8660254037844357100, -0.000000000000000000 ) ) ;
#20593=CARTESIAN_POINT ( 'NONE',  ( 213.8895336909654361, 8.132690763974602888, -24.79563718815146345 ) ) ;
#20597=VECTOR ( 'NONE', #1313, 1000.000000000000114 ) ;
#20601=ORIENTED_EDGE ( 'NONE', *, *, #20680, .T. ) ;
#20604=FACE_OUTER_BOUND ( 'NONE', #18246, .T. ) ;
#20608=DIRECTION ( 'NONE',  ( -0.7235536692358655042, -0.4177439057064740169, -0.5495089780708011240 ) ) ;
#20611=AXIS2_PLACEMENT_3D ( 'NONE', #20947, #12932, #11332 ) ;
#20616=DIRECTION ( 'NONE',  ( 0.5000000000000052180, -0.8660254037844355990, -0.000000000000000000 ) ) ;
#20618=DIRECTION ( 'NONE',  ( 0.7366891686653871396, 0.000000000000000000, 0.6762315200958181061 ) ) ;
#20619=DIRECTION ( 'NONE',  ( 1.000000000000000000, 0.000000000000000000, 0.000000000000000000 ) ) ;
#20620=CARTESIAN_POINT ( 'NONE',  ( 207.0125913935839606, 3.389466186736467268, -25.65046807331631129 ) ) ;
#20622=ORIENTED_EDGE ( 'NONE', *, *, #20170, .T. ) ;
#20623=VECTOR ( 'NONE', #7799, 1000.000000000000227 ) ;
#20624=EDGE_CURVE ( 'NONE', #16239, #2143, #9304, .T. ) ;
#20625=CARTESIAN_POINT ( 'NONE',  ( 197.5592321514251353, 4.823524888127141530, -22.03054070023847544 ) ) ;
#20631=DIRECTION ( 'NONE',  ( -0.5000000000000049960, 0.8660254037844358210, -0.000000000000000000 ) ) ;
#20633=ORIENTED_EDGE ( 'NONE', *, *, #2865, .F. ) ;
#20635=FACE_OUTER_BOUND ( 'NONE', #11135, .T. ) ;
#20637=ORIENTED_EDGE ( 'NONE', *, *, #7828, .F. ) ;
#20642=TOROIDAL_SURFACE ( 'NONE', #9797, 4.730184897849351700, 1.000000000000000000 ) ;
#20645=EDGE_CURVE ( 'NONE', #20444, #13693, #4377, .T. ) ;
#20650=CARTESIAN_POINT ( 'NONE',  ( 200.1915427753721417, 0.2241520214996718663, -5.993340328401664863 ) ) ;
#20661=PLANE ( 'NONE',  #19747 ) ;
#20667=EDGE_LOOP ( 'NONE', ( #20226, #1209, #20155, #19607, #4915, #15493 ) ) ;
#20668=EDGE_LOOP ( 'NONE', ( #12508, #119, #19076 ) ) ;
#20674=AXIS2_PLACEMENT_3D ( 'NONE', #11636, #18099, #17899 ) ;
#20680=EDGE_CURVE ( 'NONE', #5956, #3195, #3000, .T. ) ;
#20681=CARTESIAN_POINT ( 'NONE',  ( 215.9737506317248119, 15.45515208972567756, -9.718744748713270099 ) ) ;
#20685=ORIENTED_EDGE ( 'NONE', *, *, #11253, .T. ) ;
#20686=DIRECTION ( 'NONE',  ( -0.3886714912512299613, -0.2243995901002340809, -0.8936326403234116089 ) ) ;
#20687=CARTESIAN_POINT ( 'NONE',  ( 202.0496559082686474, 12.07111943211142169, -2.341985411376943826 ) ) ;
#20689=AXIS2_PLACEMENT_3D ( 'NONE', #4920, #3138, #683 ) ;
#20691=DIRECTION ( 'NONE',  ( -0.5566703992264087075, -0.3213938048432681271, 0.7660444431189863401 ) ) ;
#20693=DIRECTION ( 'NONE',  ( -0.6634139481689351747, -0.3830222215594923374, 0.6427876096865405842 ) ) ;
#20697=CARTESIAN_POINT ( 'NONE',  ( 205.2286857969292839, 9.782535276688832937, -15.28568448904319510 ) ) ;
#20699=PLANE ( 'NONE',  #3042 ) ;
#20703=ADVANCED_FACE ( 'NONE', ( #7864 ), #20477, .F. ) ;
#20706=CARTESIAN_POINT ( 'NONE',  ( 205.0662616026534693, 10.91332106064940888, -14.00000000000005507 ) ) ;
#20710=VECTOR ( 'NONE', #10600, 1000.000000000000227 ) ;
#20714=ORIENTED_EDGE ( 'NONE', *, *, #17264, .F. ) ;
#20717=( LENGTH_UNIT ( ) NAMED_UNIT ( * ) SI_UNIT ( .MILLI., .METRE. ) );
#20719=CARTESIAN_POINT ( 'NONE',  ( 199.4574108924007305, -0.1996992187545574282, -7.132002368301175288 ) ) ;
#20720=CARTESIAN_POINT ( 'NONE',  ( 208.4761278624580711, 5.007259451653140125, -14.00000000000005507 ) ) ;
#20723=ORIENTED_EDGE ( 'NONE', *, *, #2261, .F. ) ;
#20726=CIRCLE ( 'NONE', #4484, 11.94520687646042667 ) ;
#20728=EDGE_CURVE ( 'NONE', #1051, #15696, #13381, .T. ) ;
#20730=DIRECTION ( 'NONE',  ( -0.8528685319524385022, -0.4924038765061083955, 0.1736481776669413224 ) ) ;
#20731=DIRECTION ( 'NONE',  ( 0.8660254037844355990, 0.5000000000000054401, 0.000000000000000000 ) ) ;
#20735=CARTESIAN_POINT ( 'NONE',  ( 201.5316478576734198, 7.294022845898723517, -25.30691987834790524 ) ) ;
#20742=ORIENTED_EDGE ( 'NONE', *, *, #13487, .T. ) ;
#20747=ORIENTED_EDGE ( 'NONE', *, *, #14356, .F. ) ;
#20749=ORIENTED_EDGE ( 'NONE', *, *, #4022, .T. ) ;
#20752=LINE ( 'NONE', #9398, #15955 ) ;
#20755=VECTOR ( 'NONE', #418, 1000.000000000000114 ) ;
#20756=ORIENTED_EDGE ( 'NONE', *, *, #19895, .T. ) ;
#20760=EDGE_CURVE ( 'NONE', #7899, #1475, #12191, .T. ) ;
#20766=ORIENTED_EDGE ( 'NONE', *, *, #19628, .T. ) ;
#20768=DIRECTION ( 'NONE',  ( 0.000000000000000000, -0.000000000000000000, -1.000000000000000000 ) ) ;
#20774=ORIENTED_EDGE ( 'NONE', *, *, #3043, .T. ) ;
#20776=LINE ( 'NONE', #17295, #4600 ) ;
#20778=DIRECTION ( 'NONE',  ( -0.5000000000000051070, 0.8660254037844359321, -0.000000000000000000 ) ) ;
#20779=EDGE_CURVE ( 'NONE', #15885, #11656, #19551, .T. ) ;
#20788=CARTESIAN_POINT ( 'NONE',  ( 193.8244552494320772, 17.93697134796469328, -3.188775577416750995 ) ) ;
#20789=DIRECTION ( 'NONE',  ( 0.7951984747223578287, 0.4591080534401396629, -0.3960797660391672803 ) ) ;
#20790=CARTESIAN_POINT ( 'NONE',  ( 202.7150726112346319, 7.800250765496993033, -25.94618751764486575 ) ) ;
#20794=EDGE_CURVE ( 'NONE', #9080, #688, #4020, .T. ) ;
#20798=ORIENTED_EDGE ( 'NONE', *, *, #7718, .T. ) ;
#20800=CARTESIAN_POINT ( 'NONE',  ( 209.4254563108873413, 4.782534396259779719, -0.8632678296711639998 ) ) ;
#20808=FACE_OUTER_BOUND ( 'NONE', #18895, .T. ) ;
#20811=DIRECTION ( 'NONE',  ( -0.8660254037843260200, -0.5000000000001951772, 0.000000000000000000 ) ) ;
#20812=CARTESIAN_POINT ( 'NONE',  ( 219.0593366061551137, 10.34465777807333531, -13.97827067520052147 ) ) ;
#20813=APPLICATION_CONTEXT ( 'automotive_design' ) ;
#20816=EDGE_LOOP ( 'NONE', ( #17370, #7475, #10381, #19808, #10006, #10436 ) ) ;
#20818=DIRECTION ( 'NONE',  ( -0.5000000000000049960, 0.8660254037844357100, -0.000000000000000000 ) ) ;
#20819=EDGE_CURVE ( 'NONE', #10374, #10151, #18869, .T. ) ;
#20823=FACE_OUTER_BOUND ( 'NONE', #13005, .T. ) ;
#20825=DIRECTION ( 'NONE',  ( 0.5016613886297335290, 0.000000000000000000, 0.8650640734408565624 ) ) ;
#20827=VERTEX_POINT ( 'NONE', #2339 ) ;
#20829=DIRECTION ( 'NONE',  ( 0.5000000000000052180, -0.8660254037844355990, 2.220446049250312588E-16 ) ) ;
#20831=CARTESIAN_POINT ( 'NONE',  ( 206.5868379288083645, 3.916477399883220745, -1.717498466822807490 ) ) ;
#20836=VERTEX_POINT ( 'NONE', #7398 ) ;
#20838=ORIENTED_EDGE ( 'NONE', *, *, #20521, .F. ) ;
#20840=DIRECTION ( 'NONE',  ( -0.9885408208161367005, 0.000000000000000000, 0.1509537862398905028 ) ) ;
#20843=VERTEX_POINT ( 'NONE', #17274 ) ;
#20846=CARTESIAN_POINT ( 'NONE',  ( 195.0945143319839872, 3.400519391596340757, -15.43274561385865695 ) ) ;
#20848=VECTOR ( 'NONE', #10207, 1000.000000000000114 ) ;
#20851=ORIENTED_EDGE ( 'NONE', *, *, #14736, .F. ) ;
#20853=DIRECTION ( 'NONE',  ( 0.5000000000000052180, -0.8660254037844355990, -1.665334536937734318E-16 ) ) ;
#20854=VECTOR ( 'NONE', #17993, 1000.000000000000114 ) ;
#20855=DIRECTION ( 'NONE',  ( 0.5000000000000049960, -0.8660254037844358210, 0.000000000000000000 ) ) ;
#20856=CARTESIAN_POINT ( 'NONE',  ( 210.7957517463719057, 12.99668230119596934, -3.627429155984617459 ) ) ;
#20861=ORIENTED_EDGE ( 'NONE', *, *, #2537, .F. ) ;
#20865=CIRCLE ( 'NONE', #15825, 3.845804376225747667 ) ;
#20868=ORIENTED_EDGE ( 'NONE', *, *, #10687, .F. ) ;
#20871=EDGE_CURVE ( 'NONE', #3434, #437, #8897, .T. ) ;
#20879=CARTESIAN_POINT ( 'NONE',  ( 213.9717500725588479, 7.407338323375970646, -24.35247136794745515 ) ) ;
#20880=CYLINDRICAL_SURFACE ( 'NONE', #15440, 12.47473710546057646 ) ;
#20887=CARTESIAN_POINT ( 'NONE',  ( 208.0983737146324870, 5.661548828456886895, -14.00000000000005507 ) ) ;
#20892=EDGE_CURVE ( 'NONE', #18441, #18887, #20571, .T. ) ;
#20896=VECTOR ( 'NONE', #14647, 1000.000000000000114 ) ;
#20897=ORIENTED_EDGE ( 'NONE', *, *, #13268, .T. ) ;
#20898=VERTEX_POINT ( 'NONE', #1171 ) ;
#20900=ORIENTED_EDGE ( 'NONE', *, *, #20892, .F. ) ;
#20904=CARTESIAN_POINT ( 'NONE',  ( 213.2794616557154939, 7.007645419554564548, -26.10173121575784450 ) ) ;
#20906=CARTESIAN_POINT ( 'NONE',  ( 190.1957632562343008, 15.84194504888569988, -7.132002368301173512 ) ) ;
#20908=EDGE_CURVE ( 'NONE', #12371, #12475, #16187, .T. ) ;
#20914=CARTESIAN_POINT ( 'NONE',  ( 218.8798129321970976, 10.24100973658777924, -16.73990883341947367 ) ) ;
#20915=CARTESIAN_POINT ( 'NONE',  ( 209.7298162261493815, 27.11993578943074823, -11.13829696442610029 ) ) ;
#20917=ORIENTED_EDGE ( 'NONE', *, *, #10676, .F. ) ;
#20924=EDGE_CURVE ( 'NONE', #14504, #18516, #15595, .T. ) ;
#20928=B_SPLINE_CURVE_WITH_KNOTS ( 'NONE', 3,
 ( #9557, #7547, #16054, #14041 ),
 .UNSPECIFIED., .F., .F.,
 ( 4, 4 ),
 ( 3.079010676197774585E-05, 0.0008847758447462670487 ),
 .UNSPECIFIED. ) ;
#20929=VERTEX_POINT ( 'NONE', #2863 ) ;
#20931=EDGE_CURVE ( 'NONE', #11210, #15101, #3065, .T. ) ;
#20932=AXIS2_PLACEMENT_3D ( 'NONE', #15932, #3096, #1606 ) ;
#20937=EDGE_CURVE ( 'NONE', #8299, #18096, #11615, .T. ) ;
#20939=CARTESIAN_POINT ( 'NONE',  ( 213.4352746215837726, 14.52061154373172158, -6.376588578941996488 ) ) ;
#20944=ORIENTED_EDGE ( 'NONE', *, *, #4420, .T. ) ;
#20945=CARTESIAN_POINT ( 'NONE',  ( 199.4613974551745059, 6.452789800082466165, -23.47937149798923429 ) ) ;
#20946=CARTESIAN_POINT ( 'NONE',  ( 198.2729934012025979, -1.398743842967087314, -15.41218500610144559 ) ) ;
#20947=CARTESIAN_POINT ( 'NONE',  ( 201.8794782033450588, 11.97286728836375680, -26.96550585544242296 ) ) ;
#20982=COLOUR_RGB('Grey',0.48,0.52,0.57);
#20983=FILL_AREA_STYLE_COLOUR('',#20982);
#20984=FILL_AREA_STYLE('',(#20983));
#20985=SURFACE_STYLE_FILL_AREA(#20984);
#20986=SURFACE_SIDE_STYLE('',(#20985));
#20987=SURFACE_STYLE_USAGE(.BOTH.,#20986);
#20988=PRESENTATION_STYLE_ASSIGNMENT((#20987));
ENDSEC;
END-ISO-10303-21;
